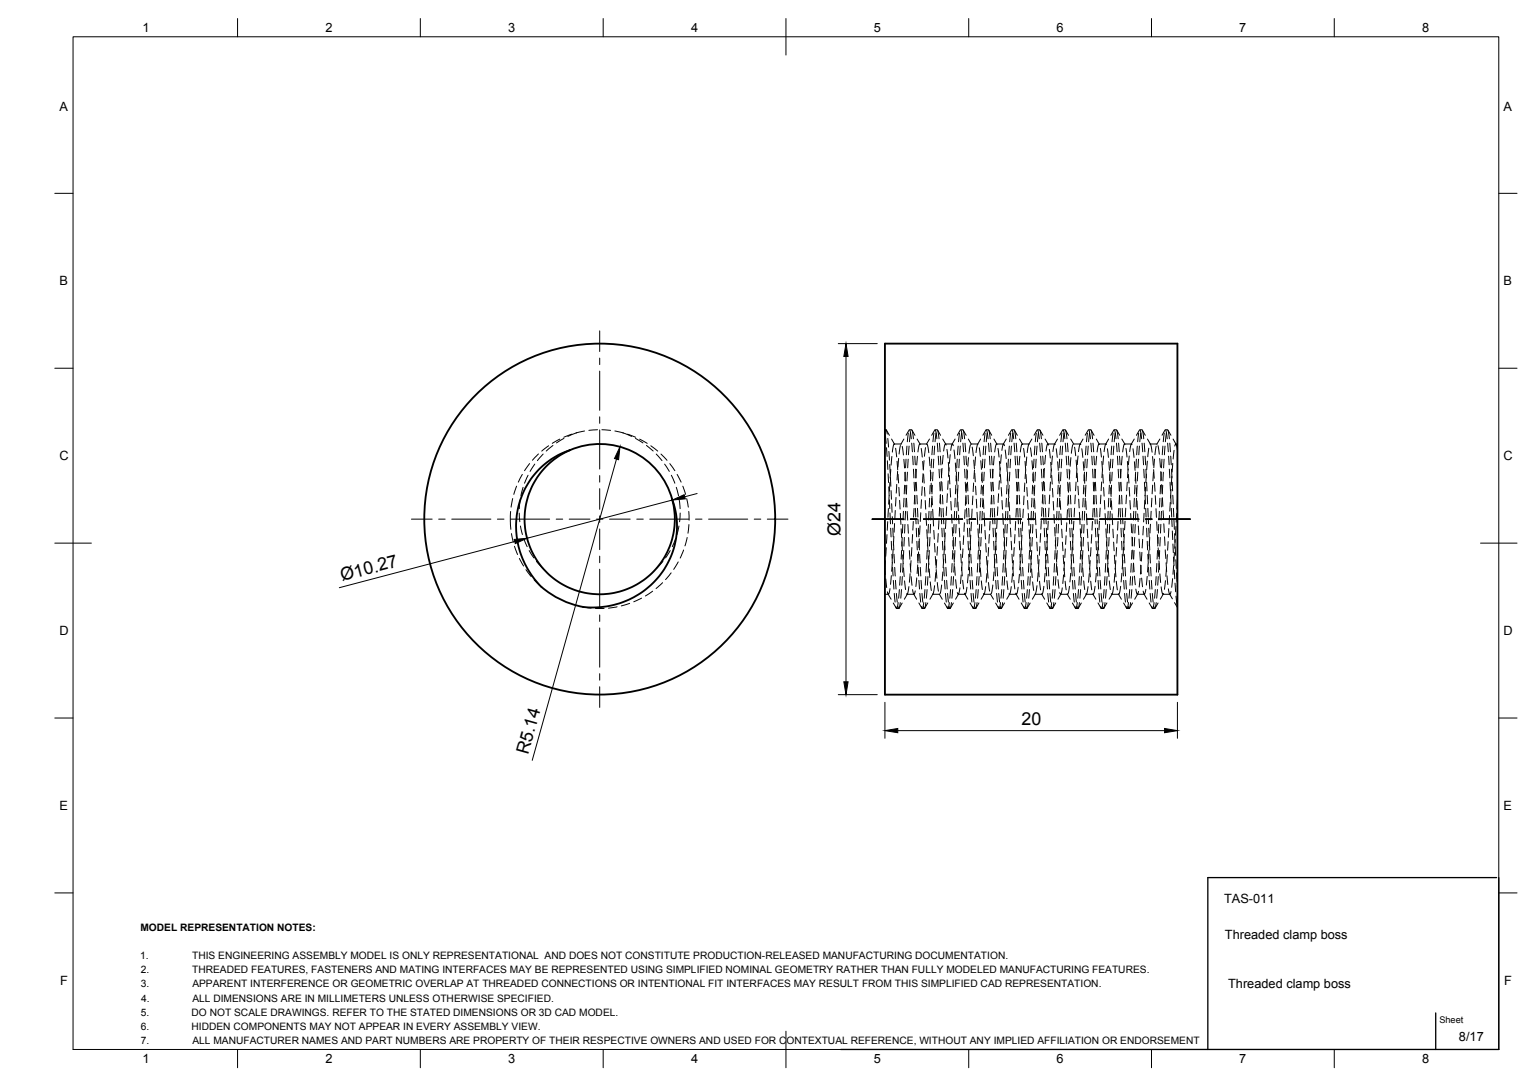
ISO-10303-21;
HEADER;
/* Generated by software containing ST-Developer
 * from STEP Tools, Inc. (www.steptools.com) 
 */

FILE_DESCRIPTION(
/* description */ (
'Independent manual bench leaf bending machine,200mm work width. Fabri
cated welded frame and folding leaf, repeated bushed and fully retaine
d hinge hardware, two handles with bonded grips, beveled clamping beam
 and modeledM12 clamp screws.2mm omitted-workpiece assembly reference 
gap, not a capacity claim. Native135deg hinge travel. Weld sizing, pro
duction fits, material condition, bending capacity, strength and life 
unassigned.'),
/* implementation_level */ '2;1');

FILE_NAME(
/* name */ 'Threaded clamp boss.step',
/* time_stamp */ '2026-11-14T09:11:34-08:00',
/* author */ (''),
/* organization */ (''),
/* preprocessor_version */ 'ST-DEVELOPER v20.2',
/* originating_system */ 'Autodesk Translation Framework v15.17.0.0',
/* authorisation */ '');

FILE_SCHEMA (('AUTOMOTIVE_DESIGN { 1 0 10303 214 3 1 1 }'));
ENDSEC;

DATA;
#10=MECHANICAL_DESIGN_GEOMETRIC_PRESENTATION_REPRESENTATION('',(#452),#37701);
#148=B_SPLINE_SURFACE_WITH_KNOTS('',3,3,((#12501,#12502,#12503,#12504,#12505,
#12506,#12507,#12508,#12509,#12510,#12511,#12512,#12513,#12514,#12515,#12516,
#12517,#12518,#12519,#12520,#12521,#12522,#12523,#12524,#12525,#12526,#12527,
#12528,#12529,#12530,#12531,#12532,#12533,#12534,#12535,#12536,#12537,#12538,
#12539,#12540,#12541,#12542,#12543,#12544,#12545,#12546,#12547,#12548,#12549,
#12550,#12551,#12552,#12553,#12554,#12555,#12556,#12557,#12558,#12559,#12560,
#12561,#12562,#12563,#12564,#12565,#12566,#12567,#12568,#12569,#12570,#12571,
#12572,#12573,#12574,#12575,#12576,#12577,#12578,#12579,#12580,#12581,#12582,
#12583,#12584,#12585,#12586,#12587,#12588,#12589,#12590,#12591,#12592,#12593,
#12594,#12595,#12596,#12597,#12598,#12599,#12600,#12601,#12602,#12603,#12604,
#12605,#12606,#12607,#12608,#12609,#12610,#12611,#12612,#12613,#12614,#12615,
#12616,#12617,#12618,#12619,#12620,#12621,#12622,#12623,#12624,#12625,#12626,
#12627,#12628,#12629,#12630,#12631,#12632,#12633,#12634,#12635,#12636,#12637,
#12638,#12639,#12640,#12641,#12642,#12643,#12644,#12645,#12646,#12647,#12648,
#12649,#12650,#12651),(#12652,#12653,#12654,#12655,#12656,#12657,#12658,
#12659,#12660,#12661,#12662,#12663,#12664,#12665,#12666,#12667,#12668,#12669,
#12670,#12671,#12672,#12673,#12674,#12675,#12676,#12677,#12678,#12679,#12680,
#12681,#12682,#12683,#12684,#12685,#12686,#12687,#12688,#12689,#12690,#12691,
#12692,#12693,#12694,#12695,#12696,#12697,#12698,#12699,#12700,#12701,#12702,
#12703,#12704,#12705,#12706,#12707,#12708,#12709,#12710,#12711,#12712,#12713,
#12714,#12715,#12716,#12717,#12718,#12719,#12720,#12721,#12722,#12723,#12724,
#12725,#12726,#12727,#12728,#12729,#12730,#12731,#12732,#12733,#12734,#12735,
#12736,#12737,#12738,#12739,#12740,#12741,#12742,#12743,#12744,#12745,#12746,
#12747,#12748,#12749,#12750,#12751,#12752,#12753,#12754,#12755,#12756,#12757,
#12758,#12759,#12760,#12761,#12762,#12763,#12764,#12765,#12766,#12767,#12768,
#12769,#12770,#12771,#12772,#12773,#12774,#12775,#12776,#12777,#12778,#12779,
#12780,#12781,#12782,#12783,#12784,#12785,#12786,#12787,#12788,#12789,#12790,
#12791,#12792,#12793,#12794,#12795,#12796,#12797,#12798,#12799,#12800,#12801,
#12802),(#12803,#12804,#12805,#12806,#12807,#12808,#12809,#12810,#12811,
#12812,#12813,#12814,#12815,#12816,#12817,#12818,#12819,#12820,#12821,#12822,
#12823,#12824,#12825,#12826,#12827,#12828,#12829,#12830,#12831,#12832,#12833,
#12834,#12835,#12836,#12837,#12838,#12839,#12840,#12841,#12842,#12843,#12844,
#12845,#12846,#12847,#12848,#12849,#12850,#12851,#12852,#12853,#12854,#12855,
#12856,#12857,#12858,#12859,#12860,#12861,#12862,#12863,#12864,#12865,#12866,
#12867,#12868,#12869,#12870,#12871,#12872,#12873,#12874,#12875,#12876,#12877,
#12878,#12879,#12880,#12881,#12882,#12883,#12884,#12885,#12886,#12887,#12888,
#12889,#12890,#12891,#12892,#12893,#12894,#12895,#12896,#12897,#12898,#12899,
#12900,#12901,#12902,#12903,#12904,#12905,#12906,#12907,#12908,#12909,#12910,
#12911,#12912,#12913,#12914,#12915,#12916,#12917,#12918,#12919,#12920,#12921,
#12922,#12923,#12924,#12925,#12926,#12927,#12928,#12929,#12930,#12931,#12932,
#12933,#12934,#12935,#12936,#12937,#12938,#12939,#12940,#12941,#12942,#12943,
#12944,#12945,#12946,#12947,#12948,#12949,#12950,#12951,#12952,#12953),
(#12954,#12955,#12956,#12957,#12958,#12959,#12960,#12961,#12962,#12963,
#12964,#12965,#12966,#12967,#12968,#12969,#12970,#12971,#12972,#12973,#12974,
#12975,#12976,#12977,#12978,#12979,#12980,#12981,#12982,#12983,#12984,#12985,
#12986,#12987,#12988,#12989,#12990,#12991,#12992,#12993,#12994,#12995,#12996,
#12997,#12998,#12999,#13000,#13001,#13002,#13003,#13004,#13005,#13006,#13007,
#13008,#13009,#13010,#13011,#13012,#13013,#13014,#13015,#13016,#13017,#13018,
#13019,#13020,#13021,#13022,#13023,#13024,#13025,#13026,#13027,#13028,#13029,
#13030,#13031,#13032,#13033,#13034,#13035,#13036,#13037,#13038,#13039,#13040,
#13041,#13042,#13043,#13044,#13045,#13046,#13047,#13048,#13049,#13050,#13051,
#13052,#13053,#13054,#13055,#13056,#13057,#13058,#13059,#13060,#13061,#13062,
#13063,#13064,#13065,#13066,#13067,#13068,#13069,#13070,#13071,#13072,#13073,
#13074,#13075,#13076,#13077,#13078,#13079,#13080,#13081,#13082,#13083,#13084,
#13085,#13086,#13087,#13088,#13089,#13090,#13091,#13092,#13093,#13094,#13095,
#13096,#13097,#13098,#13099,#13100,#13101,#13102,#13103,#13104)),
 .UNSPECIFIED.,.F.,.F.,.F.,(4,4),(4,1,1,1,1,1,1,1,1,1,1,1,1,1,1,1,1,1,1,
1,1,1,1,1,1,1,1,1,1,1,1,1,1,1,1,1,1,1,1,1,1,1,1,1,1,1,1,1,1,1,1,1,1,1,1,
1,1,1,1,1,1,1,1,1,1,1,1,1,1,1,1,1,1,1,1,1,1,1,1,1,1,1,1,1,1,1,1,1,1,1,1,
1,1,1,1,1,1,1,1,1,1,1,1,1,1,1,1,1,1,1,1,1,1,1,1,1,1,1,1,1,1,1,1,1,1,1,1,
1,1,1,1,1,1,1,1,1,1,1,1,1,1,1,1,1,1,1,1,1,4),(-6.2431789936198E-5,0.112802168308183),
(11.8516712330609,12.3505987470977,12.8494638293446,13.3483289115915,13.8471939938383,
14.3460590760852,14.8449241583321,15.343789240579,15.8426543228258,16.3415194050727,
16.8403844873196,17.3392495695665,17.8381146518133,18.3369797340602,18.8358448163071,
19.334709898554,19.8335749808009,20.3324400630477,20.8313051452946,21.3301702275415,
21.8290353097884,22.3279003920352,22.8267654742821,23.325630556529,23.8244956387759,
24.3233607210227,24.8222258032696,25.3210908855165,25.8199559677634,26.3188210500103,
26.8176861322571,27.316551214504,27.8154162967509,28.3142813789978,28.8131464612446,
29.3120115434915,29.8108766257384,30.3097417079853,30.8086067902321,31.307471872479,
31.8063369547259,32.3052020369728,32.8040671192197,33.3029322014665,33.8017972837134,
34.3006623659603,34.7995274482072,35.298392530454,35.7972576127009,36.2961226949478,
36.7949877771947,37.2938528594415,37.7927179416884,38.2915830239353,38.7904481061822,
39.2893131884291,39.7881782706759,40.2870433529228,40.7859084351697,41.2847735174166,
41.7836385996634,42.2825036819103,42.7813687641572,43.2802338464041,43.779098928651,
44.2779640108978,44.7768290931447,45.2756941753916,45.7745592576385,46.2734243398853,
46.7722894221322,47.2711545043791,47.770019586626,48.2688846688728,48.7677497511197,
49.2666148333666,49.7654799156135,50.2643449978603,50.7632100801072,51.2620751623541,
51.760940244601,52.2598053268479,52.7586704090947,53.2575354913416,53.7564005735885,
54.2552656558354,54.7541307380822,55.2529958203291,55.751860902576,56.2507259848229,
56.7495910670697,57.2484561493166,57.7473212315635,58.2461863138104,58.7450513960573,
59.2439164783041,59.742781560551,60.2416466427979,60.7405117250448,61.2393768072916,
61.7382418895385,62.2371069717854,62.7359720540323,63.2348371362792,63.733702218526,
64.2325673007729,64.7314323830198,65.2302974652667,65.7291625475135,66.2280276297604,
66.7268927120073,67.2257577942542,67.724622876501,68.2234879587479,68.7223530409948,
69.2212181232417,69.7200832054885,70.2189482877354,70.7178133699823,71.2166784522292,
71.7155435344761,72.2144086167229,72.7132736989698,73.2121387812167,73.7110038634636,
74.2098689457104,74.7087340279573,75.2075991102042,75.7064641924511,76.205329274698,
76.7041943569448,77.2030594391917,77.7019245214386,78.2007896036855,78.6996546859323,
79.1985197681792,79.6973848504261,80.196249932673,80.6951150149198,81.1939800971667,
81.6928451794136,82.1917102616605,82.6905753439074,83.1894404261542,83.6883055084011,
84.187170590648,84.6860356728949,85.1849007551417,85.6837658373886),
 .UNSPECIFIED.);
#149=B_SPLINE_SURFACE_WITH_KNOTS('',3,3,((#13322,#13323,#13324,#13325,#13326,
#13327,#13328,#13329,#13330,#13331,#13332,#13333,#13334,#13335,#13336,#13337,
#13338,#13339,#13340,#13341,#13342,#13343,#13344,#13345,#13346,#13347,#13348,
#13349,#13350,#13351,#13352,#13353,#13354,#13355,#13356,#13357,#13358,#13359,
#13360,#13361,#13362,#13363,#13364,#13365,#13366,#13367,#13368,#13369,#13370,
#13371,#13372,#13373,#13374,#13375,#13376,#13377,#13378,#13379,#13380,#13381,
#13382,#13383,#13384,#13385,#13386,#13387,#13388,#13389,#13390,#13391,#13392,
#13393,#13394,#13395,#13396,#13397,#13398,#13399,#13400,#13401,#13402,#13403,
#13404,#13405,#13406,#13407,#13408,#13409,#13410,#13411,#13412,#13413,#13414,
#13415,#13416,#13417,#13418,#13419,#13420,#13421,#13422,#13423,#13424,#13425,
#13426,#13427,#13428,#13429,#13430,#13431,#13432,#13433,#13434,#13435,#13436,
#13437,#13438,#13439,#13440,#13441,#13442,#13443,#13444,#13445,#13446,#13447,
#13448,#13449,#13450,#13451,#13452,#13453,#13454,#13455,#13456,#13457,#13458,
#13459,#13460,#13461,#13462,#13463,#13464,#13465,#13466,#13467,#13468,#13469,
#13470,#13471,#13472),(#13473,#13474,#13475,#13476,#13477,#13478,#13479,
#13480,#13481,#13482,#13483,#13484,#13485,#13486,#13487,#13488,#13489,#13490,
#13491,#13492,#13493,#13494,#13495,#13496,#13497,#13498,#13499,#13500,#13501,
#13502,#13503,#13504,#13505,#13506,#13507,#13508,#13509,#13510,#13511,#13512,
#13513,#13514,#13515,#13516,#13517,#13518,#13519,#13520,#13521,#13522,#13523,
#13524,#13525,#13526,#13527,#13528,#13529,#13530,#13531,#13532,#13533,#13534,
#13535,#13536,#13537,#13538,#13539,#13540,#13541,#13542,#13543,#13544,#13545,
#13546,#13547,#13548,#13549,#13550,#13551,#13552,#13553,#13554,#13555,#13556,
#13557,#13558,#13559,#13560,#13561,#13562,#13563,#13564,#13565,#13566,#13567,
#13568,#13569,#13570,#13571,#13572,#13573,#13574,#13575,#13576,#13577,#13578,
#13579,#13580,#13581,#13582,#13583,#13584,#13585,#13586,#13587,#13588,#13589,
#13590,#13591,#13592,#13593,#13594,#13595,#13596,#13597,#13598,#13599,#13600,
#13601,#13602,#13603,#13604,#13605,#13606,#13607,#13608,#13609,#13610,#13611,
#13612,#13613,#13614,#13615,#13616,#13617,#13618,#13619,#13620,#13621,#13622,
#13623),(#13624,#13625,#13626,#13627,#13628,#13629,#13630,#13631,#13632,
#13633,#13634,#13635,#13636,#13637,#13638,#13639,#13640,#13641,#13642,#13643,
#13644,#13645,#13646,#13647,#13648,#13649,#13650,#13651,#13652,#13653,#13654,
#13655,#13656,#13657,#13658,#13659,#13660,#13661,#13662,#13663,#13664,#13665,
#13666,#13667,#13668,#13669,#13670,#13671,#13672,#13673,#13674,#13675,#13676,
#13677,#13678,#13679,#13680,#13681,#13682,#13683,#13684,#13685,#13686,#13687,
#13688,#13689,#13690,#13691,#13692,#13693,#13694,#13695,#13696,#13697,#13698,
#13699,#13700,#13701,#13702,#13703,#13704,#13705,#13706,#13707,#13708,#13709,
#13710,#13711,#13712,#13713,#13714,#13715,#13716,#13717,#13718,#13719,#13720,
#13721,#13722,#13723,#13724,#13725,#13726,#13727,#13728,#13729,#13730,#13731,
#13732,#13733,#13734,#13735,#13736,#13737,#13738,#13739,#13740,#13741,#13742,
#13743,#13744,#13745,#13746,#13747,#13748,#13749,#13750,#13751,#13752,#13753,
#13754,#13755,#13756,#13757,#13758,#13759,#13760,#13761,#13762,#13763,#13764,
#13765,#13766,#13767,#13768,#13769,#13770,#13771,#13772,#13773,#13774),
(#13775,#13776,#13777,#13778,#13779,#13780,#13781,#13782,#13783,#13784,
#13785,#13786,#13787,#13788,#13789,#13790,#13791,#13792,#13793,#13794,#13795,
#13796,#13797,#13798,#13799,#13800,#13801,#13802,#13803,#13804,#13805,#13806,
#13807,#13808,#13809,#13810,#13811,#13812,#13813,#13814,#13815,#13816,#13817,
#13818,#13819,#13820,#13821,#13822,#13823,#13824,#13825,#13826,#13827,#13828,
#13829,#13830,#13831,#13832,#13833,#13834,#13835,#13836,#13837,#13838,#13839,
#13840,#13841,#13842,#13843,#13844,#13845,#13846,#13847,#13848,#13849,#13850,
#13851,#13852,#13853,#13854,#13855,#13856,#13857,#13858,#13859,#13860,#13861,
#13862,#13863,#13864,#13865,#13866,#13867,#13868,#13869,#13870,#13871,#13872,
#13873,#13874,#13875,#13876,#13877,#13878,#13879,#13880,#13881,#13882,#13883,
#13884,#13885,#13886,#13887,#13888,#13889,#13890,#13891,#13892,#13893,#13894,
#13895,#13896,#13897,#13898,#13899,#13900,#13901,#13902,#13903,#13904,#13905,
#13906,#13907,#13908,#13909,#13910,#13911,#13912,#13913,#13914,#13915,#13916,
#13917,#13918,#13919,#13920,#13921,#13922,#13923,#13924,#13925)),
 .UNSPECIFIED.,.F.,.F.,.F.,(4,4),(4,1,1,1,1,1,1,1,1,1,1,1,1,1,1,1,1,1,1,
1,1,1,1,1,1,1,1,1,1,1,1,1,1,1,1,1,1,1,1,1,1,1,1,1,1,1,1,1,1,1,1,1,1,1,1,
1,1,1,1,1,1,1,1,1,1,1,1,1,1,1,1,1,1,1,1,1,1,1,1,1,1,1,1,1,1,1,1,1,1,1,1,
1,1,1,1,1,1,1,1,1,1,1,1,1,1,1,1,1,1,1,1,1,1,1,1,1,1,1,1,1,1,1,1,1,1,1,1,
1,1,1,1,1,1,1,1,1,1,1,1,1,1,1,1,1,1,1,1,1,4),(-4.55374339698837E-5,0.1128189478572),
(14.3984001269718,14.8972652092187,15.3961302914656,15.8949953737124,16.3938604559593,
16.8927255382062,17.3915906204531,17.8904557026999,18.3893207849468,18.8881858671937,
19.3870509494406,19.8859160316874,20.3847811139343,20.8836461961812,21.3825112784281,
21.881376360675,22.3802414429218,22.8791065251687,23.3779716074156,23.8768366896625,
24.3757017719093,24.8745668541562,25.3734319364031,25.87229701865,26.3711621008968,
26.8700271831437,27.3688922653906,27.8677573476375,28.3666224298844,28.8654875121312,
29.3643525943781,29.863217676625,30.3620827588719,30.8609478411187,31.3598129233656,
31.8586780056125,32.3575430878594,32.8564081701062,33.3552732523531,33.8541383346,
34.3530034168469,34.8518684990938,35.3507335813406,35.8495986635875,36.3484637458344,
36.8473288280813,37.3461939103281,37.845058992575,38.3439240748219,38.8427891570688,
39.3416542393157,39.8405193215625,40.3393844038094,40.8382494860563,41.3371145683032,
41.83597965055,42.3348447327969,42.8337098150438,43.3325748972907,43.8314399795375,
44.3303050617844,44.8291701440313,45.3280352262782,45.8269003085251,46.3257653907719,
46.8246304730188,47.3234955552657,47.8223606375126,48.3212257197594,48.8200908020063,
49.3189558842532,49.8178209665001,50.316686048747,50.8155511309938,51.3144162132407,
51.8132812954876,52.3121463777345,52.8110114599813,53.3098765422282,53.8087416244751,
54.307606706722,54.8064717889688,55.3053368712157,55.8042019534626,56.3030670357095,
56.8019321179564,57.3007972002032,57.7996622824501,58.298527364697,58.7973924469439,
59.2962575291907,59.7951226114376,60.2939876936845,60.7928527759314,61.2917178581782,
61.7905829404251,62.289448022672,62.7883131049189,63.2871781871658,63.7860432694126,
64.2849083516595,64.7837734339064,65.2826385161533,65.7815035984001,66.280368680647,
66.7792337628939,67.2780988451408,67.7769639273876,68.2758290096345,68.7746940918814,
69.2735591741283,69.7724242563752,70.271289338622,70.7701544208689,71.2690195031158,
71.7678845853627,72.2667496676095,72.7656147498564,73.2644798321033,73.7633449143502,
74.2622099965971,74.7610750788439,75.2599401610908,75.7588052433377,76.2576703255846,
76.7565354078314,77.2554004900783,77.7542655723252,78.2531306545721,78.7519957368189,
79.2508608190658,79.7497259013127,80.2485909835596,80.7474560658064,81.2463211480533,
81.7451862303002,82.2440513125471,82.742916394794,83.2417814770408,83.7406465592877,
84.2395116415346,84.7383767237815,85.2372418060283,85.7361068882752,86.2349719705221,
86.733837052769,87.2327021350158,87.7315672172627,88.2304947397941),
 .UNSPECIFIED.);
#152=B_SPLINE_CURVE_WITH_KNOTS('',3,(#5917,#5918,#5919,#5920,#5921,#5922,
#5923,#5924,#5925,#5926,#5927,#5928),.UNSPECIFIED.,.F.,.F.,(4,1,1,1,1,1,
1,1,1,4),(80.7654236598523,81.1939800971667,81.6928451794136,82.1917102616605,
82.6905753439074,83.1894404261542,83.6883055084011,84.187170590648,84.6860356728949,
84.8230016469244),.UNSPECIFIED.);
#153=B_SPLINE_CURVE_WITH_KNOTS('',3,(#5930,#5931,#5932,#5933,#5934),
 .UNSPECIFIED.,.F.,.F.,(4,1,4),(84.8230016469244,85.1849007551417,85.6837658373886),
 .UNSPECIFIED.);
#154=B_SPLINE_CURVE_WITH_KNOTS('',3,(#5938,#5939,#5940,#5941,#5942,#5943,
#5944,#5945,#5946,#5947,#5948,#5949,#5950,#5951,#5952,#5953,#5954,#5955,
#5956,#5957,#5958,#5959,#5960,#5961,#5962,#5963,#5964,#5965,#5966,#5967,
#5968,#5969,#5970,#5971,#5972,#5973,#5974,#5975,#5976,#5977,#5978,#5979,
#5980,#5981,#5982,#5983,#5984,#5985,#5986,#5987,#5988,#5989),
 .UNSPECIFIED.,.F.,.F.,(4,3,3,3,3,3,3,3,3,3,3,3,3,3,3,3,3,4),(84.8230016469244,
84.9058580301686,84.9887137387844,85.0715624591206,85.1544337152411,85.2372418060283,
85.3204458619835,85.4036336567022,85.4868246260799,85.5700099876162,85.6532174303604,
85.7361068882752,85.8191359181166,85.9021481942019,85.9851620989545,86.0681715464416,
86.151200160365,86.2062322090242),.UNSPECIFIED.);
#155=B_SPLINE_CURVE_WITH_KNOTS('',3,(#5990,#5991,#5992,#5993,#5994,#5995,
#5996,#5997,#5998,#5999,#6000,#6001),.UNSPECIFIED.,.F.,.F.,(4,1,1,1,1,1,
1,1,1,4),(80.7654089732259,81.2463211480533,81.7451862303002,82.2440513125471,
82.742916394794,83.2417814770408,83.7406465592877,84.2395116415346,84.7383767237815,
84.8230016469244),.UNSPECIFIED.);
#156=B_SPLINE_CURVE_WITH_KNOTS('',3,(#6007,#6008,#6009,#6010,#6011,#6012,
#6013,#6014,#6015,#6016,#6017,#6018,#6019,#6020,#6021,#6022,#6023,#6024,
#6025,#6026,#6027,#6028,#6029,#6030,#6031,#6032,#6033,#6034,#6035,#6036,
#6037,#6038,#6039,#6040,#6041,#6042,#6043,#6044,#6045,#6046,#6047,#6048,
#6049,#6050,#6051,#6052,#6053,#6054,#6055,#6056,#6057,#6058,#6059,#6060,
#6061,#6062,#6063,#6064,#6065,#6066,#6067,#6068,#6069,#6070,#6071,#6072,
#6073,#6074,#6075,#6076,#6077,#6078,#6079,#6080,#6081,#6082,#6083,#6084,
#6085,#6086,#6087,#6088,#6089,#6090,#6091,#6092,#6093,#6094,#6095,#6096,
#6097,#6098,#6099,#6100,#6101,#6102,#6103,#6104,#6105,#6106,#6107,#6108,
#6109,#6110,#6111,#6112,#6113,#6114,#6115,#6116,#6117,#6118,#6119,#6120,
#6121,#6122,#6123,#6124,#6125,#6126,#6127,#6128,#6129,#6130,#6131,#6132,
#6133,#6134,#6135,#6136,#6137,#6138,#6139,#6140,#6141,#6142,#6143,#6144,
#6145,#6146,#6147,#6148,#6149,#6150,#6151,#6152,#6153,#6154),
 .UNSPECIFIED.,.F.,.F.,(4,3,3,3,3,3,3,3,3,3,3,3,3,3,3,3,3,3,3,3,3,3,3,3,
3,3,3,3,3,3,3,3,3,3,3,3,3,3,3,3,3,3,3,3,3,3,3,3,3,4),(74.4822133280158,
74.5653991646366,74.6486051631925,74.7087340279573,74.7919387913187,74.8751273240303,
74.9583190715775,75.0415052315879,75.1247134988495,75.2075991102042,75.2908038725438,
75.3739924042304,75.4571841507579,75.5403703097531,75.6235785760172,75.7064641924511,
75.789668956311,75.8728574895209,75.9560492375621,76.039235398063,76.1224436658041,
76.205329274698,76.2885340372514,76.3717225691568,76.454914315908,76.5381004751292,
76.6213087416209,76.7041943569448,76.7873991181458,76.8705876486823,76.9537793940503,
77.0369655518835,77.1201738169931,77.2030594391917,77.2862642100853,77.3694527503662,
77.452644505469,77.5358306730124,77.619038947697,77.7019245214386,77.7851292641372,
77.8683177761065,77.9515095029856,78.034695642409,78.1179038894172,78.2007896036855,
78.2855462877003,78.3686837869672,78.454250063356,78.5398163397448),
 .UNSPECIFIED.);
#157=B_SPLINE_CURVE_WITH_KNOTS('',3,(#6155,#6156,#6157,#6158,#6159,#6160,
#6161,#6162,#6163),.UNSPECIFIED.,.F.,.F.,(4,1,1,1,1,1,4),(78.5398163723456,
78.6996546859323,79.1985197681792,79.6973848504261,80.196249932673,80.6951150149198,
80.7654236598523),.UNSPECIFIED.);
#158=B_SPLINE_CURVE_WITH_KNOTS('',3,(#6165,#6166,#6167,#6168,#6169,#6170,
#6171,#6172,#6173),.UNSPECIFIED.,.F.,.F.,(4,1,1,1,1,1,4),(78.5398163397448,
78.7519957368189,79.2508608190658,79.7497259013127,80.2485909835596,80.7474560658064,
80.7654089732259),.UNSPECIFIED.);
#159=B_SPLINE_CURVE_WITH_KNOTS('',3,(#6174,#6175,#6176,#6177,#6178,#6179,
#6180,#6181,#6182,#6183,#6184,#6185),.UNSPECIFIED.,.F.,.F.,(4,1,1,1,1,1,
1,1,1,4),(74.4822262911247,74.7610750788439,75.2599401610908,75.7588052433377,
76.2576703255846,76.7565354078314,77.2554004900783,77.7542655723252,78.2531306545721,
78.5398163397448),.UNSPECIFIED.);
#160=B_SPLINE_CURVE_WITH_KNOTS('',3,(#6191,#6192,#6193,#6194,#6195,#6196,
#6197,#6198,#6199,#6200,#6201,#6202,#6203,#6204,#6205,#6206,#6207,#6208,
#6209,#6210,#6211,#6212,#6213,#6214,#6215,#6216,#6217,#6218,#6219,#6220,
#6221,#6222,#6223,#6224,#6225,#6226,#6227,#6228,#6229,#6230,#6231,#6232,
#6233,#6234,#6235,#6236,#6237,#6238,#6239,#6240,#6241,#6242,#6243,#6244,
#6245,#6246,#6247,#6248,#6249,#6250,#6251,#6252,#6253,#6254,#6255,#6256,
#6257,#6258,#6259,#6260,#6261,#6262,#6263,#6264,#6265,#6266,#6267,#6268,
#6269,#6270,#6271,#6272,#6273,#6274,#6275,#6276,#6277,#6278,#6279,#6280,
#6281,#6282,#6283,#6284,#6285,#6286,#6287,#6288,#6289,#6290,#6291,#6292,
#6293,#6294,#6295,#6296,#6297,#6298,#6299,#6300,#6301,#6302,#6303,#6304,
#6305,#6306,#6307,#6308,#6309,#6310,#6311,#6312,#6313,#6314,#6315,#6316,
#6317,#6318,#6319,#6320,#6321,#6322,#6323,#6324,#6325,#6326,#6327,#6328,
#6329,#6330,#6331,#6332,#6333,#6334,#6335,#6336,#6337,#6338,#6339,#6340,
#6341),.UNSPECIFIED.,.F.,.F.,(4,3,3,3,3,3,3,3,3,3,3,3,3,3,3,3,3,3,3,3,3,
3,3,3,3,3,3,3,3,3,3,3,3,3,3,3,3,3,3,3,3,3,3,3,3,3,3,3,3,3,4),(68.1990246102961,
68.2234879587479,68.3066927217448,68.3898812540909,68.473073001274,68.5562591609217,
68.6394674278267,68.7223530409948,68.805557803992,68.8887463363385,68.9719380835218,
69.0551242431698,69.1383325100748,69.2212181232417,69.3044228862387,69.3876114185846,
69.4708031657675,69.5539893254153,69.6371975923201,69.7200832054885,69.8032879684856,
69.8864765008317,69.969668248015,70.052854407663,70.136062674568,70.2189482877354,
70.3021530507327,70.3853415830785,70.4685333302618,70.5517194899096,70.6349277568148,
70.7178133699823,70.8010181329782,70.8842066653234,70.9673984125055,71.0505845721522,
71.1337928390561,71.2166784522292,71.2998832152294,71.3830717475779,71.4662634947639,
71.5494496544144,71.6326579213223,71.7155435344761,71.7987482974668,71.8819368298066,
71.9651285769834,72.0483147366248,72.1315230035237,72.2144086167229,72.2566310325652),
 .UNSPECIFIED.);
#161=B_SPLINE_CURVE_WITH_KNOTS('',3,(#6342,#6343,#6344,#6345,#6346,#6347,
#6348,#6349,#6350,#6351,#6352,#6353,#6354,#6355,#6356,#6357,#6358,#6359,
#6360,#6361,#6362,#6363,#6364,#6365,#6366,#6367,#6368,#6369,#6370,#6371,
#6372,#6373,#6374,#6375,#6376,#6377,#6378,#6379,#6380,#6381,#6382,#6383,
#6384,#6385,#6386,#6387,#6388,#6389,#6390,#6391,#6392,#6393,#6394,#6395,
#6396,#6397,#6398,#6399,#6400,#6401,#6402,#6403,#6404,#6405,#6406,#6407,
#6408,#6409,#6410,#6411,#6412,#6413,#6414,#6415,#6416,#6417,#6418,#6419,
#6420,#6421,#6422,#6423,#6424,#6425,#6426),.UNSPECIFIED.,.F.,.F.,(4,3,3,
3,3,3,3,3,3,3,3,3,3,3,3,3,3,3,3,3,3,3,3,3,3,3,3,3,4),(72.2566310327204,
72.3395787750688,72.4225108202044,72.5054456631146,72.5883776325168,72.6713290333548,
72.7132736989698,72.7964784619549,72.8796669942889,72.9628587414601,73.046044901096,
73.1292531679893,73.2121387812167,73.2953435442142,73.3785320765606,73.4617238237443,
73.5449099833926,73.6281182502978,73.7110038634636,73.7942086265049,73.8773971588956,
73.9605889061234,74.0437750658158,74.1269833327648,74.2098689457104,74.2930744028643,
74.3762623723983,74.4594439181691,74.4822133280158),.UNSPECIFIED.);
#162=B_SPLINE_CURVE_WITH_KNOTS('',3,(#6428,#6429,#6430,#6431,#6432,#6433,
#6434,#6435,#6436),.UNSPECIFIED.,.F.,.F.,(4,1,1,1,1,1,4),(72.2566310325652,
72.2667496676095,72.7656147498564,73.2644798321033,73.7633449143502,74.2622099965971,
74.4822262911247),.UNSPECIFIED.);
#163=B_SPLINE_CURVE_WITH_KNOTS('',3,(#6437,#6438,#6439,#6440,#6441,#6442,
#6443,#6444,#6445,#6446,#6447,#6448,#6449,#6450,#6451,#6452,#6453,#6454,
#6455,#6456,#6457,#6458,#6459,#6460,#6461,#6462,#6463,#6464,#6465,#6466,
#6467,#6468,#6469,#6470,#6471,#6472,#6473,#6474,#6475,#6476,#6477,#6478,
#6479,#6480,#6481,#6482,#6483,#6484,#6485,#6486,#6487,#6488,#6489,#6490,
#6491,#6492,#6493,#6494,#6495,#6496,#6497,#6498,#6499,#6500,#6501,#6502,
#6503,#6504,#6505,#6506,#6507,#6508,#6509,#6510,#6511,#6512,#6513,#6514,
#6515,#6516,#6517,#6518,#6519,#6520,#6521,#6522,#6523,#6524,#6525,#6526,
#6527,#6528,#6529,#6530,#6531,#6532,#6533,#6534,#6535,#6536,#6537,#6538,
#6539,#6540,#6541,#6542,#6543,#6544,#6545,#6546,#6547,#6548,#6549,#6550,
#6551,#6552,#6553,#6554,#6555,#6556,#6557,#6558,#6559,#6560,#6561,#6562,
#6563,#6564,#6565,#6566,#6567,#6568,#6569,#6570,#6571,#6572,#6573,#6574,
#6575,#6576,#6577,#6578,#6579,#6580,#6581,#6582,#6583,#6584),
 .UNSPECIFIED.,.F.,.F.,(4,3,3,3,3,3,3,3,3,3,3,3,3,3,3,3,3,3,3,3,3,3,3,3,
3,3,3,3,3,3,3,3,3,3,3,3,3,3,3,3,3,3,3,3,3,3,3,3,3,4),(68.1990161073015,
68.2758290096345,68.3590337726316,68.4422223049775,68.5254140521607,68.6086002118086,
68.6918084787137,68.7746940918814,68.8578988548785,68.9410873872244,69.0242791344076,
69.1074652940555,69.1906735609605,69.2735591741283,69.3567639371251,69.4399524694712,
69.5231442166544,69.6063303763024,69.6895386432074,69.7724242563752,69.8556290193721,
69.9388175517181,70.0220092989012,70.1051954585491,70.1884037254542,70.271289338622,
70.3544941016189,70.4376826339646,70.5208743811479,70.6040605407956,70.6872688077007,
70.7701544208689,70.8533591838659,70.9365477162118,71.0197394633952,71.1029256230433,
71.1861338899484,71.2690195031158,71.352224266113,71.4354127984596,71.5186045456429,
71.6017907052906,71.6849989721958,71.7678845853627,71.8510125628734,71.9341240557072,
72.0172382375382,72.1003472864947,72.1834776083169,72.2566310325652),
 .UNSPECIFIED.);
#164=B_SPLINE_CURVE_WITH_KNOTS('',3,(#6590,#6591,#6592,#6593,#6594,#6595,
#6596,#6597,#6598,#6599,#6600,#6601),.UNSPECIFIED.,.F.,.F.,(4,1,1,1,1,1,
1,1,1,4),(61.9158664354373,62.2371069717854,62.7359720540323,63.2348371362792,
63.733702218526,64.2325673007729,64.7314323830198,65.2302974652667,65.7291625475135,
65.9734457216197),.UNSPECIFIED.);
#165=B_SPLINE_CURVE_WITH_KNOTS('',3,(#6602,#6603,#6604,#6605,#6606,#6607,
#6608,#6609,#6610,#6611,#6612,#6613,#6614,#6615,#6616,#6617,#6618,#6619,
#6620,#6621,#6622,#6623,#6624,#6625,#6626,#6627,#6628,#6629,#6630,#6631,
#6632,#6633,#6634,#6635,#6636,#6637,#6638,#6639,#6640,#6641,#6642,#6643,
#6644,#6645,#6646,#6647,#6648,#6649,#6650,#6651,#6652,#6653,#6654,#6655,
#6656,#6657,#6658,#6659,#6660,#6661,#6662,#6663,#6664,#6665,#6666,#6667,
#6668,#6669,#6670,#6671,#6672,#6673,#6674,#6675,#6676,#6677,#6678,#6679,
#6680,#6681,#6682,#6683),.UNSPECIFIED.,.F.,.F.,(4,3,3,3,3,3,3,3,3,3,3,3,
3,3,3,3,3,3,3,3,3,3,3,3,3,3,3,4),(65.9734457253856,66.0575770114745,66.1428023206174,
66.2280276297604,66.3112323927575,66.3944209251034,66.4776126722867,66.5607988319345,
66.6440070988396,66.7268927120073,66.8100974750044,66.8932860073503,66.9764777545334,
67.0596639141813,67.1428721810863,67.2257577942542,67.3089625572514,67.3921510895973,
67.4753428367804,67.5585289964282,67.6417372633332,67.724622876501,67.8078273552862,
67.8910155036496,67.974204708283,68.0573885356163,68.1405895310058,68.1990246102961),
 .UNSPECIFIED.);
#166=B_SPLINE_CURVE_WITH_KNOTS('',3,(#6685,#6686,#6687,#6688,#6689,#6690,
#6691,#6692,#6693,#6694,#6695,#6696,#6697,#6698,#6699,#6700,#6701,#6702,
#6703,#6704,#6705,#6706,#6707,#6708,#6709,#6710,#6711,#6712,#6713,#6714,
#6715,#6716,#6717,#6718,#6719,#6720,#6721,#6722,#6723,#6724,#6725,#6726,
#6727,#6728,#6729,#6730,#6731,#6732,#6733,#6734,#6735,#6736,#6737,#6738,
#6739,#6740,#6741,#6742,#6743,#6744,#6745,#6746,#6747,#6748,#6749,#6750,
#6751,#6752,#6753,#6754,#6755,#6756,#6757,#6758,#6759,#6760,#6761,#6762,
#6763,#6764,#6765,#6766),.UNSPECIFIED.,.F.,.F.,(4,3,3,3,3,3,3,3,3,3,3,3,
3,3,3,3,3,3,3,3,3,3,3,3,3,3,3,4),(65.9734457253856,66.0568706822057,66.1402945367021,
66.2237400485274,66.280368680647,66.3635734436441,66.4467619759899,66.529953723173,
66.6131398828208,66.6963481497259,66.7792337628939,66.8624385258909,66.945627058237,
67.0288188054201,67.1120049650679,67.1952132319729,67.2780988451408,67.3613036081377,
67.4444921404837,67.5276838876669,67.6108700473146,67.6940783142196,67.7769639273876,
67.8601680001445,67.9448800269338,68.0280644468231,68.1135402770623,68.1990161073015),
 .UNSPECIFIED.);
#167=B_SPLINE_CURVE_WITH_KNOTS('',3,(#6767,#6768,#6769,#6770,#6771,#6772,
#6773,#6774,#6775,#6776,#6777,#6778),.UNSPECIFIED.,.F.,.F.,(4,1,1,1,1,1,
1,1,1,4),(61.9158726512869,62.289448022672,62.7883131049189,63.2871781871658,
63.7860432694126,64.2849083516595,64.7837734339064,65.2826385161533,65.7815035984001,
65.9734456901994),.UNSPECIFIED.);
#168=B_SPLINE_CURVE_WITH_KNOTS('',3,(#6784,#6785,#6786,#6787,#6788,#6789,
#6790,#6791,#6792,#6793,#6794,#6795,#6796,#6797,#6798,#6799,#6800,#6801,
#6802,#6803,#6804,#6805,#6806,#6807,#6808,#6809,#6810,#6811,#6812,#6813,
#6814,#6815,#6816,#6817,#6818,#6819,#6820,#6821,#6822,#6823,#6824,#6825,
#6826,#6827,#6828,#6829,#6830,#6831,#6832,#6833,#6834,#6835,#6836,#6837,
#6838,#6839,#6840,#6841,#6842,#6843,#6844,#6845,#6846,#6847,#6848,#6849,
#6850,#6851,#6852,#6853,#6854,#6855,#6856,#6857,#6858,#6859,#6860,#6861,
#6862,#6863,#6864,#6865,#6866,#6867,#6868,#6869,#6870,#6871,#6872,#6873,
#6874,#6875,#6876,#6877,#6878,#6879,#6880,#6881,#6882,#6883,#6884,#6885,
#6886,#6887,#6888,#6889,#6890,#6891,#6892,#6893,#6894,#6895,#6896,#6897,
#6898,#6899,#6900,#6901,#6902,#6903,#6904,#6905,#6906,#6907,#6908,#6909,
#6910,#6911,#6912,#6913,#6914,#6915,#6916,#6917,#6918,#6919,#6920,#6921,
#6922,#6923,#6924,#6925,#6926,#6927,#6928,#6929,#6930,#6931,#6932,#6933,
#6934),.UNSPECIFIED.,.F.,.F.,(4,3,3,3,3,3,3,3,3,3,3,3,3,3,3,3,3,3,3,3,3,
3,3,3,3,3,3,3,3,3,3,3,3,3,3,3,3,3,3,3,3,3,3,3,3,3,3,3,3,3,4),(55.6326446456766,
55.7158491503551,55.751860902576,55.835065665573,55.9182541979186,56.0014459451018,
56.0846321047497,56.1678403716548,56.2507259848229,56.3339307478201,56.4171192801657,
56.5003110273488,56.5834971869966,56.6667054539017,56.7495910670697,56.8327958300666,
56.9159843624127,56.9991761095957,57.0823622692435,57.1655705361485,57.2484561493166,
57.3316609123136,57.4148494446596,57.4980411918429,57.5812273514908,57.6644356183958,
57.7473212315635,57.8305259945606,57.9137145269063,57.9969062740895,58.0800924337372,
58.1633007006423,58.2461863138104,58.3293910768073,58.4125796091535,58.4957713563367,
58.5789575159845,58.6621657828895,58.7450513960573,58.8282561590543,58.9114446914002,
58.9946364385832,59.0778225982313,59.1610308651363,59.2439164783041,59.3268318318306,
59.4097299979322,59.4926282254384,59.5755226544865,59.6584334114035,59.690260418206),
 .UNSPECIFIED.);
#169=B_SPLINE_CURVE_WITH_KNOTS('',3,(#6935,#6936,#6937,#6938,#6939,#6940,
#6941,#6942,#6943),.UNSPECIFIED.,.F.,.F.,(4,1,1,1,1,1,4),(59.690260418206,
59.742781560551,60.2416466427979,60.7405117250448,61.2393768072916,61.7382418895385,
61.9158664354373),.UNSPECIFIED.);
#170=B_SPLINE_CURVE_WITH_KNOTS('',3,(#6945,#6946,#6947,#6948,#6949,#6950,
#6951,#6952,#6953),.UNSPECIFIED.,.F.,.F.,(4,1,1,1,1,1,4),(59.690260418206,
59.7951226114376,60.2939876936845,60.7928527759314,61.2917178581782,61.7905829404251,
61.9158726512869),.UNSPECIFIED.);
#171=B_SPLINE_CURVE_WITH_KNOTS('',3,(#6954,#6955,#6956,#6957,#6958,#6959,
#6960,#6961,#6962,#6963,#6964,#6965,#6966,#6967,#6968,#6969,#6970,#6971,
#6972,#6973,#6974,#6975,#6976,#6977,#6978,#6979,#6980,#6981,#6982,#6983,
#6984,#6985,#6986,#6987,#6988,#6989,#6990,#6991,#6992,#6993,#6994,#6995,
#6996,#6997,#6998,#6999,#7000,#7001,#7002,#7003,#7004,#7005,#7006,#7007,
#7008,#7009,#7010,#7011,#7012,#7013,#7014,#7015,#7016,#7017,#7018,#7019,
#7020,#7021,#7022,#7023,#7024,#7025,#7026,#7027,#7028,#7029,#7030,#7031,
#7032,#7033,#7034,#7035,#7036,#7037,#7038,#7039,#7040,#7041,#7042,#7043,
#7044,#7045,#7046,#7047,#7048,#7049,#7050,#7051,#7052,#7053,#7054,#7055,
#7056,#7057,#7058,#7059,#7060,#7061,#7062,#7063,#7064,#7065,#7066,#7067,
#7068,#7069,#7070,#7071,#7072,#7073,#7074,#7075,#7076,#7077,#7078,#7079,
#7080,#7081,#7082,#7083,#7084,#7085,#7086,#7087,#7088,#7089,#7090,#7091,
#7092,#7093,#7094,#7095,#7096,#7097,#7098,#7099,#7100,#7101),
 .UNSPECIFIED.,.F.,.F.,(4,3,3,3,3,3,3,3,3,3,3,3,3,3,3,3,3,3,3,3,3,3,3,3,
3,3,3,3,3,3,3,3,3,3,3,3,3,3,3,3,3,3,3,3,3,3,3,3,3,4),(55.6326489767496,
55.7184254651061,55.8042019534626,55.8874067164596,55.970595248806,56.0537869959891,
56.136973155637,56.220181422542,56.3030670357095,56.3862717987066,56.4694603310523,
56.5526520782354,56.6358382378835,56.7190465047884,56.8019321179564,56.8851368809535,
56.9683254132997,57.0515171604829,57.1347033201307,57.2179115870357,57.3007972002032,
57.3840019632003,57.4671904955464,57.5503822427296,57.6335684023773,57.7167766692823,
57.7996622824501,57.8828670454471,57.9660555777933,58.0492473249765,58.1324334846246,
58.2156417515297,58.298527364697,58.3817321276939,58.4649206600397,58.5481124072229,
58.6312985668706,58.7145068337754,58.7973924469439,58.880597209941,58.9637857422865,
59.0469774894696,59.1301636491172,59.2133719160221,59.2962575291907,59.3791492032558,
59.4620306976914,59.5449010195121,59.627782428294,59.690260418206),
 .UNSPECIFIED.);
#172=B_SPLINE_CURVE_WITH_KNOTS('',3,(#7107,#7108,#7109,#7110,#7111,#7112,
#7113,#7114,#7115,#7116,#7117,#7118,#7119,#7120,#7121,#7122,#7123,#7124,
#7125,#7126,#7127,#7128,#7129,#7130,#7131,#7132,#7133,#7134,#7135,#7136,
#7137,#7138,#7139,#7140,#7141,#7142,#7143,#7144,#7145,#7146,#7147,#7148,
#7149,#7150,#7151,#7152,#7153,#7154,#7155,#7156,#7157,#7158,#7159,#7160,
#7161,#7162,#7163,#7164,#7165,#7166,#7167,#7168,#7169,#7170,#7171,#7172,
#7173,#7174,#7175,#7176,#7177,#7178,#7179,#7180,#7181,#7182,#7183,#7184,
#7185,#7186,#7187,#7188,#7189,#7190,#7191,#7192,#7193,#7194,#7195,#7196,
#7197,#7198,#7199,#7200,#7201,#7202,#7203,#7204,#7205,#7206,#7207,#7208,
#7209,#7210,#7211,#7212,#7213,#7214,#7215,#7216,#7217,#7218,#7219,#7220,
#7221,#7222,#7223,#7224,#7225,#7226,#7227,#7228,#7229,#7230,#7231,#7232,
#7233,#7234,#7235,#7236,#7237,#7238,#7239,#7240,#7241,#7242,#7243,#7244,
#7245,#7246,#7247,#7248,#7249,#7250,#7251,#7252,#7253,#7254),
 .UNSPECIFIED.,.F.,.F.,(4,3,3,3,3,3,3,3,3,3,3,3,3,3,3,3,3,3,3,3,3,3,3,3,
3,3,3,3,3,3,3,3,3,3,3,3,3,3,3,3,3,3,3,3,3,3,3,3,3,4),(49.3494924806201,
49.4326810632531,49.5158807763432,49.5990669442003,49.6822752488321,49.7654799156135,
49.8486846786105,49.9318732109565,50.0150649581396,50.0982511177874,50.1814593846924,
50.2643449978603,50.3475497608573,50.4307382932033,50.5139300403864,50.5971162000342,
50.6803244669392,50.7632100801072,50.8464148431043,50.9296033754502,51.0127951226334,
51.0959812822813,51.1791895491863,51.2620751623541,51.3452799253512,51.4284684576972,
51.5116602048803,51.5948463645282,51.6780546314332,51.760940244601,51.844145007598,
51.9273335399439,52.0105252871271,52.0937114467749,52.1769197136799,52.2598053268479,
52.343010089845,52.4261986221908,52.509390369374,52.5925765290218,52.6757847959268,
52.7586704090947,52.8418751720917,52.9250637044375,53.0082554516206,53.0914416112682,
53.1746498781732,53.2575354913416,53.3441594282935,53.4070751109103),
 .UNSPECIFIED.);
#173=B_SPLINE_CURVE_WITH_KNOTS('',3,(#7255,#7256,#7257,#7258,#7259,#7260,
#7261,#7262,#7263,#7264,#7265,#7266,#7267,#7268,#7269,#7270,#7271,#7272,
#7273,#7274,#7275,#7276,#7277,#7278,#7279,#7280,#7281,#7282,#7283,#7284,
#7285,#7286,#7287,#7288,#7289,#7290,#7291,#7292,#7293,#7294,#7295,#7296,
#7297,#7298,#7299,#7300,#7301,#7302,#7303,#7304,#7305,#7306,#7307,#7308,
#7309,#7310,#7311,#7312,#7313,#7314,#7315,#7316,#7317,#7318,#7319,#7320,
#7321,#7322,#7323,#7324,#7325,#7326,#7327,#7328,#7329,#7330,#7331,#7332,
#7333,#7334,#7335,#7336,#7337,#7338,#7339),.UNSPECIFIED.,.F.,.F.,(4,3,3,
3,3,3,3,3,3,3,3,3,3,3,3,3,3,3,3,3,3,3,3,3,3,3,3,3,4),(53.4070751110264,
53.4944064766669,53.577468684068,53.6605312927296,53.7436119100014,53.7564005735885,
53.8396053365855,53.9227938689313,54.0059856161145,54.0891717757623,54.1723800426672,
54.2552656558354,54.3384704188324,54.4216589511783,54.5048506983614,54.5880368580093,
54.6712451249142,54.7541307380822,54.8373355010792,54.920524033425,55.0037157806081,
55.0869019402558,55.1701102071608,55.2529958203291,55.3361997661843,55.419392877731,
55.5025745053791,55.5857617771024,55.6326446456766),.UNSPECIFIED.);
#174=B_SPLINE_CURVE_WITH_KNOTS('',3,(#7341,#7342,#7343,#7344,#7345,#7346,
#7347,#7348,#7349,#7350,#7351,#7352,#7353,#7354,#7355,#7356,#7357,#7358,
#7359,#7360,#7361,#7362,#7363,#7364,#7365,#7366,#7367,#7368,#7369,#7370,
#7371,#7372,#7373,#7374,#7375,#7376,#7377,#7378,#7379,#7380,#7381,#7382,
#7383,#7384,#7385,#7386,#7387,#7388,#7389,#7390,#7391,#7392,#7393,#7394,
#7395,#7396,#7397,#7398,#7399,#7400,#7401,#7402,#7403,#7404,#7405,#7406,
#7407,#7408,#7409,#7410,#7411,#7412,#7413,#7414,#7415,#7416,#7417,#7418,
#7419,#7420,#7421,#7422),.UNSPECIFIED.,.F.,.F.,(4,3,3,3,3,3,3,3,3,3,3,3,
3,3,3,3,3,3,3,3,3,3,3,3,3,3,3,4),(53.4070751111526,53.4899407286186,53.5728065866223,
53.6556666653888,53.7385482014372,53.8087416244751,53.8919463874721,53.9751349198181,
54.0583266670012,54.1415128266491,54.224721093554,54.307606706722,54.390811469719,
54.4740000020651,54.5571917492483,54.6403779088962,54.7235861758011,54.8064717889688,
54.8896765519659,54.9728650843119,55.056056831495,55.1392429911428,55.2224512580478,
55.3053368712157,55.3885448552999,55.4717348798802,55.5549254912121,55.6326489767496),
 .UNSPECIFIED.);
#175=B_SPLINE_CURVE_WITH_KNOTS('',3,(#7423,#7424,#7425,#7426,#7427,#7428,
#7429,#7430,#7431,#7432,#7433,#7434,#7435,#7436,#7437,#7438,#7439,#7440,
#7441,#7442,#7443,#7444,#7445,#7446,#7447,#7448,#7449,#7450,#7451,#7452,
#7453,#7454,#7455,#7456,#7457,#7458,#7459,#7460,#7461,#7462,#7463,#7464,
#7465,#7466,#7467,#7468,#7469,#7470,#7471,#7472,#7473,#7474,#7475,#7476,
#7477,#7478,#7479,#7480,#7481,#7482,#7483,#7484,#7485,#7486,#7487,#7488,
#7489,#7490,#7491,#7492,#7493,#7494,#7495,#7496,#7497,#7498,#7499,#7500,
#7501,#7502,#7503,#7504,#7505,#7506,#7507,#7508,#7509,#7510,#7511,#7512,
#7513,#7514,#7515,#7516,#7517,#7518,#7519,#7520,#7521,#7522,#7523,#7524,
#7525,#7526,#7527,#7528,#7529,#7530,#7531,#7532,#7533,#7534,#7535,#7536,
#7537,#7538,#7539,#7540,#7541,#7542,#7543,#7544,#7545,#7546,#7547,#7548,
#7549,#7550,#7551,#7552,#7553,#7554,#7555,#7556,#7557,#7558,#7559,#7560,
#7561,#7562,#7563,#7564,#7565,#7566,#7567,#7568,#7569,#7570,#7571,#7572,
#7573),.UNSPECIFIED.,.F.,.F.,(4,3,3,3,3,3,3,3,3,3,3,3,3,3,3,3,3,3,3,3,3,
3,3,3,3,3,3,3,3,3,3,3,3,3,3,3,3,3,3,3,3,3,3,3,3,3,3,3,3,3,4),(49.349485040032,
49.432683045519,49.5158673552897,49.5990562489482,49.6822420940411,49.7654475102057,
49.8178209665001,49.9010257294971,49.984214261843,50.0674060090262,50.150592168674,
50.233800435579,50.316686048747,50.399890811744,50.48307934409,50.5662710912732,
50.649457250921,50.732665517826,50.8155511309938,50.8987558939908,50.9819444263367,
51.0651361735199,51.1483223331677,51.2315306000727,51.3144162132407,51.3976209762378,
51.4808095085838,51.564001255767,51.6471874154149,51.7303956823199,51.8132812954876,
51.8964860584847,51.9796745908306,52.0628663380137,52.1460524976615,52.2292607645664,
52.3121463777345,52.3953511407315,52.4785396730773,52.5617314202605,52.6449175799084,
52.7281258468134,52.8110114599813,52.8942162229782,52.977404755324,53.060596502507,
53.1437826621548,53.2269909290597,53.3098765422282,53.3983951832703,53.4070751110264),
 .UNSPECIFIED.);
#176=B_SPLINE_CURVE_WITH_KNOTS('',3,(#7579,#7580,#7581,#7582,#7583,#7584,
#7585,#7586,#7587,#7588,#7589,#7590,#7591,#7592,#7593,#7594,#7595,#7596,
#7597,#7598,#7599,#7600,#7601,#7602,#7603,#7604,#7605,#7606,#7607,#7608,
#7609,#7610,#7611,#7612,#7613,#7614,#7615,#7616,#7617,#7618,#7619,#7620,
#7621,#7622,#7623,#7624,#7625,#7626,#7627,#7628,#7629,#7630,#7631,#7632,
#7633,#7634,#7635,#7636,#7637,#7638,#7639,#7640,#7641,#7642,#7643,#7644,
#7645,#7646,#7647,#7648,#7649,#7650,#7651,#7652,#7653,#7654,#7655,#7656,
#7657,#7658,#7659,#7660,#7661,#7662,#7663,#7664,#7665,#7666,#7667,#7668,
#7669,#7670,#7671,#7672,#7673,#7674,#7675,#7676,#7677,#7678,#7679,#7680,
#7681,#7682,#7683,#7684,#7685,#7686,#7687,#7688,#7689,#7690,#7691,#7692,
#7693,#7694,#7695,#7696,#7697,#7698,#7699,#7700,#7701,#7702,#7703,#7704,
#7705,#7706,#7707,#7708,#7709,#7710,#7711,#7712,#7713,#7714,#7715,#7716,
#7717,#7718,#7719,#7720,#7721,#7722,#7723,#7724,#7725,#7726,#7727,#7728,
#7729),.UNSPECIFIED.,.F.,.F.,(4,3,3,3,3,3,3,3,3,3,3,3,3,3,3,3,3,3,3,3,3,
3,3,3,3,3,3,3,3,3,3,3,3,3,3,3,3,3,3,3,3,3,3,3,3,3,3,3,3,3,4),(43.0662846573068,
43.1494705378359,43.2326756410144,43.2802338464041,43.3634386094009,43.4466271417468,
43.5298188889299,43.6130050485777,43.6962133154828,43.779098928651,43.8623036916481,
43.945492223994,44.0286839711771,44.1118701308249,44.1950783977299,44.2779640108978,
44.3611687738949,44.4443573062409,44.5275490534239,44.6107352130717,44.6939434799768,
44.7768290931447,44.8600338561417,44.9432223884882,45.0264141356714,45.1096002953193,
45.1928085622243,45.2756941753916,45.3588989383885,45.4420874707345,45.5252792179175,
45.6084653775653,45.6916736444701,45.7745592576385,45.8577640206358,45.9409525529818,
46.0241443001649,46.1073304598125,46.1905387267174,46.2734243398853,46.3566291028823,
46.439817635228,46.5230093824112,46.6061955420591,46.6894038089641,46.7722894221322,
46.8553557362354,46.9384085402281,47.0214499107393,47.1044938151874,47.1238898038469),
 .UNSPECIFIED.);
#177=B_SPLINE_CURVE_WITH_KNOTS('',3,(#7730,#7731,#7732,#7733,#7734,#7735,
#7736,#7737,#7738,#7739,#7740,#7741,#7742,#7743,#7744,#7745,#7746,#7747,
#7748,#7749,#7750,#7751,#7752,#7753,#7754,#7755,#7756,#7757,#7758,#7759,
#7760,#7761,#7762,#7763,#7764,#7765,#7766,#7767,#7768,#7769,#7770,#7771,
#7772,#7773,#7774,#7775,#7776,#7777,#7778,#7779,#7780,#7781,#7782,#7783,
#7784,#7785,#7786,#7787,#7788,#7789,#7790,#7791,#7792,#7793,#7794,#7795,
#7796,#7797,#7798,#7799,#7800,#7801,#7802,#7803,#7804,#7805,#7806,#7807,
#7808,#7809,#7810,#7811),.UNSPECIFIED.,.F.,.F.,(4,3,3,3,3,3,3,3,3,3,3,3,
3,3,3,3,3,3,3,3,3,3,3,3,3,3,3,4),(47.1238898039573,47.2105854036145,47.2711545043791,
47.3543592673762,47.4375477997221,47.5207395469052,47.603925706553,47.6871339734579,
47.770019586626,47.8532243496231,47.9364128819692,48.0196046291524,48.1027907888001,
48.1859990557052,48.2688846688728,48.3520894318698,48.4352779642157,48.5184697113989,
48.6016558710467,48.6848641379517,48.7677497511197,48.8509545141168,48.9341430464628,
49.017334793646,49.1005209532939,49.183729220199,49.2666148333666,49.3494924806201),
 .UNSPECIFIED.);
#178=B_SPLINE_CURVE_WITH_KNOTS('',3,(#7813,#7814,#7815,#7816,#7817,#7818,
#7819,#7820,#7821,#7822,#7823,#7824,#7825,#7826,#7827,#7828,#7829,#7830,
#7831,#7832,#7833,#7834,#7835,#7836,#7837,#7838,#7839,#7840,#7841,#7842,
#7843,#7844,#7845,#7846,#7847,#7848,#7849,#7850,#7851,#7852,#7853,#7854,
#7855,#7856,#7857,#7858,#7859,#7860,#7861,#7862,#7863,#7864,#7865,#7866,
#7867,#7868,#7869,#7870,#7871,#7872,#7873,#7874,#7875,#7876,#7877,#7878,
#7879,#7880,#7881,#7882,#7883,#7884,#7885,#7886,#7887,#7888,#7889,#7890,
#7891,#7892,#7893,#7894,#7895,#7896,#7897),.UNSPECIFIED.,.F.,.F.,(4,3,3,
3,3,3,3,3,3,3,3,3,3,3,3,3,3,3,3,3,3,3,3,3,3,3,3,3,4),(47.1238898039889,
47.2091197733778,47.2943777275482,47.3234955552657,47.4067003182626,47.4898888506086,
47.5730805977918,47.6562667574395,47.7394750243445,47.8223606375126,47.9055654005096,
47.9887539328555,48.0719456800387,48.1551318396864,48.2383401065915,48.3212257197594,
48.4044304827564,48.4876190151023,48.5708107622854,48.6539969219332,48.7372051888382,
48.8200908020063,48.9032955650034,48.9864840973494,49.0696758445326,49.1528620041804,
49.2360702710854,49.3189558842532,49.349485040032),.UNSPECIFIED.);
#179=B_SPLINE_CURVE_WITH_KNOTS('',3,(#7898,#7899,#7900,#7901,#7902,#7903,
#7904,#7905,#7906,#7907,#7908,#7909,#7910,#7911,#7912,#7913,#7914,#7915,
#7916,#7917,#7918,#7919,#7920,#7921,#7922,#7923,#7924,#7925,#7926,#7927,
#7928,#7929,#7930,#7931,#7932,#7933,#7934,#7935,#7936,#7937,#7938,#7939,
#7940,#7941,#7942,#7943,#7944,#7945,#7946,#7947,#7948,#7949,#7950,#7951,
#7952,#7953,#7954,#7955,#7956,#7957,#7958,#7959,#7960,#7961,#7962,#7963,
#7964,#7965,#7966,#7967,#7968,#7969,#7970,#7971,#7972,#7973,#7974,#7975,
#7976,#7977,#7978,#7979,#7980,#7981,#7982,#7983,#7984,#7985,#7986,#7987,
#7988,#7989,#7990,#7991,#7992,#7993,#7994,#7995,#7996,#7997,#7998,#7999,
#8000,#8001,#8002,#8003,#8004,#8005,#8006,#8007,#8008,#8009,#8010,#8011,
#8012,#8013,#8014,#8015,#8016,#8017,#8018,#8019,#8020,#8021,#8022,#8023,
#8024,#8025,#8026,#8027,#8028,#8029,#8030,#8031,#8032,#8033,#8034,#8035,
#8036,#8037,#8038,#8039,#8040,#8041,#8042,#8043,#8044,#8045,#8046,#8047,
#8048),.UNSPECIFIED.,.F.,.F.,(4,3,3,3,3,3,3,3,3,3,3,3,3,3,3,3,3,3,3,3,3,
3,3,3,3,3,3,3,3,3,3,3,3,3,3,3,3,3,3,3,3,3,3,3,3,3,3,3,3,3,4),(43.066293790228,
43.1494805290637,43.2326671870035,43.3158711701376,43.3325748972907,43.4157796602877,
43.4989681926337,43.5821599398169,43.6653460994647,43.7485543663697,43.8314399795375,
43.9146447425345,43.9978332748805,44.0810250220636,44.1642111817114,44.2474194486164,
44.3303050617844,44.4135098247815,44.4966983571275,44.5798901043107,44.6630762639585,
44.7462845308635,44.8291701440313,44.9123749070284,44.9955634393744,45.0787551865576,
45.1619413462055,45.2451496131105,45.3280352262782,45.4112399892752,45.4944285216212,
45.5776202688043,45.6608064284521,45.7440146953571,45.8269003085251,45.9101050715222,
45.993293603868,46.0764853510512,46.159671510699,46.242879777604,46.3257653907719,
46.4089701537688,46.4921586861147,46.5753504332978,46.6585365929456,46.7417448598505,
46.8246304730188,46.9081622099044,46.9916752427181,47.0751808263689,47.1238898038469),
 .UNSPECIFIED.);
#180=B_SPLINE_CURVE_WITH_KNOTS('',3,(#8054,#8055,#8056,#8057,#8058,#8059,
#8060,#8061,#8062,#8063,#8064,#8065,#8066),.UNSPECIFIED.,.F.,.F.,(4,1,1,
1,1,1,1,1,1,1,4),(36.7831013013255,36.7949877771947,37.2938528594415,37.7927179416884,
38.2915830239353,38.7904481061822,39.2893131884291,39.7881782706759,40.2870433529228,
40.7859084351697,40.8407044966673),.UNSPECIFIED.);
#181=B_SPLINE_CURVE_WITH_KNOTS('',3,(#8067,#8068,#8069,#8070,#8071,#8072,
#8073,#8074,#8075,#8076,#8077,#8078,#8079,#8080,#8081,#8082,#8083,#8084,
#8085,#8086,#8087,#8088,#8089,#8090,#8091,#8092,#8093,#8094,#8095,#8096,
#8097,#8098,#8099,#8100,#8101,#8102,#8103,#8104,#8105,#8106,#8107,#8108,
#8109,#8110,#8111,#8112,#8113,#8114,#8115,#8116,#8117,#8118,#8119,#8120,
#8121,#8122,#8123,#8124,#8125,#8126,#8127,#8128,#8129,#8130,#8131,#8132,
#8133,#8134,#8135,#8136,#8137,#8138,#8139,#8140,#8141,#8142,#8143,#8144,
#8145,#8146,#8147,#8148,#8149,#8150,#8151),.UNSPECIFIED.,.F.,.F.,(4,3,3,
3,3,3,3,3,3,3,3,3,3,3,3,3,3,3,3,3,3,3,3,3,3,3,3,3,4),(40.8407044966673,
40.9236082621666,41.0064970381205,41.0893890046342,41.1722791221436,41.255188027838,
41.2847735174166,41.3679782804136,41.4511668127597,41.5343585599429,41.6175447195908,
41.7007529864957,41.7836385996634,41.8668433626605,41.9500318950066,42.0332236421897,
42.1164098018374,42.1996180687424,42.2825036819103,42.3657084449074,42.4488969772536,
42.5320887244368,42.6152748840845,42.6984831509895,42.7813687641572,42.8645746921478,
42.9477630246613,43.0309462152979,43.0662846573068),.UNSPECIFIED.);
#182=B_SPLINE_CURVE_WITH_KNOTS('',3,(#8153,#8154,#8155,#8156,#8157,#8158,
#8159,#8160,#8161,#8162,#8163,#8164,#8165,#8166,#8167,#8168,#8169,#8170,
#8171,#8172,#8173,#8174,#8175,#8176,#8177,#8178,#8179,#8180,#8181,#8182,
#8183,#8184,#8185,#8186,#8187,#8188,#8189,#8190,#8191,#8192,#8193,#8194,
#8195,#8196,#8197,#8198,#8199,#8200,#8201,#8202,#8203,#8204,#8205,#8206,
#8207,#8208,#8209,#8210,#8211,#8212,#8213,#8214,#8215,#8216,#8217,#8218,
#8219,#8220,#8221,#8222,#8223,#8224,#8225,#8226,#8227,#8228,#8229,#8230,
#8231,#8232,#8233,#8234),.UNSPECIFIED.,.F.,.F.,(4,3,3,3,3,3,3,3,3,3,3,3,
3,3,3,3,3,3,3,3,3,3,3,3,3,3,3,4),(40.8407044966673,40.9238896807017,41.007058573913,
41.0902305668682,41.1733970921888,41.2565855470319,41.3371145683032,41.4203193313002,
41.5035078636461,41.5866996108293,41.6698857704772,41.7530940373822,41.83597965055,
41.9191844135471,42.002372945893,42.0855646930761,42.1687508527239,42.2519591196289,
42.3348447327969,42.418049495794,42.50123802814,42.5844297753232,42.6676159349711,
42.7508242018762,42.8337098150438,42.9169142021957,43.0001074756034,43.066293790228),
 .UNSPECIFIED.);
#183=B_SPLINE_CURVE_WITH_KNOTS('',3,(#8235,#8236,#8237,#8238,#8239,#8240,
#8241,#8242,#8243,#8244,#8245,#8246,#8247,#8248,#8249,#8250,#8251,#8252,
#8253,#8254,#8255,#8256,#8257,#8258,#8259,#8260,#8261,#8262,#8263,#8264,
#8265,#8266,#8267,#8268,#8269,#8270,#8271,#8272,#8273,#8274,#8275,#8276,
#8277,#8278,#8279,#8280,#8281,#8282,#8283,#8284,#8285,#8286,#8287,#8288,
#8289,#8290,#8291,#8292,#8293,#8294,#8295,#8296,#8297,#8298,#8299,#8300,
#8301,#8302,#8303,#8304,#8305,#8306,#8307,#8308,#8309,#8310,#8311,#8312,
#8313,#8314,#8315,#8316,#8317,#8318,#8319,#8320,#8321,#8322,#8323,#8324,
#8325,#8326,#8327,#8328,#8329,#8330,#8331,#8332,#8333,#8334,#8335,#8336,
#8337,#8338,#8339,#8340,#8341,#8342,#8343,#8344,#8345,#8346,#8347,#8348,
#8349,#8350,#8351,#8352,#8353,#8354,#8355,#8356,#8357,#8358,#8359,#8360,
#8361,#8362,#8363,#8364,#8365,#8366,#8367,#8368,#8369,#8370,#8371,#8372,
#8373,#8374,#8375,#8376,#8377,#8378,#8379,#8380,#8381,#8382,#8383,#8384,
#8385),.UNSPECIFIED.,.F.,.F.,(4,3,3,3,3,3,3,3,3,3,3,3,3,3,3,3,3,3,3,3,3,
3,3,3,3,3,3,3,3,3,3,3,3,3,3,3,3,3,3,3,3,3,3,3,3,3,3,3,3,3,4),(36.7830907836671,
36.8473288280813,36.9305335910781,37.0137221234244,37.0969138706075,37.1801000302554,
37.2633082971604,37.3461939103281,37.4293986733251,37.512587205671,37.595778952854,
37.6789651125019,37.762173379407,37.845058992575,37.928263755572,38.011452287918,
38.0946440351011,38.1778301947487,38.2610384616539,38.3439240748219,38.427128837819,
38.5103173701645,38.5935091173477,38.6766952769955,38.7599035439005,38.8427891570688,
38.9259939200658,39.009182452412,39.0923741995953,39.1755603592432,39.2587686261481,
39.3416542393157,39.4248590023125,39.5080475346586,39.5912392818417,39.6744254414893,
39.7576337083944,39.8405193215625,39.9237240845596,40.0069126169054,40.0901043640886,
40.1732905237363,40.2564987906412,40.3393844038094,40.4225891668065,40.5057776991523,
40.5889694463354,40.6721556059833,40.7553638728884,40.8382494860563,40.8407044963635),
 .UNSPECIFIED.);
#184=B_SPLINE_CURVE_WITH_KNOTS('',3,(#8391,#8392,#8393,#8394,#8395,#8396,
#8397,#8398,#8399,#8400,#8401,#8402,#8403,#8404,#8405,#8406,#8407,#8408,
#8409,#8410,#8411,#8412,#8413,#8414,#8415,#8416,#8417,#8418,#8419,#8420,
#8421,#8422,#8423,#8424,#8425,#8426,#8427,#8428,#8429,#8430,#8431,#8432,
#8433,#8434,#8435,#8436,#8437,#8438,#8439,#8440,#8441,#8442,#8443,#8444,
#8445,#8446,#8447,#8448,#8449,#8450,#8451,#8452,#8453,#8454,#8455,#8456,
#8457,#8458,#8459,#8460,#8461,#8462,#8463,#8464,#8465,#8466,#8467,#8468,
#8469,#8470,#8471,#8472,#8473,#8474,#8475,#8476,#8477,#8478,#8479,#8480,
#8481,#8482,#8483,#8484,#8485,#8486,#8487,#8488,#8489,#8490,#8491,#8492,
#8493,#8494,#8495,#8496,#8497,#8498,#8499,#8500,#8501,#8502,#8503,#8504,
#8505,#8506,#8507,#8508,#8509,#8510,#8511,#8512,#8513,#8514,#8515,#8516,
#8517,#8518,#8519,#8520,#8521,#8522,#8523,#8524,#8525,#8526,#8527,#8528,
#8529,#8530,#8531,#8532,#8533,#8534,#8535,#8536,#8537,#8538),
 .UNSPECIFIED.,.F.,.F.,(4,3,3,3,3,3,3,3,3,3,3,3,3,3,3,3,3,3,3,3,3,3,3,3,
3,3,3,3,3,3,3,3,3,3,3,3,3,3,3,3,3,3,3,3,3,3,3,3,3,4),(30.4999301101848,
30.5831195524751,30.6663053868848,30.7495113023812,30.8086067902321,30.8918115532291,
30.9750000855751,31.0581918327582,31.141377992406,31.224586259311,31.307471872479,
31.3906766354761,31.473865167822,31.5570569150052,31.6402430746531,31.7234513415581,
31.8063369547259,31.889541717723,31.972730250069,32.0559219972522,32.1391081569,
32.222316423805,32.3052020369728,32.3884067999698,32.4715953323158,32.5547870794989,
32.6379732391468,32.7211815060518,32.8040671192197,32.8872718822167,32.9704604145627,
33.0536521617459,33.1368383213936,33.2200465882987,33.3029322014665,33.3861369644635,
33.4693254968094,33.5525172439925,33.6357034036404,33.7189116705454,33.8017972837134,
33.8850020467105,33.9681905790564,34.0513823262396,34.1345684858875,34.2177767527926,
34.3006623659603,34.3847827412953,34.4711509653915,34.5575191894877),
 .UNSPECIFIED.);
#185=B_SPLINE_CURVE_WITH_KNOTS('',3,(#8539,#8540,#8541,#8542,#8543,#8544,
#8545,#8546),.UNSPECIFIED.,.F.,.F.,(4,1,1,1,1,4),(34.5575191949046,34.7995274482072,
35.298392530454,35.7972576127009,36.2961226949478,36.7831013013255),
 .UNSPECIFIED.);
#186=B_SPLINE_CURVE_WITH_KNOTS('',3,(#8548,#8549,#8550,#8551,#8552,#8553,
#8554,#8555,#8556,#8557,#8558,#8559,#8560,#8561,#8562,#8563,#8564,#8565,
#8566,#8567,#8568,#8569,#8570,#8571,#8572,#8573,#8574,#8575,#8576,#8577,
#8578,#8579,#8580,#8581,#8582,#8583,#8584,#8585,#8586,#8587,#8588,#8589,
#8590,#8591,#8592,#8593,#8594,#8595,#8596,#8597,#8598,#8599,#8600,#8601,
#8602,#8603,#8604,#8605,#8606,#8607,#8608,#8609,#8610,#8611,#8612,#8613,
#8614,#8615,#8616,#8617,#8618,#8619,#8620,#8621,#8622,#8623,#8624,#8625,
#8626,#8627,#8628,#8629,#8630,#8631,#8632),.UNSPECIFIED.,.F.,.F.,(4,3,3,
3,3,3,3,3,3,3,3,3,3,3,3,3,3,3,3,3,3,3,3,3,3,3,3,3,4),(34.5575191894877,
34.6410858833927,34.7246534185875,34.8082419415075,34.8518684990938,34.9350732620908,
35.0182617944371,35.1014535416203,35.1846397012681,35.2678479681731,35.3507335813406,
35.4339383443377,35.5171268766836,35.6003186238667,35.6835047835147,35.7667130504196,
35.8495986635875,35.9328034265846,36.0159919589303,36.0991837061135,36.1823698657615,
36.2655781326667,36.3484637458344,36.4316678909786,36.5148555434348,36.5980411279957,
36.6812216768781,36.7644129039734,36.7830907836671),.UNSPECIFIED.);
#187=B_SPLINE_CURVE_WITH_KNOTS('',3,(#8633,#8634,#8635,#8636,#8637,#8638,
#8639,#8640,#8641,#8642,#8643,#8644,#8645,#8646,#8647,#8648,#8649,#8650,
#8651,#8652,#8653,#8654,#8655,#8656,#8657,#8658,#8659,#8660,#8661,#8662,
#8663,#8664,#8665,#8666,#8667,#8668,#8669,#8670,#8671,#8672,#8673,#8674,
#8675,#8676,#8677,#8678,#8679,#8680,#8681,#8682,#8683,#8684,#8685,#8686,
#8687,#8688,#8689,#8690,#8691,#8692,#8693,#8694,#8695,#8696,#8697,#8698,
#8699,#8700,#8701,#8702,#8703,#8704,#8705,#8706,#8707,#8708,#8709,#8710,
#8711,#8712,#8713,#8714,#8715,#8716,#8717,#8718,#8719,#8720,#8721,#8722,
#8723,#8724,#8725,#8726,#8727,#8728,#8729,#8730,#8731,#8732,#8733,#8734,
#8735,#8736,#8737,#8738,#8739,#8740,#8741,#8742,#8743,#8744,#8745,#8746,
#8747,#8748,#8749,#8750,#8751,#8752,#8753,#8754,#8755,#8756,#8757,#8758,
#8759,#8760,#8761,#8762,#8763,#8764,#8765,#8766,#8767,#8768,#8769,#8770,
#8771,#8772,#8773,#8774,#8775,#8776,#8777,#8778,#8779,#8780,#8781,#8782,
#8783),.UNSPECIFIED.,.F.,.F.,(4,3,3,3,3,3,3,3,3,3,3,3,3,3,3,3,3,3,3,3,3,
3,3,3,3,3,3,3,3,3,3,3,3,3,3,3,3,3,3,3,3,3,3,3,3,3,3,3,3,3,4),(30.4999360201024,
30.5831176496859,30.6663049468445,30.7494912023174,30.8326954253169,30.8609478411187,
30.9441526041158,31.0273411364619,31.1105328836451,31.193719043293,31.2769273101981,
31.3598129233656,31.4430176863626,31.5262062187086,31.6093979658918,31.6925841255396,
31.7757923924446,31.8586780056125,31.9418827686095,32.0250713009555,32.1082630481386,
32.1914492077864,32.2746574746914,32.3575430878594,32.4407478508565,32.5239363832024,
32.6071281303855,32.6903142900333,32.7735225569383,32.8564081701062,32.9396129331032,
33.0228014654491,33.1059932126322,33.1891793722801,33.272387639185,33.3552732523531,
33.4384780153501,33.5216665476963,33.6048582948794,33.6880444545274,33.7712527214324,
33.8541383346,33.937343097597,34.0205316299431,34.1037233771263,34.1869095367742,
34.2701178036792,34.3530034168469,34.4381472840239,34.5232671972151,34.5575191893576),
 .UNSPECIFIED.);
#188=B_SPLINE_CURVE_WITH_KNOTS('',3,(#8789,#8790,#8791,#8792,#8793,#8794,
#8795,#8796,#8797,#8798,#8799,#8800,#8801,#8802,#8803,#8804,#8805,#8806,
#8807,#8808,#8809,#8810,#8811,#8812,#8813,#8814,#8815,#8816,#8817,#8818,
#8819,#8820,#8821,#8822,#8823,#8824,#8825,#8826,#8827,#8828,#8829,#8830,
#8831,#8832,#8833,#8834,#8835,#8836,#8837,#8838,#8839,#8840,#8841,#8842,
#8843,#8844,#8845,#8846,#8847,#8848,#8849,#8850,#8851,#8852,#8853,#8854,
#8855,#8856,#8857,#8858,#8859,#8860,#8861,#8862,#8863,#8864,#8865,#8866,
#8867,#8868,#8869,#8870,#8871,#8872,#8873,#8874,#8875,#8876,#8877,#8878,
#8879,#8880,#8881,#8882,#8883,#8884,#8885,#8886,#8887,#8888,#8889,#8890,
#8891,#8892,#8893,#8894,#8895,#8896,#8897,#8898,#8899,#8900,#8901,#8902,
#8903,#8904,#8905,#8906,#8907,#8908,#8909,#8910,#8911,#8912,#8913,#8914,
#8915,#8916,#8917,#8918,#8919,#8920,#8921,#8922,#8923,#8924,#8925,#8926,
#8927,#8928,#8929,#8930,#8931,#8932,#8933,#8934,#8935,#8936,#8937,#8938,
#8939),.UNSPECIFIED.,.F.,.F.,(4,3,3,3,3,3,3,3,3,3,3,3,3,3,3,3,3,3,3,3,3,
3,3,3,3,3,3,3,3,3,3,3,3,3,3,3,3,3,3,3,3,3,3,3,3,3,3,3,3,3,4),(24.216717884951,
24.299921981893,24.3233607210227,24.4065654840083,24.4897540163421,24.5729457635133,
24.656131923149,24.7393401900419,24.8222258032696,24.905430566277,24.9886190986334,
25.0718108458273,25.1549970054856,25.2382052724013,25.3210908855165,25.4042956485073,
25.4874841808471,25.5706759280239,25.6538620876651,25.7370703545637,25.8199559677634,
25.9031607307635,25.9863492631122,26.0695410102983,26.1527271699493,26.2359354368573,
26.3188210500103,26.4020258130063,26.4852143453511,26.5684060925334,26.6515922521803,
26.7348005190843,26.8176861322571,26.9008908952543,26.9840794276,27.0672711747833,
27.150457334431,27.2336656013361,27.316551214504,27.3997559775011,27.4829445098478,
27.5661362570311,27.649322416679,27.7325306835841,27.8154162967509,27.8983765004895,
27.9813196738763,28.0642637478914,28.1472037199699,28.2301616567405,28.2743338821564),
 .UNSPECIFIED.);
#189=B_SPLINE_CURVE_WITH_KNOTS('',3,(#8940,#8941,#8942,#8943,#8944,#8945,
#8946,#8947,#8948,#8949,#8950,#8951,#8952,#8953,#8954,#8955,#8956,#8957,
#8958,#8959,#8960,#8961,#8962,#8963,#8964,#8965,#8966,#8967,#8968,#8969,
#8970,#8971,#8972,#8973,#8974,#8975,#8976,#8977,#8978,#8979,#8980,#8981,
#8982,#8983,#8984,#8985,#8986,#8987,#8988,#8989,#8990,#8991,#8992,#8993,
#8994,#8995,#8996,#8997,#8998,#8999,#9000,#9001,#9002,#9003,#9004,#9005,
#9006,#9007,#9008,#9009,#9010,#9011,#9012,#9013,#9014,#9015,#9016,#9017,
#9018,#9019,#9020,#9021,#9022,#9023,#9024),.UNSPECIFIED.,.F.,.F.,(4,3,3,
3,3,3,3,3,3,3,3,3,3,3,3,3,3,3,3,3,3,3,3,3,3,3,3,3,4),(28.2743338823081,
28.3142813789978,28.397486141995,28.4806746743415,28.5638664215248,28.6470525811728,
28.730260848078,28.8131464612446,28.8963512242415,28.9795397565875,29.0627315037705,
29.1459176634183,29.2291259303233,29.3120115434915,29.3952163064886,29.4784048388345,
29.5615965860178,29.6447827456656,29.7279910125707,29.8108766257384,29.8940813887354,
29.9772699210814,30.0604616682645,30.1436478279123,30.2268560948173,30.3097417079853,
30.3929456544943,30.4761344023573,30.4999301101848),.UNSPECIFIED.);
#190=B_SPLINE_CURVE_WITH_KNOTS('',3,(#9026,#9027,#9028,#9029,#9030,#9031,
#9032,#9033,#9034,#9035,#9036,#9037,#9038,#9039,#9040,#9041,#9042,#9043,
#9044,#9045,#9046,#9047,#9048,#9049,#9050,#9051,#9052,#9053,#9054,#9055,
#9056,#9057,#9058,#9059,#9060,#9061,#9062,#9063,#9064,#9065,#9066,#9067,
#9068,#9069,#9070,#9071,#9072,#9073,#9074,#9075,#9076,#9077,#9078,#9079,
#9080,#9081,#9082,#9083,#9084,#9085,#9086,#9087,#9088,#9089,#9090,#9091,
#9092,#9093,#9094,#9095,#9096,#9097,#9098,#9099,#9100,#9101,#9102,#9103,
#9104,#9105,#9106,#9107),.UNSPECIFIED.,.F.,.F.,(4,3,3,3,3,3,3,3,3,3,3,3,
3,3,3,3,3,3,3,3,3,3,3,3,3,3,3,4),(28.2743338823081,28.3666224298844,28.4498271928843,
28.5330157252333,28.6162074724194,28.6993936320702,28.7826018989782,28.8654875121312,
28.9486922751272,29.0318808074722,29.1150725546544,29.1982587143012,29.2814669812052,
29.3643525943781,29.4475573573753,29.5307458897214,29.6139376369048,29.6971237965528,
29.780332063458,29.863217676625,29.9464224396222,30.0296109719682,30.1128027191515,
30.1959888787995,30.2791971457046,30.3620827588719,30.4452883358325,30.4999360201024),
 .UNSPECIFIED.);
#191=B_SPLINE_CURVE_WITH_KNOTS('',3,(#9108,#9109,#9110,#9111,#9112,#9113,
#9114,#9115,#9116,#9117,#9118,#9119,#9120,#9121,#9122,#9123,#9124,#9125,
#9126,#9127,#9128,#9129,#9130,#9131,#9132,#9133,#9134,#9135,#9136,#9137,
#9138,#9139,#9140,#9141,#9142,#9143,#9144,#9145,#9146,#9147,#9148,#9149,
#9150,#9151,#9152,#9153,#9154,#9155,#9156,#9157,#9158,#9159,#9160,#9161,
#9162,#9163,#9164,#9165,#9166,#9167,#9168,#9169,#9170,#9171,#9172,#9173,
#9174,#9175,#9176,#9177,#9178,#9179,#9180,#9181,#9182,#9183,#9184,#9185,
#9186,#9187,#9188,#9189,#9190,#9191,#9192,#9193,#9194,#9195,#9196,#9197,
#9198,#9199,#9200,#9201,#9202,#9203,#9204,#9205,#9206,#9207,#9208,#9209,
#9210,#9211,#9212,#9213,#9214,#9215,#9216,#9217,#9218,#9219,#9220,#9221,
#9222,#9223,#9224,#9225,#9226,#9227,#9228,#9229,#9230,#9231,#9232,#9233,
#9234,#9235,#9236,#9237,#9238,#9239,#9240,#9241,#9242,#9243,#9244,#9245,
#9246,#9247,#9248,#9249,#9250,#9251,#9252,#9253,#9254,#9255),
 .UNSPECIFIED.,.F.,.F.,(4,3,3,3,3,3,3,3,3,3,3,3,3,3,3,3,3,3,3,3,3,3,3,3,
3,3,3,3,3,3,3,3,3,3,3,3,3,3,3,3,3,3,3,3,3,3,3,3,3,4),(24.2167209753283,
24.2999284446391,24.3757017719093,24.4589065342714,24.5420950659734,24.6252868125053,
24.7084729714987,24.791681237751,24.8745668541562,24.9577716175062,25.0409601502098,
25.1241518977543,25.2073380577647,25.2905463250312,25.3734319364031,25.4566366992492,
25.5398252314424,25.6230169784713,25.7062031379642,25.7894114047152,25.87229701865,
25.9555017816906,26.0386903140807,26.1218820613081,26.2050682210001,26.2882764879492,
26.3711621008968,26.4543668638941,26.5375553962401,26.6207471434236,26.7039333030718,
26.7871415699773,26.8700271831437,26.953231946129,27.0364204784631,27.1196122256344,
27.2027983852704,27.2860066521636,27.3688922653906,27.452097028398,27.5352855607541,
27.618477307948,27.7016634676065,27.7848717345221,27.8677573476375,27.950630740422,
28.0334950107661,28.116348080326,28.1992149244415,28.2743338821488),
 .UNSPECIFIED.);
#192=B_SPLINE_CURVE_WITH_KNOTS('',3,(#9261,#9262,#9263,#9264,#9265,#9266,
#9267,#9268,#9269),.UNSPECIFIED.,.F.,.F.,(4,1,1,1,1,1,4),(15.7079632679489,
15.8949953737124,16.3938604559593,16.8927255382062,17.3915906204531,17.8904557026999,
17.9335636647299),.UNSPECIFIED.);
#193=B_SPLINE_CURVE_WITH_KNOTS('',3,(#9271,#9272,#9273,#9274,#9275,#9276),
 .UNSPECIFIED.,.F.,.F.,(4,1,1,4),(14.3984001269718,14.8972652092187,15.3961302914656,
15.7079632679489),.UNSPECIFIED.);
#194=B_SPLINE_CURVE_WITH_KNOTS('',3,(#9280,#9281,#9282,#9283,#9284,#9285,
#9286,#9287,#9288,#9289,#9290,#9291,#9292,#9293,#9294,#9295,#9296,#9297,
#9298,#9299,#9300,#9301,#9302,#9303,#9304,#9305,#9306,#9307,#9308,#9309,
#9310,#9311,#9312,#9313,#9314,#9315,#9316,#9317,#9318,#9319,#9320,#9321,
#9322,#9323,#9324,#9325,#9326,#9327,#9328,#9329,#9330,#9331,#9332,#9333,
#9334,#9335,#9336,#9337,#9338,#9339,#9340,#9341,#9342,#9343,#9344,#9345,
#9346,#9347,#9348,#9349),.UNSPECIFIED.,.F.,.F.,(4,3,3,3,3,3,3,3,3,3,3,3,
3,3,3,3,3,3,3,3,3,3,3,4),(13.8759337553362,13.9589611884219,14.0419725517034,
14.1249865839979,14.2079967440506,14.2910269801202,14.3460590760852,14.4292629924508,
14.51245069532,14.5956416479347,14.6788270336895,14.7620345691255,14.8449241583321,
14.9281250993385,15.0113097465424,15.0944975472168,15.1776797345729,15.2608840240016,
15.343789240579,15.4267884627978,15.5097751925943,15.592750663241,15.6757311232471,
15.7079632679489),.UNSPECIFIED.);
#195=B_SPLINE_CURVE_WITH_KNOTS('',3,(#9350,#9351,#9352,#9353,#9354,#9355,
#9356,#9357,#9358,#9359,#9360,#9361,#9362,#9363,#9364,#9365,#9366,#9367,
#9368,#9369,#9370,#9371,#9372,#9373,#9374,#9375,#9376,#9377,#9378,#9379,
#9380,#9381,#9382,#9383,#9384,#9385,#9386,#9387,#9388,#9389,#9390,#9391,
#9392,#9393,#9394,#9395,#9396,#9397,#9398,#9399,#9400,#9401,#9402,#9403,
#9404,#9405,#9406,#9407,#9408,#9409,#9410,#9411,#9412,#9413,#9414,#9415,
#9416,#9417,#9418,#9419,#9420,#9421,#9422,#9423,#9424,#9425,#9426,#9427,
#9428,#9429,#9430,#9431,#9432,#9433,#9434),.UNSPECIFIED.,.F.,.F.,(4,3,3,
3,3,3,3,3,3,3,3,3,3,3,3,3,3,3,3,3,3,3,3,3,3,3,3,3,4),(15.7079632680893,
15.7950775824961,15.8426543228258,15.9258568205529,16.0090430574305,16.0922324840386,
16.1754163139598,16.2586222581903,16.3415194050727,16.4247252502413,16.5079148782708,
16.5911077317026,16.6742950011921,16.7575043732806,16.8403844873196,16.9235888701302,
17.0067770180441,17.0899683778634,17.1731541493092,17.2563620303484,17.3392495695665,
17.4224543918057,17.5056429836855,17.5888347902833,17.672021009163,17.7552293344183,
17.8381146518133,17.921318645311,17.9335664739021),.UNSPECIFIED.);
#196=B_SPLINE_CURVE_WITH_KNOTS('',3,(#9440,#9441,#9442,#9443,#9444,#9445,
#9446,#9447,#9448,#9449,#9450,#9451,#9452,#9453,#9454,#9455,#9456,#9457,
#9458,#9459,#9460,#9461,#9462,#9463,#9464,#9465,#9466,#9467,#9468,#9469,
#9470,#9471,#9472,#9473,#9474,#9475,#9476,#9477,#9478,#9479,#9480,#9481,
#9482,#9483,#9484,#9485,#9486,#9487,#9488,#9489,#9490,#9491,#9492,#9493,
#9494,#9495,#9496,#9497,#9498,#9499,#9500,#9501,#9502,#9503,#9504,#9505,
#9506,#9507),.UNSPECIFIED.,.F.,.F.,(4,2,2,2,2,2,2,2,2,2,2,2,2,2,2,2,2,2,
2,2,2,2,2,2,2,2,2,2,2,2,2,2,2,4),(3.21211487024883E-5,0.0789352746093392,
0.125900885216109,0.194687536519382,0.235964866096197,0.260949154170126,
0.318423911537595,0.387900638259459,0.463726389496267,0.514560383592697,
0.580602031721947,0.645219715092042,0.720385217165228,0.769263684680726,
0.826314664490939,0.892514875423717,0.99193614383231,1.0300811327044,1.08495853522793,
1.15083401376278,1.24505839048266,1.2860599861693,1.34209173725548,1.4085307353683,
1.49904769502063,1.54210420930418,1.6033802411766,1.67075334491485,1.74659608796949,
1.79662732553455,1.85318325250244,1.92072567690366,2.01576766849767,2.0528946271821),
 .UNSPECIFIED.);
#197=B_SPLINE_CURVE_WITH_KNOTS('',3,(#9510,#9511,#9512,#9513,#9514,#9515,
#9516,#9517,#9518,#9519,#9520,#9521,#9522,#9523,#9524,#9525,#9526,#9527,
#9528,#9529,#9530,#9531,#9532,#9533,#9534,#9535,#9536,#9537,#9538,#9539,
#9540,#9541,#9542,#9543,#9544,#9545,#9546,#9547,#9548,#9549,#9550,#9551,
#9552,#9553,#9554,#9555,#9556,#9557,#9558,#9559,#9560,#9561,#9562,#9563,
#9564,#9565,#9566,#9567,#9568,#9569,#9570,#9571,#9572,#9573,#9574,#9575,
#9576,#9577,#9578,#9579,#9580,#9581,#9582,#9583,#9584,#9585,#9586,#9587,
#9588,#9589,#9590,#9591,#9592,#9593,#9594,#9595,#9596,#9597,#9598,#9599,
#9600,#9601,#9602,#9603,#9604,#9605,#9606,#9607),.UNSPECIFIED.,.F.,.F.,
(4,2,2,2,2,2,2,2,2,2,2,2,2,2,2,2,2,2,2,2,2,2,2,2,2,2,2,2,2,2,2,2,2,2,2,
2,2,2,2,2,2,2,2,2,2,2,2,2,4),(-5.86775810127551,-5.77865085129505,-5.72879583160343,
-5.64761852141392,-5.61689286788677,-5.54175378043255,-5.49593445407308,
-5.4210022791591,-5.36917519324587,-5.32999908682785,-5.26057884393074,
-5.20983829062336,-5.11311910543699,-5.05694894394058,-4.98922760967673,
-4.89378617981899,-4.85349774549445,-4.79705316735085,-4.73079766409471,
-4.6414271299511,-4.59765033110434,-4.53624621476361,-4.46895286460035,
-4.39375558925325,-4.3422088475698,-4.2887681416752,-4.21895559732193,-4.12372343019229,
-4.08333396673305,-4.02676275422254,-3.96056758056503,-3.87140429745958,
-3.8274912977314,-3.7659411752726,-3.69875702039177,-3.6270581440989,-3.57197264493549,
-3.51871698633678,-3.48379939085449,-3.45946983959537,-3.40770778211876,
-3.31627953506947,-3.25897883939447,-3.19263751159846,-3.09559065383727,
-3.05613493947002,-3.00105661676876,-2.93406942190934,-2.93406320703471),
 .UNSPECIFIED.);
#198=B_SPLINE_CURVE_WITH_KNOTS('',3,(#9613,#9614,#9615,#9616,#9617,#9618,
#9619,#9620,#9621,#9622,#9623,#9624,#9625,#9626,#9627,#9628,#9629,#9630,
#9631,#9632,#9633,#9634,#9635,#9636,#9637),.UNSPECIFIED.,.F.,.F.,(4,3,3,
3,3,3,3,3,4),(63.5596986986593,63.6465864533654,63.7334716784127,63.8203763732837,
63.8547305276003,63.9421373160612,64.0295237721704,64.116898968737,64.141416212773),
 .UNSPECIFIED.);
#199=B_SPLINE_CURVE_WITH_KNOTS('',3,(#9638,#9639,#9640,#9641,#9642,#9643,
#9644,#9645,#9646,#9647,#9648,#9649,#9650,#9651,#9652,#9653,#9654,#9655,
#9656,#9657,#9658,#9659,#9660,#9661,#9662,#9663,#9664,#9665,#9666,#9667,
#9668,#9669,#9670,#9671,#9672,#9673,#9674,#9675,#9676,#9677,#9678,#9679,
#9680,#9681,#9682,#9683,#9684,#9685,#9686,#9687,#9688,#9689,#9690,#9691,
#9692,#9693,#9694,#9695,#9696,#9697,#9698,#9699,#9700,#9701,#9702,#9703,
#9704,#9705,#9706,#9707,#9708,#9709,#9710,#9711,#9712,#9713,#9714,#9715,
#9716,#9717,#9718,#9719,#9720,#9721,#9722,#9723,#9724,#9725,#9726,#9727,
#9728,#9729,#9730,#9731,#9732,#9733,#9734,#9735,#9736,#9737),
 .UNSPECIFIED.,.F.,.F.,(4,2,2,2,2,2,2,2,2,2,2,2,2,2,2,2,2,2,2,2,2,2,2,2,
2,2,2,2,2,2,2,2,2,2,2,2,2,2,2,2,2,2,2,2,2,2,2,2,2,4),(2.0528946271821,2.05626576241009,
2.11302674968695,2.1830480906073,2.26413783199407,2.31157823672075,2.38070629598805,
2.44266215948112,2.49346033978971,2.56725647762745,2.61934692210331,2.69359183141892,
2.76083907262114,2.82229340458244,2.86610520161253,2.95542529828825,3.02169497932261,
3.07812176742366,3.11844011147168,3.2138055265495,3.27997468806069,3.33443328707101,
3.37351131970449,3.47132296969718,3.53831306246984,3.594430509328,3.64658886723371,
3.72050260660357,3.78778092905754,3.84919614272541,3.89300151309997,3.98233280802618,
4.04860055488936,4.10503243207252,4.14534577607919,4.24072351997691,4.3105533054657,
4.36390165735659,4.41591933462917,4.49067966246195,4.55794899396488,4.61937890270551,
4.6439987187184,4.69174215466658,4.75022353405068,4.79591121803213,4.84141672820665,
4.87360389107397,4.8998465902543,4.9868883946957),.UNSPECIFIED.);
#200=B_SPLINE_CURVE_WITH_KNOTS('',3,(#9739,#9740,#9741,#9742,#9743,#9744,
#9745,#9746,#9747,#9748,#9749,#9750,#9751,#9752,#9753,#9754,#9755,#9756,
#9757,#9758,#9759,#9760,#9761,#9762,#9763,#9764,#9765,#9766,#9767,#9768,
#9769,#9770,#9771,#9772,#9773,#9774,#9775,#9776,#9777,#9778,#9779,#9780,
#9781,#9782,#9783,#9784,#9785,#9786,#9787,#9788,#9789,#9790,#9791,#9792,
#9793,#9794,#9795,#9796,#9797,#9798,#9799,#9800,#9801,#9802,#9803,#9804,
#9805,#9806,#9807,#9808,#9809,#9810,#9811,#9812,#9813,#9814,#9815,#9816,
#9817,#9818,#9819,#9820,#9821,#9822,#9823,#9824,#9825,#9826,#9827,#9828,
#9829,#9830,#9831,#9832,#9833,#9834,#9835,#9836,#9837,#9838),
 .UNSPECIFIED.,.F.,.F.,(4,2,2,2,2,2,2,2,2,2,2,2,2,2,2,2,2,2,2,2,2,2,2,2,
2,2,2,2,2,2,2,2,2,2,2,2,2,2,2,2,2,2,2,2,2,2,2,2,2,4),(-2.93406320703471,
-2.87143399520746,-2.80165066855307,-2.78957633910132,-2.71955698375995,
-2.66455054203141,-2.64104511916306,-2.58128673311468,-2.54612054414229,
-2.49425519550508,-2.41918658143175,-2.35194063334941,-2.29048684232513,
-2.24665291139098,-2.15736466716485,-2.09112088683949,-2.03465266774453,
-1.99431292889813,-1.89898389290717,-1.83330110908048,-1.77821193978767,
-1.73874744368731,-1.64171364265346,-1.57537757862754,-1.51806752718927,
-1.42663305972774,-1.37487191786161,-1.35054239140323,-1.31562238273091,
-1.2623809917774,-1.20733488400603,-1.13558991658024,-1.06839518968176,
-1.0068654029055,-0.962977971966592,-0.873771092672304,-0.807566317326094,
-0.751021334432702,-0.710631251450796,-0.615394224793618,-0.547614894728043,
-0.491462320766733,-0.439215915126281,-0.365393474686328,-0.31952736516029,
-0.244028081793439,-0.213798227303348,-0.122271307731145,-0.0727085983661,
-4.44326005386446E-5),.UNSPECIFIED.);
#201=B_SPLINE_CURVE_WITH_KNOTS('',3,(#9839,#9840,#9841,#9842,#9843,#9844),
 .UNSPECIFIED.,.F.,.F.,(4,1,1,4),(-60.4048973677144,-60.3626749518721,-59.8638098696252,
-59.8231584322936),.UNSPECIFIED.);
#202=B_SPLINE_CURVE_WITH_KNOTS('',3,(#9850,#9851,#9852,#9853,#9854),
 .UNSPECIFIED.,.F.,.F.,(4,1,4),(57.2764810726534,57.3694844583909,57.8582308908959),
 .UNSPECIFIED.);
#203=B_SPLINE_CURVE_WITH_KNOTS('',3,(#9855,#9856,#9857,#9858,#9859,#9860,
#9861,#9862,#9863,#9864,#9865,#9866,#9867,#9868,#9869,#9870,#9871,#9872,
#9873,#9874,#9875,#9876,#9877,#9878,#9879,#9880,#9881,#9882,#9883,#9884,
#9885,#9886,#9887,#9888,#9889,#9890,#9891,#9892,#9893,#9894,#9895,#9896,
#9897,#9898,#9899,#9900,#9901,#9902,#9903,#9904,#9905,#9906,#9907,#9908,
#9909,#9910,#9911,#9912,#9913,#9914,#9915,#9916,#9917,#9918,#9919,#9920,
#9921,#9922,#9923,#9924,#9925,#9926,#9927,#9928,#9929,#9930,#9931,#9932,
#9933,#9934,#9935,#9936,#9937,#9938,#9939,#9940,#9941,#9942,#9943,#9944,
#9945,#9946,#9947,#9948,#9949,#9950,#9951,#9952,#9953,#9954,#9955,#9956,
#9957,#9958,#9959,#9960,#9961,#9962,#9963,#9964,#9965,#9966,#9967,#9968,
#9969,#9970,#9971,#9972,#9973,#9974,#9975,#9976,#9977,#9978,#9979,#9980,
#9981,#9982,#9983,#9984,#9985,#9986,#9987,#9988,#9989,#9990,#9991,#9992,
#9993,#9994,#9995,#9996,#9997,#9998,#9999,#10000,#10001,#10002,#10003,#10004,
#10005,#10006,#10007,#10008,#10009,#10010,#10011,#10012,#10013,#10014,#10015,
#10016,#10017,#10018,#10019,#10020,#10021,#10022,#10023,#10024,#10025,#10026,
#10027,#10028,#10029,#10030,#10031,#10032,#10033,#10034,#10035,#10036,#10037,
#10038,#10039,#10040,#10041,#10042,#10043,#10044,#10045,#10046,#10047,#10048,
#10049,#10050,#10051,#10052,#10053,#10054,#10055,#10056,#10057,#10058,#10059,
#10060,#10061,#10062,#10063,#10064,#10065),.UNSPECIFIED.,.F.,.F.,(4,3,3,
3,3,3,3,3,3,3,3,3,3,3,3,3,3,3,3,3,3,3,3,3,3,3,3,3,3,3,3,3,3,3,3,3,3,3,3,
3,3,3,3,3,3,3,3,3,3,3,3,3,3,3,3,3,3,3,3,3,3,3,3,3,3,3,3,3,3,3,4),(57.8582309055934,
57.8683495406378,57.9552544117093,58.042141744008,58.1290322085361,58.2159174169424,
58.302824308488,58.3672146228846,58.4541194939581,58.5410068262592,58.6278972907892,
58.7147824991975,58.8016893907451,58.8660797051315,58.9529845762033,59.0398719085024,
59.1267623730308,59.2136475814373,59.3005544729832,59.3649447873784,59.4518496584542,
59.5387369907573,59.6256274552896,59.7125126637,59.7994195552498,59.8638098696252,
59.9507147406915,60.0376020729851,60.124492537508,60.2113777459091,60.2982846374498,
60.3626749518721,60.4495798229561,60.5364671552673,60.6233576198078,60.7102428282263,
60.7971497197841,60.861540034119,60.9484449051794,61.0353322374671,61.1222227019841,
61.2091079103795,61.2960148019144,61.3604051163659,61.4473099874394,61.53419731974,
61.6210877842698,61.7079729926777,61.7948798842248,61.8592701986127,61.9461750697315,
62.0330624020779,62.1199528666535,62.2068380751072,62.2937449666998,62.3581352808596,
62.4450401517717,62.5319274839105,62.6188179482788,62.7057031565261,62.7926100479151,
62.8570003631065,62.9439052345569,63.0307925672361,63.1176830321429,63.204568240926,
63.2914751328423,63.3558654453534,63.4427695286802,63.5296580199759,63.5596986986593),
 .UNSPECIFIED.);
#204=B_SPLINE_CURVE_WITH_KNOTS('',3,(#10067,#10068,#10069,#10070,#10071,
#10072,#10073,#10074,#10075,#10076,#10077,#10078,#10079,#10080,#10081),
 .UNSPECIFIED.,.F.,.F.,(4,1,1,1,1,1,1,1,1,1,1,1,4),(-59.8231584322936,-59.3649447873784,
-58.8660797051315,-58.3672146228846,-57.8683495406377,-57.3694844583909,
-56.870619376144,-56.3717542938971,-55.8728892116502,-55.3740241294033,
-54.8751590471565,-54.3762939649096,-54.1217120605348),.UNSPECIFIED.);
#205=B_SPLINE_CURVE_WITH_KNOTS('',3,(#10082,#10083,#10084,#10085,#10086,
#10087,#10088,#10089,#10090,#10091,#10092,#10093,#10094,#10095,#10096,#10097,
#10098,#10099,#10100,#10101,#10102,#10103),.UNSPECIFIED.,.F.,.F.,(4,3,3,
3,3,3,3,4),(-54.1217120605348,-54.03365517902,-53.9455686638589,-53.8774288826627,
-53.7905200232061,-53.7036306829589,-53.6167399703894,-53.5400003888938),
 .UNSPECIFIED.);
#206=B_SPLINE_CURVE_WITH_KNOTS('',3,(#10109,#10110,#10111,#10112,#10113,
#10114,#10115,#10116,#10117,#10118,#10119,#10120,#10121,#10122,#10123,#10124,
#10125,#10126,#10127,#10128,#10129,#10130,#10131,#10132,#10133),
 .UNSPECIFIED.,.F.,.F.,(4,3,3,3,3,3,3,3,4),(50.9933372706279,51.0802213852619,
51.1671097576151,51.253994887845,51.3409000108923,51.3831034714283,51.4723469196116,
51.561562638303,51.5750455984138),.UNSPECIFIED.);
#207=B_SPLINE_CURVE_WITH_KNOTS('',3,(#10134,#10135,#10136,#10137,#10138,
#10139,#10140,#10141,#10142,#10143,#10144,#10145,#10146,#10147,#10148),
 .UNSPECIFIED.,.F.,.F.,(4,1,1,1,1,1,1,1,1,1,1,1,4),(51.5750455984138,51.8819685536752,
52.3808336359221,52.879698718169,53.3785638004159,53.8774288826627,54.3762939649096,
54.8751590471565,55.3740241294034,55.8728892116502,56.3717542938971,56.870619376144,
57.2764810726534),.UNSPECIFIED.);
#208=B_SPLINE_CURVE_WITH_KNOTS('',3,(#10150,#10151,#10152,#10153,#10154,
#10155,#10156,#10157,#10158,#10159,#10160,#10161,#10162,#10163,#10164,#10165,
#10166,#10167,#10168,#10169,#10170,#10171,#10172,#10173,#10174,#10175,#10176,
#10177,#10178,#10179,#10180,#10181,#10182,#10183,#10184,#10185,#10186,#10187,
#10188,#10189,#10190,#10191,#10192,#10193,#10194,#10195,#10196,#10197,#10198,
#10199,#10200,#10201,#10202,#10203,#10204,#10205,#10206,#10207,#10208,#10209,
#10210,#10211,#10212,#10213,#10214,#10215,#10216,#10217,#10218,#10219,#10220,
#10221,#10222,#10223,#10224,#10225,#10226,#10227,#10228,#10229,#10230,#10231,
#10232,#10233,#10234,#10235,#10236,#10237,#10238,#10239,#10240,#10241,#10242,
#10243,#10244,#10245,#10246,#10247,#10248,#10249,#10250,#10251,#10252,#10253,
#10254,#10255,#10256,#10257,#10258,#10259,#10260,#10261,#10262,#10263,#10264,
#10265,#10266,#10267,#10268,#10269,#10270,#10271,#10272,#10273,#10274,#10275,
#10276,#10277,#10278,#10279,#10280,#10281,#10282,#10283,#10284,#10285,#10286,
#10287,#10288,#10289,#10290,#10291,#10292,#10293,#10294,#10295,#10296,#10297,
#10298,#10299,#10300,#10301,#10302,#10303,#10304,#10305,#10306,#10307,#10308,
#10309,#10310,#10311,#10312,#10313,#10314,#10315,#10316,#10317,#10318,#10319,
#10320,#10321,#10322,#10323,#10324,#10325,#10326,#10327,#10328,#10329,#10330,
#10331,#10332,#10333,#10334,#10335,#10336,#10337,#10338,#10339,#10340,#10341,
#10342,#10343,#10344,#10345,#10346,#10347,#10348,#10349,#10350,#10351,#10352,
#10353,#10354,#10355,#10356,#10357),.UNSPECIFIED.,.F.,.F.,(4,3,3,3,3,3,
3,3,3,3,3,3,3,3,3,3,3,3,3,3,3,3,3,3,3,3,3,3,3,3,3,3,3,3,3,3,3,3,3,3,3,3,
3,3,3,3,3,3,3,3,3,3,3,3,3,3,3,3,3,3,3,3,3,3,3,3,3,3,3,4),(-53.5400003888938,
-53.4530924137426,-53.3785638004158,-53.2916589293431,-53.2047715970428,
-53.1178811325135,-53.0309959241062,-52.9440890325594,-52.879698718169,
-52.7927938470961,-52.7059065147958,-52.6190160502663,-52.5321308418588,
-52.4452239503118,-52.3808336359221,-52.2939287648492,-52.2070414325489,
-52.1201509680195,-52.0332657596117,-51.9463588680647,-51.8819685536752,
-51.7950636826023,-51.708176350302,-51.6212858857725,-51.5344006773649,
-51.4474937858178,-51.3831034714283,-51.2961986003556,-51.2093112680556,
-51.1224208035263,-51.0355355951188,-50.948628703572,-50.8842383891815,
-50.7973335181086,-50.7104461858084,-50.6235557212789,-50.5366705128713,
-50.4497636213243,-50.3853733069346,-50.2984684358617,-50.2115811035614,
-50.124690639032,-50.0378054306243,-49.9508985390773,-49.8865082246877,
-49.7996033536149,-49.7127160213146,-49.6258255567852,-49.5389403483777,
-49.4520334568307,-49.3876431424408,-49.3007382713678,-49.2138509390675,
-49.126960474538,-49.0400752661303,-48.9531683745832,-48.8887780601939,
-48.8018731891212,-48.714985856821,-48.6280953922917,-48.5412101838842,
-48.4543032923373,-48.3899129779471,-48.3030081068742,-48.216120774574,
-48.1292303100445,-48.0423451016371,-47.9554382100901,-47.8910478957002,
-47.8385267533552),.UNSPECIFIED.);
#209=B_SPLINE_CURVE_WITH_KNOTS('',3,(#10358,#10359,#10360,#10361,#10362,
#10363,#10364,#10365,#10366,#10367,#10368,#10369),.UNSPECIFIED.,.F.,.F.,
(4,2,2,2,2,4),(-6.46678606976702,-6.36974609711427,-6.35327484653255,-6.24967349408771,
-6.22280337759775,-6.16735576612806),.UNSPECIFIED.);
#210=B_SPLINE_CURVE_WITH_KNOTS('',3,(#10375,#10376,#10377,#10378,#10379),
 .UNSPECIFIED.,.F.,.F.,(4,1,4),(44.710117486282,44.897857402219,45.2918602818348),
 .UNSPECIFIED.);
#211=B_SPLINE_CURVE_WITH_KNOTS('',3,(#10380,#10381,#10382,#10383,#10384,
#10385,#10386,#10387,#10388,#10389,#10390,#10391,#10392,#10393,#10394,#10395,
#10396,#10397,#10398,#10399,#10400,#10401,#10402,#10403,#10404,#10405,#10406,
#10407,#10408,#10409,#10410,#10411,#10412,#10413,#10414,#10415,#10416,#10417,
#10418,#10419,#10420,#10421,#10422,#10423,#10424,#10425,#10426,#10427,#10428,
#10429,#10430,#10431,#10432,#10433,#10434,#10435,#10436,#10437,#10438,#10439,
#10440,#10441,#10442,#10443,#10444,#10445,#10446,#10447,#10448,#10449,#10450,
#10451,#10452,#10453,#10454,#10455,#10456,#10457,#10458,#10459,#10460,#10461,
#10462,#10463,#10464,#10465,#10466,#10467,#10468,#10469,#10470,#10471,#10472,
#10473,#10474,#10475,#10476,#10477,#10478,#10479,#10480,#10481,#10482,#10483,
#10484,#10485,#10486,#10487,#10488,#10489,#10490,#10491,#10492,#10493,#10494,
#10495,#10496,#10497,#10498,#10499,#10500,#10501,#10502,#10503,#10504,#10505,
#10506,#10507,#10508,#10509,#10510,#10511,#10512,#10513,#10514,#10515,#10516,
#10517,#10518,#10519,#10520,#10521,#10522,#10523,#10524,#10525,#10526,#10527,
#10528,#10529,#10530,#10531,#10532,#10533,#10534,#10535,#10536,#10537,#10538,
#10539,#10540,#10541,#10542,#10543,#10544,#10545,#10546,#10547,#10548,#10549,
#10550,#10551,#10552,#10553,#10554,#10555,#10556,#10557,#10558,#10559,#10560,
#10561,#10562,#10563,#10564,#10565,#10566,#10567,#10568,#10569,#10570,#10571,
#10572,#10573,#10574,#10575,#10576,#10577,#10578,#10579,#10580,#10581,#10582,
#10583,#10584,#10585,#10586,#10587,#10588,#10589,#10590),.UNSPECIFIED.,
 .F.,.F.,(4,3,3,3,3,3,3,3,3,3,3,3,3,3,3,3,3,3,3,3,3,3,3,3,3,3,3,3,3,3,3,
3,3,3,3,3,3,3,3,3,3,3,3,3,3,3,3,3,3,3,3,3,3,3,3,3,3,3,3,3,3,3,3,3,3,3,3,
3,3,3,4),(45.2918602912342,45.3839897102111,45.3967224844658,45.4836273555394,
45.5705146878403,45.6574051523704,45.7442903607789,45.8311972523266,45.8955875667127,
45.9824924377854,46.0693797700853,46.1562702346145,46.2431554430219,46.3300623345686,
46.3944526489596,46.4813575200326,46.5682448523329,46.6551353168625,46.7420205252702,
46.8289274168173,46.8933177312065,46.9802226022792,47.0671099345793,47.1540003991085,
47.240885607516,47.3277924990628,47.3921828134533,47.4790876845262,47.5659750168264,
47.6528654813558,47.7397506897635,47.8266575813105,47.8910478957002,47.9779527667731,
48.0648400990734,48.1517305636029,48.2386157720106,48.3255226635576,48.3899129779471,
48.47681784902,48.5637051813202,48.6505956458497,48.7374808542574,48.8243877458044,
48.888778060194,48.9756829312668,49.0625702635668,49.1494607280961,49.2363459365036,
49.3232528280504,49.3876431424408,49.4745480135137,49.5614353458139,49.6483258103434,
49.7352110187511,49.8221179102981,49.8865082246877,49.9734130957606,50.0603004280608,
50.1471908925903,50.234076100998,50.320982992545,50.3853733069346,50.4722781780076,
50.5591655103079,50.6460559748374,50.732941183245,50.8198480747921,50.8842383891815,
50.9711426268903,50.9933372706279),.UNSPECIFIED.);
#212=B_SPLINE_CURVE_WITH_KNOTS('',3,(#10591,#10592,#10593,#10594,#10595,
#10596,#10597,#10598,#10599,#10600,#10601,#10602,#10603,#10604,#10605,#10606,
#10607,#10608,#10609,#10610,#10611,#10612,#10613,#10614,#10615,#10616,#10617,
#10618,#10619,#10620,#10621,#10622,#10623,#10624,#10625,#10626,#10627,#10628,
#10629,#10630,#10631,#10632,#10633,#10634,#10635,#10636,#10637,#10638,#10639,
#10640,#10641,#10642,#10643,#10644,#10645,#10646,#10647,#10648,#10649,#10650,
#10651,#10652,#10653,#10654,#10655,#10656,#10657,#10658,#10659,#10660,#10661,
#10662,#10663,#10664,#10665,#10666,#10667,#10668,#10669,#10670,#10671,#10672,
#10673,#10674,#10675,#10676,#10677,#10678,#10679,#10680,#10681,#10682,#10683,
#10684,#10685,#10686,#10687,#10688,#10689,#10690,#10691,#10692,#10693,#10694,
#10695,#10696,#10697,#10698,#10699,#10700,#10701,#10702),.UNSPECIFIED.,
 .F.,.F.,(4,2,2,2,2,2,2,2,2,2,2,2,2,2,2,2,2,2,2,2,2,2,2,2,2,2,2,2,2,2,2,
2,2,2,2,2,2,2,2,2,2,2,2,2,2,2,2,2,2,2,2,2,2,2,2,4),(-6.16735576612806,-6.15921345146165,
-6.11345500378577,-6.01807848390996,-5.97776732229564,-5.92133925481309,
-5.85507237955178,-5.76574269662213,-5.72193933189343,-5.66052737580998,
-5.59325028222066,-5.51873451616644,-5.46743249191829,-5.41027892343107,
-5.34388007609257,-5.24667547941811,-5.20730073602016,-5.15235443733306,
-5.0866278090815,-4.99107975420786,-4.95085991288905,-4.89457189350567,
-4.82967302269615,-4.73488188081266,-4.69426163275514,-4.63736534206582,
-4.57134972752306,-4.48254497888756,-4.43840929496829,-4.37651978835189,
-4.30958035640124,-4.23801488265242,-4.18284695730065,-4.12965507624722,
-4.09471677844922,-4.07038370453636,-4.01862976067098,-3.92717495748881,
-3.86986731003032,-3.8033950930707,-3.70182512452207,-3.66560106131781,
-3.60357428245561,-3.53882169825608,-3.45805550073204,-3.41189659075085,
-3.36164150274549,-3.30921114318311,-3.28606788502557,-3.23338728280752,
-3.17281530728171,-3.1431045953554,-3.07197166944413,-3.01772333034713,
-2.99411202495098,-2.93408130173726),.UNSPECIFIED.);
#213=B_SPLINE_CURVE_WITH_KNOTS('',3,(#10708,#10709,#10710,#10711,#10712,
#10713,#10714,#10715,#10716,#10717,#10718,#10719),.UNSPECIFIED.,.F.,.F.,
(4,2,2,2,2,4),(-0.29941706624709,-0.272624008446249,-0.193071594358554,
-0.14393047447416,-0.0491105809088329,-4.41492292512854E-5),
 .UNSPECIFIED.);
#214=B_SPLINE_CURVE_WITH_KNOTS('',3,(#10720,#10721,#10722,#10723,#10724,
#10725,#10726,#10727,#10728,#10729,#10730,#10731,#10732,#10733,#10734),
 .UNSPECIFIED.,.F.,.F.,(4,1,1,1,1,1,1,1,1,1,1,1,4),(39.0086749840546,39.4103414975033,
39.9092065797502,40.4080716619971,40.9069367442439,41.4058018264908,41.9046669087377,
42.4035319909846,42.9023970732314,43.4012621554783,43.9001272377252,44.3989923199721,
44.710117486282),.UNSPECIFIED.);
#215=B_SPLINE_CURVE_WITH_KNOTS('',3,(#10736,#10737,#10738,#10739,#10740,
#10741,#10742,#10743,#10744,#10745,#10746,#10747,#10748,#10749,#10750,#10751,
#10752,#10753,#10754,#10755,#10756,#10757,#10758,#10759,#10760,#10761,#10762,
#10763,#10764,#10765,#10766,#10767,#10768,#10769,#10770,#10771,#10772,#10773,
#10774,#10775,#10776,#10777,#10778,#10779,#10780,#10781,#10782,#10783,#10784,
#10785,#10786,#10787,#10788,#10789,#10790,#10791,#10792,#10793,#10794,#10795,
#10796,#10797,#10798,#10799,#10800,#10801,#10802,#10803,#10804,#10805,#10806,
#10807,#10808,#10809,#10810,#10811,#10812,#10813,#10814,#10815,#10816,#10817,
#10818,#10819,#10820,#10821,#10822,#10823,#10824,#10825,#10826,#10827,#10828,
#10829,#10830,#10831,#10832,#10833,#10834,#10835,#10836,#10837),
 .UNSPECIFIED.,.F.,.F.,(4,2,2,2,2,2,2,2,2,2,2,2,2,2,2,2,2,2,2,2,2,2,2,2,
2,2,2,2,2,2,2,2,2,2,2,2,2,2,2,2,2,2,2,2,2,2,2,2,2,2,4),(-2.93408130173726,
-2.93304885547358,-2.91194674280188,-2.88204922197342,-2.84302030640522,
-2.77352700671621,-2.70675002102001,-2.64463095528211,-2.60033769366457,
-2.51176973473058,-2.44586660880208,-2.38876135407395,-2.34799899037949,
-2.25346425894163,-2.18361280540833,-2.12995714258924,-2.03336695858138,
-1.98251129590212,-1.88096958966132,-1.84930159101389,-1.80041718264956,
-1.74516693890976,-1.67541237326298,-1.6186224109205,-1.57807059358303,
-1.48313964198103,-1.4134917643136,-1.3597162357856,-1.30826755598738,-1.23305628927718,
-1.16582344893134,-1.10434789521201,-1.06049846430573,-0.971231602678871,
-0.904997802848148,-0.848507296731753,-0.808152960198933,-0.712848230441378,
-0.646904496746172,-0.592135568633003,-0.552865968410389,-0.45543675033151,
-0.388883997280267,-0.332023636198457,-0.308123738779688,-0.257508419796942,
-0.198789885410597,-0.152986897520325,-0.0793248458577054,-0.0663949178379873,
-4.4182641542272E-5),.UNSPECIFIED.);
#216=B_SPLINE_CURVE_WITH_KNOTS('',3,(#10838,#10839,#10840,#10841,#10842),
 .UNSPECIFIED.,.F.,.F.,(4,1,4),(-35.272156138996,-34.9205557572814,-34.690424885304),
 .UNSPECIFIED.);
#217=B_SPLINE_CURVE_WITH_KNOTS('',3,(#10847,#10848,#10849,#10850,#10851,
#10852,#10853,#10854,#10855,#10856,#10857,#10858,#10859,#10860,#10861,#10862,
#10863,#10864,#10865,#10866,#10867,#10868,#10869,#10870,#10871,#10872,#10873,
#10874,#10875,#10876,#10877,#10878,#10879,#10880,#10881,#10882,#10883,#10884,
#10885,#10886,#10887,#10888,#10889,#10890,#10891,#10892,#10893,#10894,#10895,
#10896,#10897,#10898,#10899,#10900,#10901,#10902,#10903,#10904,#10905,#10906,
#10907,#10908,#10909,#10910,#10911,#10912,#10913,#10914,#10915,#10916,#10917,
#10918,#10919,#10920,#10921,#10922,#10923,#10924,#10925,#10926,#10927,#10928,
#10929,#10930,#10931,#10932,#10933,#10934,#10935,#10936,#10937,#10938,#10939,
#10940,#10941,#10942,#10943,#10944,#10945,#10946,#10947,#10948,#10949,#10950,
#10951,#10952,#10953,#10954,#10955,#10956,#10957,#10958,#10959,#10960,#10961,
#10962,#10963,#10964),.UNSPECIFIED.,.F.,.F.,(4,2,2,2,2,2,2,2,2,2,2,2,2,
2,2,2,2,2,2,2,2,2,2,2,2,2,2,2,2,2,2,2,2,2,2,2,2,2,2,2,2,2,2,2,2,2,2,2,2,
2,2,2,2,2,2,2,2,2,4),(-3.53273226990805,-3.51217029370589,-3.43143246081615,
-3.38602691469201,-3.33619900388063,-3.2836417674659,-3.2333912848074,-3.18011428936759,
-3.13269368376827,-3.09047605886201,-2.99852804850881,-2.93085259017726,
-2.8733208960313,-2.86123265038794,-2.79119116778289,-2.7362228838575,-2.71271252262557,
-2.65289371301879,-2.6270334813131,-2.59632911246521,-2.55229814685202,
-2.49081566908837,-2.42306295857898,-2.36232675411795,-2.31900273175731,
-2.22889487345454,-2.16223976266328,-2.10653972026565,-2.06669457195355,
-1.97040951439539,-1.90341780941698,-1.84665279589094,-1.79446397924416,
-1.72073312461513,-1.65346107052155,-1.59203976036453,-1.54822866909107,
-1.4588996007104,-1.39263551281092,-1.33620007127111,-1.2958819143125,-1.20050681071984,
-1.17730395962771,-1.12221644598454,-1.07691779399216,-0.985679253607082,
-0.933714695344074,-0.909482207307218,-0.875100002972594,-0.820236697278058,
-0.768907984868682,-0.693855037781347,-0.62660630905221,-0.565153519541634,
-0.521320313654361,-0.432027958888678,-0.365781987637995,-0.309414102241624,
-0.29941706624709),.UNSPECIFIED.);
#218=B_SPLINE_CURVE_WITH_KNOTS('',3,(#10966,#10967,#10968,#10969,#10970,
#10971,#10972,#10973,#10974,#10975,#10976,#10977,#10978,#10979,#10980),
 .UNSPECIFIED.,.F.,.F.,(4,1,1,1,1,1,1,1,1,1,1,1,4),(-34.690424885304,-34.4216906750345,
-33.9228255927876,-33.4239605105408,-32.9250954282939,-32.426230346047,
-31.9273652638001,-31.4285001815533,-30.9296350993064,-30.4307700170595,
-29.9319049348126,-29.4330398525657,-28.9889708747585),.UNSPECIFIED.);
#219=B_SPLINE_CURVE_WITH_KNOTS('',3,(#10981,#10982,#10983,#10984,#10985,
#10986,#10987,#10988,#10989,#10990,#10991,#10992,#10993,#10994,#10995,#10996,
#10997,#10998,#10999,#11000,#11001,#11002,#11003,#11004,#11005),
 .UNSPECIFIED.,.F.,.F.,(4,3,3,3,3,3,3,3,4),(-28.9889708318164,-28.9341747703189,
-28.8472698992443,-28.7603825669425,-28.6734921024112,-28.5866068940016,
-28.4997000024527,-28.435309688072,-28.4072371742117),.UNSPECIFIED.);
#220=B_SPLINE_CURVE_WITH_KNOTS('',3,(#11011,#11012,#11013,#11014,#11015,
#11016,#11017,#11018,#11019,#11020,#11021,#11022,#11023,#11024),
 .UNSPECIFIED.,.F.,.F.,(4,2,2,2,2,2,4),(-0.299389883818606,-0.261813445457985,
-0.235776114650808,-0.189442449010928,-0.130882530543728,-0.0850842402352701,
-4.4159677240208E-5),.UNSPECIFIED.);
#221=B_SPLINE_CURVE_WITH_KNOTS('',3,(#11025,#11026,#11027,#11028,#11029,
#11030,#11031,#11032,#11033,#11034,#11035,#11036,#11037,#11038,#11039,#11040,
#11041,#11042,#11043,#11044,#11045,#11046,#11047,#11048,#11049,#11050,#11051,
#11052,#11053,#11054,#11055,#11056,#11057,#11058,#11059,#11060,#11061,#11062,
#11063,#11064,#11065,#11066,#11067,#11068,#11069,#11070,#11071,#11072,#11073,
#11074,#11075,#11076,#11077,#11078,#11079,#11080,#11081,#11082,#11083,#11084,
#11085,#11086,#11087,#11088,#11089,#11090,#11091,#11092,#11093,#11094,#11095,
#11096,#11097,#11098,#11099,#11100,#11101,#11102,#11103,#11104,#11105,#11106,
#11107,#11108,#11109,#11110,#11111,#11112,#11113,#11114,#11115,#11116,#11117,
#11118,#11119,#11120,#11121,#11122,#11123,#11124),.UNSPECIFIED.,.F.,.F.,
(4,2,2,2,2,2,2,2,2,2,2,2,2,2,2,2,2,2,2,2,2,2,2,2,2,2,2,2,2,2,2,2,2,2,2,
2,2,2,2,2,2,2,2,2,2,2,2,2,2,4),(-6.46680925296249,-6.38442007318614,-6.33863123016491,
-6.28248089476868,-6.23448359497408,-6.21006599349175,-6.14608635288184,
-6.09823123559437,-6.04639873864054,-5.95477998639039,-5.90909496631497,
-5.85413175757243,-5.83093420372116,-5.73604918032842,-5.69547435977023,
-5.63864626091275,-5.57258925836412,-5.48369869485737,-5.43961270500058,
-5.37779513039796,-5.31079934616192,-5.23445340596768,-5.18506973985015,
-5.12779019417545,-5.0612833673779,-4.96469937036644,-4.9250099182995,-4.86955389952252,
-4.80413015425949,-4.70888429015701,-4.67968108286381,-4.64838581031007,
-4.55174482168042,-4.49656510528779,-4.42664142849673,-4.41462808513177,
-4.3583027779773,-4.29069171816555,-4.19532338116545,-4.15500509298302,
-4.09856603006887,-4.03230201601623,-3.94297927638577,-3.89916840051344,
-3.83774544887639,-3.77047264300654,-3.6957926407437,-3.64557402910458,
-3.57459764904799,-3.53273226990805),.UNSPECIFIED.);
#222=B_SPLINE_CURVE_WITH_KNOTS('',3,(#11126,#11127,#11128,#11129,#11130,
#11131,#11132,#11133,#11134,#11135,#11136,#11137,#11138,#11139,#11140,#11141,
#11142,#11143,#11144,#11145,#11146,#11147,#11148,#11149,#11150,#11151,#11152,
#11153,#11154,#11155,#11156,#11157,#11158,#11159,#11160,#11161,#11162,#11163,
#11164,#11165,#11166,#11167,#11168,#11169,#11170,#11171,#11172,#11173,#11174,
#11175,#11176,#11177,#11178,#11179,#11180,#11181,#11182,#11183,#11184,#11185,
#11186,#11187,#11188,#11189,#11190,#11191,#11192,#11193,#11194,#11195,#11196,
#11197,#11198,#11199,#11200,#11201,#11202,#11203,#11204,#11205,#11206,#11207,
#11208,#11209,#11210,#11211,#11212,#11213,#11214,#11215,#11216,#11217,#11218,
#11219,#11220,#11221,#11222,#11223,#11224,#11225,#11226,#11227,#11228,#11229,
#11230,#11231,#11232,#11233,#11234,#11235,#11236,#11237,#11238,#11239,#11240,
#11241,#11242,#11243,#11244,#11245,#11246,#11247,#11248,#11249,#11250,#11251,
#11252,#11253,#11254,#11255,#11256,#11257,#11258,#11259,#11260,#11261,#11262,
#11263,#11264,#11265,#11266,#11267,#11268,#11269,#11270,#11271,#11272,#11273,
#11274,#11275,#11276,#11277,#11278,#11279,#11280,#11281,#11282,#11283,#11284,
#11285,#11286,#11287,#11288,#11289,#11290,#11291,#11292,#11293,#11294,#11295,
#11296,#11297,#11298,#11299,#11300,#11301,#11302,#11303,#11304,#11305,#11306,
#11307,#11308,#11309,#11310,#11311,#11312,#11313,#11314,#11315,#11316,#11317,
#11318,#11319,#11320,#11321,#11322,#11323,#11324,#11325,#11326,#11327,#11328,
#11329,#11330,#11331,#11332,#11333),.UNSPECIFIED.,.F.,.F.,(4,3,3,3,3,3,
3,3,3,3,3,3,3,3,3,3,3,3,3,3,3,3,3,3,3,3,3,3,3,3,3,3,3,3,3,3,3,3,3,3,3,3,
3,3,3,3,3,3,3,3,3,3,3,3,3,3,3,3,3,3,3,3,3,3,3,3,3,3,3,4),(-28.4072371742117,
-28.3203388291425,-28.23345547998,-28.1465675751263,-28.0596823795464,-27.9727775859982,
-27.9364446058251,-27.849539734752,-27.7626524024515,-27.6757619379218,
-27.5888767295139,-27.5019698379666,-27.4375795235782,-27.3506746525055,
-27.2637873202054,-27.1768968556761,-27.0900116472686,-27.0031047557218,
-26.9387144413314,-26.8518095702586,-26.7649222379583,-26.6780317734289,
-26.5911465650213,-26.5042396734743,-26.4398493590845,-26.3529444880116,
-26.2660571557112,-26.1791666911817,-26.0922814827741,-26.005374591227,
-25.9409842768376,-25.8540794057648,-25.7671920734646,-25.6803016089352,
-25.5934164005277,-25.5065095089807,-25.4421191945907,-25.3552143235177,
-25.2683269912175,-25.181436526688,-25.0945513182803,-25.0076444267333,
-24.9432541123438,-24.8563492412711,-24.7694619089709,-24.6825714444416,
-24.5956862360341,-24.5087793444873,-24.444389030097,-24.3574841590241,
-24.2705968267238,-24.1837063621944,-24.0968211537868,-24.0099142622398,
-23.9455239478501,-23.8586190767772,-23.771731744477,-23.6848412799475,
-23.5979560715399,-23.5110491799929,-23.4466588656032,-23.3597539945303,
-23.2728666622302,-23.1859761977007,-23.0990909892933,-23.0121840977463,
-22.9477937833563,-22.8596658861628,-22.7715576075161,-22.7057855246368),
 .UNSPECIFIED.);
#223=B_SPLINE_CURVE_WITH_KNOTS('',3,(#11334,#11335,#11336,#11337,#11338,
#11339,#11340,#11341,#11342,#11343,#11344,#11345),.UNSPECIFIED.,.F.,.F.,
(4,2,2,2,2,4),(-6.46682447949202,-6.36050996356338,-6.3360943075336,-6.25630149105725,
-6.21056945448505,-6.16740264682167),.UNSPECIFIED.);
#224=B_SPLINE_CURVE_WITH_KNOTS('',3,(#11350,#11351,#11352,#11353,#11354,
#11355,#11356,#11357,#11358,#11359,#11360,#11361,#11362,#11363,#11364,#11365,
#11366,#11367,#11368,#11369,#11370,#11371,#11372,#11373,#11374,#11375,#11376,
#11377,#11378,#11379,#11380,#11381,#11382,#11383,#11384,#11385,#11386,#11387,
#11388,#11389,#11390,#11391,#11392,#11393,#11394,#11395,#11396,#11397,#11398,
#11399,#11400,#11401,#11402,#11403,#11404,#11405,#11406,#11407,#11408,#11409,
#11410,#11411,#11412,#11413,#11414,#11415,#11416,#11417,#11418,#11419,#11420,
#11421,#11422,#11423,#11424,#11425,#11426,#11427,#11428,#11429,#11430,#11431,
#11432,#11433,#11434,#11435,#11436,#11437,#11438,#11439,#11440,#11441,#11442,
#11443,#11444,#11445,#11446,#11447,#11448,#11449,#11450,#11451,#11452,#11453,
#11454,#11455,#11456,#11457,#11458,#11459,#11460,#11461,#11462,#11463),
 .UNSPECIFIED.,.F.,.F.,(4,2,2,2,2,2,2,2,2,2,2,2,2,2,2,2,2,2,2,2,2,2,2,2,
2,2,2,2,2,2,2,2,2,2,2,2,2,2,2,2,2,2,2,2,2,2,2,2,2,2,2,2,2,2,2,2,4),(-3.53204766679888,
-3.49982421516289,-3.47626775403068,-3.42173140785212,-3.36502956813804,
-3.34916018500265,-3.31900175765622,-3.25903249160735,-3.23286461982597,
-3.18258127700049,-3.12816194346365,-3.0808734759152,-2.9894913208945,-2.93774632455422,
-2.9134283703324,-2.8785335070882,-2.82527828015015,-2.77339179940797,-2.6985322974546,
-2.63129804283183,-2.56988945816759,-2.5260875802445,-2.43681108506132,
-2.37058223526934,-2.31415718165661,-2.27384726176553,-2.17852929410056,
-2.11277006943221,-2.05784330744651,-2.01848056986588,-1.92131214425873,
-1.85494144458653,-1.79780691309944,-1.7437811615371,-1.67161461307685,
-1.60238749597071,-1.54374644484518,-1.5019238525573,-1.40929374630339,
-1.34120370799465,-1.28446321322327,-1.23364780099984,-1.15854616594712,
-1.09130309820798,-1.02984437445668,-0.986007010959373,-0.896723369940915,
-0.830481941090336,-0.774008379874504,-0.733665362334244,-0.638341651544923,
-0.572859401100843,-0.517511704800658,-0.477887577999317,-0.382128516453115,
-0.313437902341981,-0.299389883818606),.UNSPECIFIED.);
#225=B_SPLINE_CURVE_WITH_KNOTS('',3,(#11464,#11465,#11466,#11467,#11468,
#11469,#11470,#11471,#11472,#11473,#11474,#11475,#11476,#11477,#11478,#11479,
#11480,#11481,#11482,#11483,#11484,#11485,#11486,#11487,#11488,#11489,#11490,
#11491,#11492,#11493,#11494,#11495,#11496,#11497,#11498,#11499,#11500,#11501,
#11502,#11503,#11504,#11505,#11506,#11507,#11508,#11509,#11510,#11511,#11512,
#11513,#11514,#11515,#11516,#11517,#11518,#11519,#11520,#11521,#11522,#11523,
#11524,#11525,#11526,#11527,#11528,#11529,#11530,#11531,#11532,#11533,#11534,
#11535,#11536,#11537,#11538,#11539,#11540,#11541,#11542,#11543,#11544,#11545,
#11546,#11547,#11548,#11549,#11550,#11551,#11552,#11553,#11554,#11555,#11556,
#11557,#11558,#11559,#11560,#11561,#11562,#11563,#11564,#11565,#11566,#11567,
#11568,#11569,#11570,#11571,#11572,#11573,#11574,#11575,#11576,#11577,#11578,
#11579),.UNSPECIFIED.,.F.,.F.,(4,2,2,2,2,2,2,2,2,2,2,2,2,2,2,2,2,2,2,2,
2,2,2,2,2,2,2,2,2,2,2,2,2,2,2,2,2,2,2,2,2,2,2,2,2,2,2,2,2,2,2,2,2,2,2,2,
2,4),(-6.16740264682167,-6.11563365794476,-6.07532444593123,-6.0188994362692,
-5.9526295528832,-5.86329436872957,-5.81949304354482,-5.75808399690235,
-5.69080327778159,-5.61641055390375,-5.56442438541974,-5.50967749272918,
-5.43531913424907,-5.37797403236362,-5.31542697489267,-5.28344297801199,
-5.187491173287,-5.13146699607826,-5.05785111294859,-5.02512521307028,-4.96672822773466,
-4.94166264026503,-4.89085619430738,-4.79412421453088,-4.73988129353064,
-4.67071491794505,-4.57533420650859,-4.53502488775429,-4.47859966065171,
-4.41233088639287,-4.32299749628851,-4.27919607150013,-4.21778687492078,
-4.15050739988328,-4.07645024969687,-4.02442447301068,-3.95504297002624,
-3.90807117489429,-3.85496196358606,-3.78258372534596,-3.76997422021965,
-3.73282142537731,-3.67247481912233,-3.6489218695235,-3.59427629725168,
-3.524052896448,-3.51184750374542,-3.44139495257376,-3.3944774964091,-3.34125289840925,
-3.26408027613105,-3.2335036593988,-3.19016415151798,-3.12768137039442,
-3.06040030541999,-2.99899320386999,-2.95519186805188,-2.93416253856114),
 .UNSPECIFIED.);
#226=B_SPLINE_CURVE_WITH_KNOTS('',3,(#11585,#11586,#11587,#11588,#11589,
#11590,#11591,#11592,#11593,#11594,#11595,#11596,#11597,#11598),
 .UNSPECIFIED.,.F.,.F.,(4,2,2,2,2,2,4),(-0.299449727543266,-0.287141748908116,
-0.223493924177034,-0.196628569872181,-0.0910589500302473,-0.0595876231948999,
-4.44166853382205E-5),.UNSPECIFIED.);
#227=B_SPLINE_CURVE_WITH_KNOTS('',3,(#11599,#11600,#11601,#11602,#11603,
#11604,#11605,#11606,#11607,#11608,#11609,#11610,#11611,#11612,#11613,#11614,
#11615,#11616,#11617,#11618,#11619,#11620,#11621,#11622,#11623,#11624,#11625,
#11626,#11627,#11628,#11629,#11630,#11631,#11632,#11633,#11634,#11635,#11636,
#11637,#11638,#11639,#11640,#11641,#11642,#11643,#11644,#11645,#11646,#11647,
#11648,#11649,#11650,#11651,#11652,#11653,#11654,#11655,#11656,#11657,#11658,
#11659,#11660,#11661,#11662,#11663,#11664,#11665,#11666,#11667,#11668,#11669,
#11670,#11671,#11672,#11673,#11674,#11675,#11676,#11677,#11678,#11679,#11680,
#11681,#11682,#11683,#11684,#11685,#11686,#11687,#11688,#11689,#11690,#11691,
#11692,#11693,#11694,#11695,#11696,#11697,#11698,#11699,#11700),
 .UNSPECIFIED.,.F.,.F.,(4,2,2,2,2,2,2,2,2,2,2,2,2,2,2,2,2,2,2,2,2,2,2,2,
2,2,2,2,2,2,2,2,2,2,2,2,2,2,2,2,2,2,2,2,2,2,2,2,2,2,4),(-6.46489889827727,
-6.41872330513384,-6.37412377088042,-6.29277358877099,-6.23367193274467,
-6.18453002104199,-6.16086699093738,-6.1070859069055,-6.07222718892308,
-6.04791497663975,-5.99615591714179,-5.90471723431846,-5.84788220120214,
-5.78135088156293,-5.68395911282417,-5.64470746758329,-5.5899603318361,
-5.52401238712714,-5.42883390716834,-5.38845088473501,-5.33191111691408,
-5.26573841136418,-5.17658551816971,-5.132706347603,-5.07118567603099,-5.00402471070972,
-4.92852970160446,-4.87769643036357,-4.82291086896213,-4.7551299024827,
-4.65684710934992,-4.6180311171497,-4.56401881018412,-4.4975433648843,-4.40222212718805,
-4.3619159629023,-4.30549331372222,-4.23925984243533,-4.14998075341933,
-4.10618318176873,-4.04477879324171,-3.97753798197369,-3.9028000877843,
-3.85143748823915,-3.78217319085083,-3.73521456109145,-3.68213522868841,
-3.6097860585557,-3.59717469579274,-3.5603009501235,-3.53204766679888),
 .UNSPECIFIED.);
#228=B_SPLINE_CURVE_WITH_KNOTS('',3,(#11702,#11703,#11704,#11705,#11706,
#11707,#11708,#11709,#11710,#11711,#11712,#11713,#11714,#11715,#11716,#11717,
#11718,#11719,#11720,#11721,#11722,#11723,#11724,#11725,#11726,#11727,#11728,
#11729,#11730,#11731,#11732,#11733,#11734,#11735,#11736,#11737,#11738,#11739,
#11740,#11741,#11742,#11743,#11744,#11745,#11746,#11747,#11748,#11749,#11750,
#11751,#11752,#11753,#11754,#11755,#11756,#11757,#11758,#11759,#11760,#11761,
#11762,#11763,#11764,#11765,#11766,#11767,#11768,#11769,#11770,#11771,#11772,
#11773,#11774,#11775,#11776,#11777,#11778,#11779,#11780,#11781,#11782,#11783,
#11784,#11785,#11786,#11787,#11788,#11789,#11790,#11791,#11792,#11793,#11794,
#11795,#11796,#11797,#11798,#11799),.UNSPECIFIED.,.F.,.F.,(4,2,2,2,2,2,
2,2,2,2,2,2,2,2,2,2,2,2,2,2,2,2,2,2,2,2,2,2,2,2,2,2,2,2,2,2,2,2,2,2,2,2,
2,2,2,2,2,2,4),(-2.93416253856114,-2.8658487605409,-2.7995778425485,-2.74315680984522,
-2.70284793186746,-2.60745671480959,-2.58425385749397,-2.52916228410746,
-2.48271237418502,-2.43431203632113,-2.35897151295802,-2.29623441308256,
-2.22702425643058,-2.2150594067632,-2.14520695210958,-2.08988541840876,
-2.03740229931192,-1.97158151274785,-1.9243935139356,-1.84252085959546,
-1.77221502501627,-1.71643224860532,-1.67653453813169,-1.58035272865833,
-1.51310228342344,-1.45663670399648,-1.40556004367395,-1.33064675499336,
-1.26338555679267,-1.20194942495713,-1.15812767395307,-1.0688161119025,
-1.00256045821056,-0.946109900161033,-0.905781699015191,-0.810426361879754,
-0.744510427396677,-0.689724658717433,-0.650444847521016,-0.553035219322984,
-0.486499385581561,-0.429607216311699,-0.37861337124737,-0.301545345367292,
-0.255833865889075,-0.176908182396489,-0.151053254639042,-0.0538737242154548,
-4.41474414227578E-5),.UNSPECIFIED.);
#229=B_SPLINE_CURVE_WITH_KNOTS('',3,(#11800,#11801,#11802,#11803,#11804),
 .UNSPECIFIED.,.F.,.F.,(4,1,4),(-10.1394149102777,-9.97730164493754,-9.55771221567013),
 .UNSPECIFIED.);
#230=B_SPLINE_CURVE_WITH_KNOTS('',3,(#11810,#11811,#11812,#11813,#11814,
#11815,#11816,#11817,#11818,#11819,#11820,#11821,#11822,#11823,#11824,#11825,
#11826,#11827,#11828,#11829,#11830,#11831,#11832,#11833,#11834,#11835,#11836,
#11837,#11838,#11839,#11840,#11841,#11842,#11843,#11844,#11845,#11846,#11847,
#11848,#11849,#11850,#11851,#11852,#11853,#11854,#11855,#11856,#11857,#11858,
#11859,#11860,#11861,#11862,#11863,#11864,#11865,#11866,#11867,#11868,#11869,
#11870,#11871,#11872,#11873,#11874,#11875,#11876,#11877,#11878,#11879,#11880,
#11881,#11882,#11883,#11884,#11885,#11886,#11887,#11888,#11889,#11890,#11891,
#11892,#11893,#11894,#11895,#11896,#11897,#11898,#11899,#11900,#11901,#11902,
#11903,#11904,#11905,#11906,#11907,#11908,#11909,#11910,#11911,#11912,#11913,
#11914,#11915,#11916,#11917,#11918,#11919,#11920,#11921,#11922,#11923,#11924,
#11925,#11926,#11927,#11928,#11929,#11930),.UNSPECIFIED.,.F.,.F.,(4,3,3,
3,3,3,3,3,3,3,3,3,3,3,3,3,3,3,3,3,3,3,3,3,3,3,3,3,3,3,3,3,3,3,3,3,3,3,3,
3,4),(-3.27449886892727,-3.18761614376122,-3.10073466380896,-3.01383445139677,
-2.99319049348126,-2.90628637831284,-2.81939983534294,-2.73251020278055,
-2.64562584817912,-2.55871983698197,-2.49432541123439,-2.40740187823325,
-2.32049576623348,-2.23358652858203,-2.14668259333812,-2.05975722263729,
-1.99546032898751,-1.90861705921206,-1.82179160018738,-1.73496281748211,
-1.64813904686475,-1.56129263759828,-1.49659524674063,-1.409546118953,-1.32251404603999,
-1.23547955077808,-1.14845104380955,-1.06140335733105,-0.997730164493756,
-0.911094995373688,-0.824477714185506,-0.737855241080792,-0.651236305870609,
-0.564590515016393,-0.498865082246876,-0.411426010329821,-0.324005451184797,
-0.23658882318787,-0.149182757533382,-0.0617684476840146,0.),
 .UNSPECIFIED.);
#231=B_SPLINE_CURVE_WITH_KNOTS('',3,(#11933,#11934,#11935,#11936,#11937,
#11938,#11939,#11940,#11941,#11942,#11943,#11944,#11945,#11946,#11947,#11948,
#11949,#11950,#11951,#11952,#11953,#11954,#11955,#11956,#11957,#11958,#11959,
#11960,#11961,#11962,#11963,#11964,#11965,#11966,#11967,#11968,#11969,#11970,
#11971,#11972,#11973,#11974,#11975,#11976,#11977,#11978,#11979,#11980,#11981,
#11982,#11983,#11984,#11985,#11986,#11987,#11988,#11989,#11990,#11991,#11992,
#11993,#11994,#11995,#11996,#11997,#11998,#11999,#12000,#12001,#12002,#12003,
#12004,#12005,#12006,#12007,#12008,#12009,#12010,#12011,#12012,#12013,#12014,
#12015,#12016,#12017,#12018),.UNSPECIFIED.,.F.,.F.,(4,2,2,2,2,2,2,2,2,2,
2,2,2,2,2,2,2,2,2,2,2,2,2,2,2,2,2,2,2,2,2,2,2,2,2,2,2,2,2,2,2,2,4),(-6.09872156040909,
-6.00749427805286,-5.95742926200475,-5.8822861453486,-5.85809857342036,
-5.78022624038386,-5.73447496159819,-5.63655125552659,-5.59754757665871,
-5.54254594849079,-5.47675567134605,-5.38173848350033,-5.34123963860053,
-5.2847878351896,-5.21852565229132,-5.12920756671915,-5.085388588857,-5.023881617872,
-4.95667908611682,-4.88197222379136,-4.82990297021068,-4.77657904741458,
-4.7416829481717,-4.7173559230713,-4.66557707226733,-4.57412938940594,-4.517139405479,
-4.45003936488945,-4.35464382778697,-4.31434369371454,-4.25790859518146,
-4.19164432464583,-4.10233620771383,-4.05851850179046,-3.99710349847546,
-3.92982829922061,-3.85557626231805,-3.80332580353464,-3.74888562478497,
-3.67415716796871,-3.61620401672537,-3.55429967198194,-3.53290494255096),
 .UNSPECIFIED.);
#232=B_SPLINE_CURVE_WITH_KNOTS('',3,(#12020,#12021,#12022,#12023,#12024,
#12025,#12026,#12027,#12028,#12029,#12030,#12031,#12032,#12033,#12034,#12035,
#12036,#12037,#12038,#12039,#12040,#12041,#12042,#12043,#12044,#12045,#12046,
#12047,#12048,#12049,#12050,#12051,#12052,#12053,#12054,#12055,#12056,#12057,
#12058,#12059,#12060,#12061,#12062,#12063,#12064,#12065,#12066,#12067,#12068,
#12069,#12070,#12071,#12072,#12073,#12074,#12075,#12076,#12077,#12078,#12079,
#12080,#12081,#12082,#12083,#12084,#12085,#12086,#12087,#12088,#12089,#12090,
#12091,#12092,#12093,#12094,#12095,#12096,#12097,#12098,#12099,#12100,#12101,
#12102,#12103,#12104,#12105,#12106,#12107,#12108,#12109,#12110,#12111,#12112,
#12113,#12114,#12115,#12116,#12117,#12118,#12119,#12120,#12121,#12122,#12123,
#12124,#12125,#12126,#12127,#12128,#12129,#12130,#12131),.UNSPECIFIED.,
 .F.,.F.,(4,2,2,2,2,2,2,2,2,2,2,2,2,2,2,2,2,2,2,2,2,2,2,2,2,2,2,2,2,2,2,
2,2,2,2,2,2,2,2,2,2,2,2,2,2,2,2,2,2,2,2,2,2,2,2,4),(-3.53290494255096,-3.52220028737842,
-3.42634731206105,-3.37017838496927,-3.29839478213502,-3.26691402455281,
-3.20007373282,-3.17593663231303,-3.12374653463165,-3.04965357055732,-3.01994343430044,
-2.94881420189061,-2.89456737670883,-2.87095448036624,-2.80988148046529,
-2.78713854085941,-2.75675827729302,-2.71452852641755,-2.65036372662648,
-2.58355717107225,-2.52147302895015,-2.47720377226936,-2.3885914938337,
-2.32266697315307,-2.26559363389747,-2.22485270583054,-2.13027050849742,
-2.06329937440856,-2.00582007712969,-1.95319927659059,-1.88007976087321,
-1.81284777182449,-1.75136827054773,-1.70751629794579,-1.61825068119185,
-1.55201726258365,-1.49552289407734,-1.45516613459724,-1.35986300161468,
-1.29371280701194,-1.23920424216273,-1.20009091465415,-1.10234083242336,
-1.03544008499539,-0.97917424594622,-0.926655501305632,-0.853133409595351,
-0.78587124449319,-0.72443292852784,-0.680609872629603,-0.591296775173454,
-0.525040040584877,-0.468587421209888,-0.428257965622739,-0.332901112037465,
-0.299449727543266),.UNSPECIFIED.);
#233=B_SPLINE_CURVE_WITH_KNOTS('',3,(#12133,#12134,#12135,#12136,#12137,
#12138,#12139,#12140,#12141,#12142,#12143,#12144,#12145,#12146,#12147,#12148),
 .UNSPECIFIED.,.F.,.F.,(4,1,1,1,1,1,1,1,1,1,1,1,1,4),(-9.55771221567013,
-9.47843656269067,-8.97957148044379,-8.48070639819691,-7.98184131595003,
-7.48297623370316,-6.98411115145628,-6.4852460692094,-5.98638098696252,
-5.48751590471565,-4.98865082246877,-4.48978574022189,-3.99092065797502,
-3.85622961843176),.UNSPECIFIED.);
#234=B_SPLINE_CURVE_WITH_KNOTS('',3,(#12149,#12150,#12151,#12152,#12153,
#12154,#12155,#12156,#12157,#12158,#12159,#12160,#12161,#12162,#12163,#12164,
#12165,#12166,#12167,#12168,#12169,#12170,#12171,#12172,#12173),
 .UNSPECIFIED.,.F.,.F.,(4,3,3,3,3,3,3,3,4),(-3.85622960309808,-3.76518609625559,
-3.67851407926643,-3.59184296748841,-3.50515277910997,-3.49205557572814,
-3.4051555060907,-3.31826970863097,-3.27449886892727),.UNSPECIFIED.);
#235=B_SPLINE_CURVE_WITH_KNOTS('',3,(#12176,#12177,#12178,#12179,#12180,
#12181,#12182,#12183,#12184,#12185,#12186,#12187,#12188,#12189,#12190,#12191,
#12192,#12193,#12194,#12195,#12196,#12197,#12198,#12199,#12200,#12201,#12202,
#12203,#12204,#12205,#12206,#12207,#12208,#12209,#12210,#12211,#12212,#12213,
#12214,#12215,#12216,#12217,#12218,#12219,#12220,#12221,#12222,#12223,#12224,
#12225,#12226,#12227,#12228,#12229,#12230,#12231,#12232,#12233,#12234,#12235,
#12236,#12237,#12238,#12239,#12240,#12241,#12242,#12243,#12244,#12245,#12246,
#12247,#12248,#12249,#12250,#12251,#12252,#12253,#12254,#12255,#12256,#12257,
#12258,#12259,#12260,#12261,#12262,#12263,#12264,#12265,#12266,#12267,#12268,
#12269,#12270,#12271,#12272,#12273,#12274,#12275,#12276,#12277,#12278,#12279,
#12280,#12281,#12282,#12283,#12284,#12285,#12286,#12287,#12288,#12289,#12290,
#12291,#12292,#12293,#12294,#12295,#12296,#12297,#12298,#12299,#12300,#12301,
#12302,#12303,#12304,#12305,#12306,#12307,#12308,#12309,#12310,#12311,#12312,
#12313,#12314,#12315,#12316,#12317,#12318,#12319,#12320,#12321,#12322,#12323),
 .UNSPECIFIED.,.F.,.F.,(4,3,3,3,3,3,3,3,3,3,3,3,3,3,3,3,3,3,3,3,3,3,3,3,
3,3,3,3,3,3,3,3,3,3,3,3,3,3,3,3,3,3,3,3,3,3,3,3,3,4),(17.9335664739021,
18.0167532469952,18.0999437848247,18.1831297542433,18.2663367453336,18.3369797340602,
18.4201844407613,18.5033729159824,18.5865646052947,18.6697507067779,18.7529589155841,
18.8358448163071,18.9190496178174,19.0022381892001,19.0854299758621,19.1686161751527,
19.2518244815942,19.334709898554,19.4179146417019,19.5011031539455,19.5842948808243,
19.6674810200974,19.7506892667057,19.8335749808009,19.9167797515611,19.9999682917609,
20.0831600468638,20.1663462144518,20.2495544892548,20.3324400630477,20.4156448242515,
20.4988333547888,20.5820251001567,20.6652112579893,20.7484195230966,20.8313051452946,
20.9145099078806,20.9976984398057,21.0808901865568,21.1640763457672,21.2472846122301,
21.3301702275415,21.4133749913722,21.4965635245643,21.5797552726057,21.6629414331165,
21.7461497008841,21.8290353097884,21.9152790381123,21.9911485749839),
 .UNSPECIFIED.);
#236=B_SPLINE_CURVE_WITH_KNOTS('',3,(#12324,#12325,#12326,#12327,#12328,
#12329,#12330,#12331,#12332,#12333,#12334,#12335,#12336,#12337,#12338,#12339,
#12340,#12341,#12342,#12343,#12344,#12345,#12346,#12347,#12348,#12349,#12350,
#12351,#12352,#12353,#12354,#12355,#12356,#12357,#12358,#12359,#12360,#12361,
#12362,#12363,#12364,#12365,#12366,#12367,#12368,#12369,#12370,#12371,#12372,
#12373,#12374,#12375,#12376,#12377,#12378,#12379,#12380,#12381,#12382,#12383,
#12384,#12385,#12386,#12387,#12388,#12389,#12390,#12391,#12392,#12393,#12394,
#12395,#12396,#12397,#12398,#12399,#12400,#12401,#12402,#12403,#12404,#12405),
 .UNSPECIFIED.,.F.,.F.,(4,3,3,3,3,3,3,3,3,3,3,3,3,3,3,3,3,3,3,3,3,3,3,3,
3,3,3,4),(21.9911485751285,22.0753365293552,22.1584867074775,22.2431935497563,
22.3279003920352,22.4111051553879,22.4942936880944,22.5774854356416,22.6606715956548,
22.743879862924,22.8267654742821,22.9099702371268,22.9931587693188,23.0763505163464,
23.1595366758383,23.242744942588,23.325630556529,23.4088353195699,23.4920238519602,
23.5752155991881,23.6584017588804,23.7416100258298,23.8244956387759,23.9076996034063,
23.9908936205378,24.0740760457086,24.157266075357,24.216717884951),
 .UNSPECIFIED.);
#237=B_SPLINE_CURVE_WITH_KNOTS('',3,(#12407,#12408,#12409,#12410,#12411,
#12412,#12413,#12414,#12415,#12416,#12417,#12418,#12419,#12420,#12421,#12422,
#12423,#12424,#12425,#12426,#12427,#12428,#12429,#12430,#12431,#12432,#12433,
#12434,#12435,#12436,#12437,#12438,#12439,#12440,#12441,#12442,#12443,#12444,
#12445,#12446,#12447,#12448,#12449,#12450,#12451,#12452,#12453,#12454,#12455,
#12456,#12457,#12458,#12459,#12460,#12461,#12462,#12463,#12464,#12465,#12466,
#12467,#12468,#12469,#12470,#12471,#12472,#12473,#12474,#12475,#12476,#12477,
#12478,#12479,#12480,#12481,#12482,#12483,#12484,#12485,#12486,#12487,#12488),
 .UNSPECIFIED.,.F.,.F.,(4,3,3,3,3,3,3,3,3,3,3,3,3,3,3,3,3,3,3,3,3,3,3,3,
3,3,3,4),(21.9911485751285,22.0740357535315,22.1569243101385,22.2398084002157,
22.3227130388891,22.3802414429218,22.4634462136298,22.5466347537768,22.6298265088266,
22.7130126763613,22.7962209511113,22.8791065251687,22.962311286388,23.0454998169407,
23.1286915623243,23.2118777201727,23.2950859852955,23.3779716074156,23.461176370002,
23.5443649019275,23.627556648679,23.7107428078902,23.7939510743537,23.8768366896625,
23.961807761079,24.0449981194178,24.1308595473731,24.2167209753283),
 .UNSPECIFIED.);
#238=B_SPLINE_CURVE_WITH_KNOTS('',3,(#12489,#12490,#12491,#12492,#12493,
#12494,#12495,#12496,#12497,#12498,#12499,#12500),.UNSPECIFIED.,.F.,.F.,
(4,1,1,1,1,1,1,1,1,4),(17.9335636647299,18.3893207849468,18.8881858671937,
19.3870509494406,19.8859160316874,20.3847811139343,20.8836461961812,21.3825112784281,
21.881376360675,21.9911485751285),.UNSPECIFIED.);
#239=B_SPLINE_CURVE_WITH_KNOTS('',3,(#13106,#13107,#13108,#13109,#13110,
#13111,#13112,#13113,#13114,#13115,#13116,#13117,#13118,#13119,#13120,#13121,
#13122,#13123,#13124,#13125,#13126,#13127,#13128,#13129,#13130,#13131,#13132,
#13133,#13134,#13135,#13136,#13137,#13138,#13139,#13140,#13141,#13142,#13143,
#13144,#13145,#13146,#13147,#13148,#13149,#13150,#13151,#13152,#13153,#13154,
#13155,#13156,#13157,#13158,#13159,#13160,#13161,#13162,#13163,#13164,#13165,
#13166,#13167,#13168,#13169,#13170,#13171,#13172,#13173,#13174,#13175,#13176,
#13177,#13178,#13179,#13180,#13181,#13182,#13183,#13184,#13185,#13186,#13187,
#13188,#13189,#13190,#13191,#13192,#13193,#13194,#13195,#13196,#13197,#13198,
#13199,#13200,#13201,#13202,#13203,#13204,#13205,#13206,#13207,#13208,#13209,
#13210,#13211,#13212,#13213,#13214),.UNSPECIFIED.,.F.,.F.,(4,3,3,3,3,3,
3,3,3,3,3,3,3,3,3,3,3,3,3,3,3,3,3,3,3,3,3,3,3,3,3,3,3,3,3,3,4),(0.,0.0504375942257773,
0.101438275560147,0.152274851141068,0.202297764828748,0.22690245747524,
0.234086631352025,0.240471303452472,0.290088861606672,0.300961710715322,
0.350777659556104,0.400503660438411,0.449535507751653,0.461532737431569,
0.467774024709387,0.516338001498774,0.564497803363664,0.590321666658535,
0.638741707992651,0.678586472467412,0.686372968117243,0.73377925644372,
0.781056303170048,0.827516437945467,0.867854641571887,0.88442683737737,
0.893641475723393,0.901004136370051,0.947492195713632,0.988132467775281,
1.00845260380611,1.02136292095409,1.02877273983693,1.07430587688627,1.11913723974879,
1.13300977445962,1.14791015664666),.UNSPECIFIED.);
#240=B_SPLINE_CURVE_WITH_KNOTS('',3,(#13215,#13216,#13217,#13218,#13219,
#13220,#13221,#13222,#13223,#13224,#13225,#13226,#13227,#13228,#13229,#13230,
#13231,#13232,#13233,#13234,#13235,#13236,#13237,#13238,#13239,#13240,#13241,
#13242,#13243,#13244,#13245,#13246,#13247,#13248,#13249,#13250,#13251,#13252,
#13253,#13254,#13255,#13256,#13257,#13258,#13259,#13260,#13261,#13262,#13263,
#13264,#13265,#13266,#13267,#13268,#13269,#13270,#13271,#13272,#13273,#13274,
#13275,#13276,#13277,#13278,#13279,#13280,#13281,#13282,#13283,#13284,#13285,
#13286,#13287,#13288,#13289,#13290,#13291,#13292,#13293,#13294,#13295,#13296,
#13297,#13298,#13299,#13300,#13301,#13302,#13303,#13304,#13305,#13306,#13307,
#13308,#13309,#13310,#13311,#13312,#13313,#13314,#13315,#13316,#13317),
 .UNSPECIFIED.,.F.,.F.,(4,3,3,3,3,3,3,3,3,3,3,3,3,3,3,3,3,3,3,3,3,3,3,3,
3,3,3,3,3,3,3,3,3,3,4),(0.,0.0441046329368436,0.0893560015723501,0.135009828313389,
0.180704033776388,0.193938392122172,0.203205013495769,0.210348094081718,
0.257081268324377,0.264009708387661,0.310275553315939,0.357011042681633,
0.403920433703055,0.412397541162293,0.418270821497181,0.465898848410438,
0.514060796055048,0.539889422154883,0.58787940607083,0.631052019999542,
0.637374575989874,0.686132719762263,0.735352712852578,0.78461919933138,
0.827437465561715,0.848796759809365,0.857479630116978,0.869246119150075,
0.918875449822967,0.969139233393724,0.998311819542916,1.02159545864218,
1.07387015547638,1.12614485231058,1.14369440702988),.UNSPECIFIED.);
#241=B_SPLINE_CURVE_WITH_KNOTS('',3,(#13318,#13319,#13320,#13321),
 .UNSPECIFIED.,.F.,.F.,(4,4),(-0.000845053830584482,0.),.UNSPECIFIED.);
#242=B_SPLINE_CURVE_WITH_KNOTS('',3,(#13926,#13927,#13928,#13929,#13930,
#13931,#13932,#13933,#13934,#13935,#13936,#13937,#13938,#13939,#13940,#13941,
#13942,#13943,#13944,#13945,#13946,#13947,#13948,#13949,#13950,#13951,#13952,
#13953,#13954,#13955,#13956,#13957,#13958,#13959,#13960,#13961,#13962,#13963,
#13964,#13965,#13966,#13967,#13968,#13969,#13970,#13971,#13972,#13973,#13974,
#13975,#13976,#13977,#13978,#13979,#13980,#13981,#13982,#13983,#13984,#13985,
#13986,#13987,#13988,#13989,#13990,#13991,#13992,#13993,#13994,#13995,#13996,
#13997,#13998,#13999,#14000,#14001,#14002,#14003,#14004,#14005,#14006,#14007,
#14008,#14009,#14010,#14011,#14012,#14013,#14014,#14015,#14016,#14017,#14018,
#14019,#14020,#14021,#14022,#14023,#14024,#14025,#14026,#14027,#14028,#14029,
#14030,#14031),.UNSPECIFIED.,.F.,.F.,(4,3,3,3,3,3,3,3,3,3,3,3,3,3,3,3,3,
3,3,3,3,3,3,3,3,3,3,3,3,3,3,3,3,3,3,4),(0.,0.0441046059006624,0.0893559560019204,
0.135009773091842,0.180703983785403,0.193938306952095,0.20186334331925,
0.20763014540964,0.254347571323218,0.264009708387664,0.310275573079556,
0.357011074596214,0.40392046597413,0.412397589145282,0.418270878708949,
0.465898922469038,0.514060873473489,0.539889422154889,0.587879400706368,
0.63105191632105,0.63737455243671,0.686132686358541,0.735352674476775,0.784619161308775,
0.827437465561743,0.846106677233546,0.854394315893421,0.861034178817951,
0.910558531735202,0.960799533634331,0.998311819663738,1.00642292873682,
1.05734275824645,1.10836149070654,1.12614485231059,1.14369440711896),
 .UNSPECIFIED.);
#243=B_SPLINE_CURVE_WITH_KNOTS('',3,(#14033,#14034,#14035,#14036),
 .UNSPECIFIED.,.F.,.F.,(4,4),(0.,0.000845029145043154),.UNSPECIFIED.);
#244=B_SPLINE_CURVE_WITH_KNOTS('',3,(#14037,#14038,#14039,#14040,#14041,
#14042,#14043,#14044,#14045,#14046,#14047,#14048,#14049,#14050,#14051,#14052,
#14053,#14054,#14055,#14056,#14057,#14058,#14059,#14060,#14061,#14062,#14063,
#14064,#14065,#14066,#14067,#14068,#14069,#14070,#14071,#14072,#14073,#14074,
#14075,#14076,#14077,#14078,#14079,#14080,#14081,#14082,#14083,#14084,#14085,
#14086,#14087,#14088,#14089,#14090,#14091,#14092,#14093,#14094,#14095,#14096,
#14097,#14098,#14099,#14100,#14101,#14102,#14103,#14104,#14105,#14106,#14107,
#14108,#14109,#14110,#14111,#14112,#14113,#14114,#14115,#14116,#14117,#14118,
#14119,#14120,#14121,#14122,#14123,#14124,#14125,#14126,#14127,#14128,#14129,
#14130,#14131,#14132,#14133,#14134,#14135,#14136,#14137,#14138,#14139,#14140,
#14141,#14142),.UNSPECIFIED.,.F.,.F.,(4,3,3,3,3,3,3,3,3,3,3,3,3,3,3,3,3,
3,3,3,3,3,3,3,3,3,3,3,3,3,3,3,3,3,3,4),(0.,0.0504375760143521,0.101438257257583,
0.152274841648771,0.202297771586617,0.226902464456934,0.234086657304898,
0.24047130670072,0.290088872824462,0.300961710715323,0.350765609901174,
0.400474445038685,0.447936250443642,0.461532739091791,0.473284706306216,
0.521843710447206,0.569966130302076,0.590321666658515,0.638741707119349,
0.678586470967118,0.686372967853733,0.733779255798812,0.781056301894992,
0.827516432241143,0.867854641571862,0.894324374113917,0.901004135934422,
0.947484960275739,0.993866163821704,1.01125911515144,1.02227210782131,1.03199949352102,
1.07751008814374,1.12231103370646,1.1330097744596,1.14791015664664),
 .UNSPECIFIED.);
#416=SHAPE_REPRESENTATION_RELATIONSHIP('SRR','None',#37785,#434);
#434=ADVANCED_BREP_SHAPE_REPRESENTATION('',(#470),#37689);
#452=STYLED_ITEM('',(#37880),#470);
#470=MANIFOLD_SOLID_BREP('Body1',#4150);
#500=FACE_BOUND('',#913,.T.);
#501=FACE_BOUND('',#916,.T.);
#552=PLANE('',#4483);
#553=PLANE('',#4487);
#656=FACE_OUTER_BOUND('',#886,.T.);
#657=FACE_OUTER_BOUND('',#887,.T.);
#658=FACE_OUTER_BOUND('',#888,.T.);
#659=FACE_OUTER_BOUND('',#889,.T.);
#660=FACE_OUTER_BOUND('',#890,.T.);
#661=FACE_OUTER_BOUND('',#891,.T.);
#662=FACE_OUTER_BOUND('',#892,.T.);
#663=FACE_OUTER_BOUND('',#893,.T.);
#664=FACE_OUTER_BOUND('',#894,.T.);
#665=FACE_OUTER_BOUND('',#895,.T.);
#666=FACE_OUTER_BOUND('',#896,.T.);
#667=FACE_OUTER_BOUND('',#897,.T.);
#668=FACE_OUTER_BOUND('',#898,.T.);
#669=FACE_OUTER_BOUND('',#899,.T.);
#670=FACE_OUTER_BOUND('',#900,.T.);
#671=FACE_OUTER_BOUND('',#901,.T.);
#672=FACE_OUTER_BOUND('',#902,.T.);
#673=FACE_OUTER_BOUND('',#903,.T.);
#674=FACE_OUTER_BOUND('',#904,.T.);
#675=FACE_OUTER_BOUND('',#905,.T.);
#676=FACE_OUTER_BOUND('',#906,.T.);
#677=FACE_OUTER_BOUND('',#907,.T.);
#678=FACE_OUTER_BOUND('',#908,.T.);
#679=FACE_OUTER_BOUND('',#909,.T.);
#680=FACE_OUTER_BOUND('',#910,.T.);
#681=FACE_OUTER_BOUND('',#911,.T.);
#682=FACE_OUTER_BOUND('',#912,.T.);
#683=FACE_OUTER_BOUND('',#914,.T.);
#684=FACE_OUTER_BOUND('',#915,.T.);
#886=EDGE_LOOP('',(#2883,#2884,#2885,#2886,#2887,#2888));
#887=EDGE_LOOP('',(#2889,#2890,#2891,#2892,#2893,#2894));
#888=EDGE_LOOP('',(#2895,#2896,#2897,#2898,#2899,#2900));
#889=EDGE_LOOP('',(#2901,#2902,#2903,#2904,#2905,#2906));
#890=EDGE_LOOP('',(#2907,#2908,#2909,#2910,#2911,#2912));
#891=EDGE_LOOP('',(#2913,#2914,#2915,#2916,#2917,#2918));
#892=EDGE_LOOP('',(#2919,#2920,#2921,#2922,#2923,#2924));
#893=EDGE_LOOP('',(#2925,#2926,#2927,#2928,#2929,#2930));
#894=EDGE_LOOP('',(#2931,#2932,#2933,#2934,#2935,#2936));
#895=EDGE_LOOP('',(#2937,#2938,#2939,#2940,#2941,#2942));
#896=EDGE_LOOP('',(#2943,#2944,#2945,#2946,#2947,#2948));
#897=EDGE_LOOP('',(#2949,#2950,#2951,#2952));
#898=EDGE_LOOP('',(#2953,#2954,#2955,#2956,#2957,#2958));
#899=EDGE_LOOP('',(#2959,#2960,#2961,#2962,#2963,#2964));
#900=EDGE_LOOP('',(#2965,#2966,#2967,#2968,#2969,#2970));
#901=EDGE_LOOP('',(#2971,#2972,#2973,#2974,#2975));
#902=EDGE_LOOP('',(#2976,#2977,#2978,#2979,#2980,#2981));
#903=EDGE_LOOP('',(#2982,#2983,#2984,#2985,#2986));
#904=EDGE_LOOP('',(#2987,#2988,#2989,#2990,#2991,#2992));
#905=EDGE_LOOP('',(#2993,#2994,#2995,#2996));
#906=EDGE_LOOP('',(#2997,#2998,#2999,#3000,#3001,#3002));
#907=EDGE_LOOP('',(#3003,#3004,#3005,#3006));
#908=EDGE_LOOP('',(#3007,#3008,#3009,#3010,#3011));
#909=EDGE_LOOP('',(#3012,#3013,#3014,#3015,#3016,#3017));
#910=EDGE_LOOP('',(#3018,#3019,#3020,#3021,#3022,#3023,#3024,#3025,#3026,
#3027,#3028,#3029,#3030,#3031,#3032,#3033,#3034,#3035,#3036,#3037,#3038,
#3039,#3040,#3041,#3042,#3043,#3044,#3045,#3046,#3047,#3048,#3049,#3050,
#3051,#3052,#3053,#3054,#3055,#3056,#3057,#3058,#3059,#3060,#3061,#3062,
#3063,#3064));
#911=EDGE_LOOP('',(#3065,#3066,#3067,#3068,#3069,#3070,#3071,#3072,#3073,
#3074,#3075,#3076,#3077,#3078,#3079,#3080,#3081,#3082,#3083,#3084,#3085,
#3086,#3087,#3088,#3089,#3090,#3091,#3092,#3093,#3094,#3095,#3096,#3097,
#3098,#3099,#3100,#3101,#3102,#3103,#3104,#3105,#3106,#3107,#3108,#3109,
#3110));
#912=EDGE_LOOP('',(#3111));
#913=EDGE_LOOP('',(#3112,#3113,#3114,#3115,#3116));
#914=EDGE_LOOP('',(#3117,#3118,#3119,#3120));
#915=EDGE_LOOP('',(#3121));
#916=EDGE_LOOP('',(#3122,#3123,#3124,#3125,#3126));
#1150=LINE('',#5915,#1399);
#1151=LINE('',#6005,#1400);
#1152=LINE('',#6189,#1401);
#1153=LINE('',#6588,#1402);
#1154=LINE('',#6782,#1403);
#1155=LINE('',#7105,#1404);
#1156=LINE('',#7577,#1405);
#1157=LINE('',#8052,#1406);
#1158=LINE('',#8389,#1407);
#1159=LINE('',#8787,#1408);
#1160=LINE('',#9259,#1409);
#1161=LINE('',#9438,#1410);
#1162=LINE('',#9611,#1411);
#1163=LINE('',#9848,#1412);
#1164=LINE('',#10107,#1413);
#1165=LINE('',#10373,#1414);
#1166=LINE('',#10706,#1415);
#1167=LINE('',#10846,#1416);
#1168=LINE('',#11009,#1417);
#1169=LINE('',#11349,#1418);
#1170=LINE('',#11583,#1419);
#1171=LINE('',#11808,#1420);
#1172=LINE('',#14148,#1421);
#1399=VECTOR('',#4987,6.11325);
#1400=VECTOR('',#4992,6.11325);
#1401=VECTOR('',#4995,6.11325);
#1402=VECTOR('',#4998,6.11325);
#1403=VECTOR('',#5001,6.11325);
#1404=VECTOR('',#5004,6.11325);
#1405=VECTOR('',#5007,6.11325);
#1406=VECTOR('',#5010,6.11325);
#1407=VECTOR('',#5013,6.11325);
#1408=VECTOR('',#5016,6.11325);
#1409=VECTOR('',#5019,6.11325);
#1410=VECTOR('',#5024,5.13675);
#1411=VECTOR('',#5029,5.13675);
#1412=VECTOR('',#5032,5.13675);
#1413=VECTOR('',#5035,5.13675);
#1414=VECTOR('',#5038,5.13675);
#1415=VECTOR('',#5041,5.13675);
#1416=VECTOR('',#5044,5.13675);
#1417=VECTOR('',#5047,5.13675);
#1418=VECTOR('',#5050,5.13675);
#1419=VECTOR('',#5053,5.13675);
#1420=VECTOR('',#5056,5.13675);
#1421=VECTOR('',#5069,12.);
#1586=CIRCLE('',#4456,6.11325);
#1587=CIRCLE('',#4467,6.11325);
#1588=CIRCLE('',#4469,5.13675);
#1589=CIRCLE('',#4480,5.13675);
#1590=CIRCLE('',#4484,12.);
#1591=CIRCLE('',#4486,12.);
#1717=VERTEX_POINT('',#5913);
#1718=VERTEX_POINT('',#5914);
#1719=VERTEX_POINT('',#5916);
#1720=VERTEX_POINT('',#5929);
#1721=VERTEX_POINT('',#5935);
#1722=VERTEX_POINT('',#5937);
#1723=VERTEX_POINT('',#6003);
#1724=VERTEX_POINT('',#6004);
#1725=VERTEX_POINT('',#6006);
#1726=VERTEX_POINT('',#6164);
#1727=VERTEX_POINT('',#6187);
#1728=VERTEX_POINT('',#6188);
#1729=VERTEX_POINT('',#6190);
#1730=VERTEX_POINT('',#6427);
#1731=VERTEX_POINT('',#6586);
#1732=VERTEX_POINT('',#6587);
#1733=VERTEX_POINT('',#6589);
#1734=VERTEX_POINT('',#6684);
#1735=VERTEX_POINT('',#6780);
#1736=VERTEX_POINT('',#6781);
#1737=VERTEX_POINT('',#6783);
#1738=VERTEX_POINT('',#6944);
#1739=VERTEX_POINT('',#7103);
#1740=VERTEX_POINT('',#7104);
#1741=VERTEX_POINT('',#7106);
#1742=VERTEX_POINT('',#7340);
#1743=VERTEX_POINT('',#7575);
#1744=VERTEX_POINT('',#7576);
#1745=VERTEX_POINT('',#7578);
#1746=VERTEX_POINT('',#7812);
#1747=VERTEX_POINT('',#8050);
#1748=VERTEX_POINT('',#8051);
#1749=VERTEX_POINT('',#8053);
#1750=VERTEX_POINT('',#8152);
#1751=VERTEX_POINT('',#8387);
#1752=VERTEX_POINT('',#8388);
#1753=VERTEX_POINT('',#8390);
#1754=VERTEX_POINT('',#8547);
#1755=VERTEX_POINT('',#8785);
#1756=VERTEX_POINT('',#8786);
#1757=VERTEX_POINT('',#8788);
#1758=VERTEX_POINT('',#9025);
#1759=VERTEX_POINT('',#9257);
#1760=VERTEX_POINT('',#9258);
#1761=VERTEX_POINT('',#9260);
#1762=VERTEX_POINT('',#9270);
#1763=VERTEX_POINT('',#9277);
#1764=VERTEX_POINT('',#9279);
#1765=VERTEX_POINT('',#9436);
#1766=VERTEX_POINT('',#9437);
#1767=VERTEX_POINT('',#9439);
#1768=VERTEX_POINT('',#9508);
#1769=VERTEX_POINT('',#9609);
#1770=VERTEX_POINT('',#9610);
#1771=VERTEX_POINT('',#9612);
#1772=VERTEX_POINT('',#9738);
#1773=VERTEX_POINT('',#9846);
#1774=VERTEX_POINT('',#9847);
#1775=VERTEX_POINT('',#9849);
#1776=VERTEX_POINT('',#10066);
#1777=VERTEX_POINT('',#10105);
#1778=VERTEX_POINT('',#10106);
#1779=VERTEX_POINT('',#10108);
#1780=VERTEX_POINT('',#10149);
#1781=VERTEX_POINT('',#10371);
#1782=VERTEX_POINT('',#10372);
#1783=VERTEX_POINT('',#10374);
#1784=VERTEX_POINT('',#10704);
#1785=VERTEX_POINT('',#10705);
#1786=VERTEX_POINT('',#10707);
#1787=VERTEX_POINT('',#10735);
#1788=VERTEX_POINT('',#10844);
#1789=VERTEX_POINT('',#10845);
#1790=VERTEX_POINT('',#10965);
#1791=VERTEX_POINT('',#11007);
#1792=VERTEX_POINT('',#11008);
#1793=VERTEX_POINT('',#11010);
#1794=VERTEX_POINT('',#11125);
#1795=VERTEX_POINT('',#11347);
#1796=VERTEX_POINT('',#11348);
#1797=VERTEX_POINT('',#11581);
#1798=VERTEX_POINT('',#11582);
#1799=VERTEX_POINT('',#11584);
#1800=VERTEX_POINT('',#11701);
#1801=VERTEX_POINT('',#11806);
#1802=VERTEX_POINT('',#11807);
#1803=VERTEX_POINT('',#11809);
#1804=VERTEX_POINT('',#11931);
#1805=VERTEX_POINT('',#12132);
#1806=VERTEX_POINT('',#12175);
#1807=VERTEX_POINT('',#12406);
#1808=VERTEX_POINT('',#13105);
#1809=VERTEX_POINT('',#14032);
#1810=VERTEX_POINT('',#14144);
#1811=VERTEX_POINT('',#14147);
#2175=EDGE_CURVE('',#1717,#1718,#1150,.T.);
#2176=EDGE_CURVE('',#1718,#1719,#152,.T.);
#2177=EDGE_CURVE('',#1719,#1720,#153,.T.);
#2178=EDGE_CURVE('',#1721,#1720,#1586,.T.);
#2179=EDGE_CURVE('',#1722,#1721,#154,.T.);
#2180=EDGE_CURVE('',#1717,#1722,#155,.T.);
#2181=EDGE_CURVE('',#1723,#1724,#1151,.T.);
#2182=EDGE_CURVE('',#1724,#1725,#156,.T.);
#2183=EDGE_CURVE('',#1725,#1718,#157,.T.);
#2184=EDGE_CURVE('',#1726,#1717,#158,.T.);
#2185=EDGE_CURVE('',#1723,#1726,#159,.T.);
#2186=EDGE_CURVE('',#1727,#1728,#1152,.T.);
#2187=EDGE_CURVE('',#1728,#1729,#160,.T.);
#2188=EDGE_CURVE('',#1729,#1724,#161,.T.);
#2189=EDGE_CURVE('',#1730,#1723,#162,.T.);
#2190=EDGE_CURVE('',#1727,#1730,#163,.T.);
#2191=EDGE_CURVE('',#1731,#1732,#1153,.T.);
#2192=EDGE_CURVE('',#1732,#1733,#164,.T.);
#2193=EDGE_CURVE('',#1733,#1728,#165,.T.);
#2194=EDGE_CURVE('',#1734,#1727,#166,.T.);
#2195=EDGE_CURVE('',#1731,#1734,#167,.T.);
#2196=EDGE_CURVE('',#1735,#1736,#1154,.T.);
#2197=EDGE_CURVE('',#1736,#1737,#168,.T.);
#2198=EDGE_CURVE('',#1737,#1732,#169,.T.);
#2199=EDGE_CURVE('',#1738,#1731,#170,.T.);
#2200=EDGE_CURVE('',#1735,#1738,#171,.T.);
#2201=EDGE_CURVE('',#1739,#1740,#1155,.T.);
#2202=EDGE_CURVE('',#1740,#1741,#172,.T.);
#2203=EDGE_CURVE('',#1741,#1736,#173,.T.);
#2204=EDGE_CURVE('',#1742,#1735,#174,.T.);
#2205=EDGE_CURVE('',#1739,#1742,#175,.T.);
#2206=EDGE_CURVE('',#1743,#1744,#1156,.T.);
#2207=EDGE_CURVE('',#1744,#1745,#176,.T.);
#2208=EDGE_CURVE('',#1745,#1740,#177,.T.);
#2209=EDGE_CURVE('',#1746,#1739,#178,.T.);
#2210=EDGE_CURVE('',#1743,#1746,#179,.T.);
#2211=EDGE_CURVE('',#1747,#1748,#1157,.T.);
#2212=EDGE_CURVE('',#1748,#1749,#180,.T.);
#2213=EDGE_CURVE('',#1749,#1744,#181,.T.);
#2214=EDGE_CURVE('',#1750,#1743,#182,.T.);
#2215=EDGE_CURVE('',#1747,#1750,#183,.T.);
#2216=EDGE_CURVE('',#1751,#1752,#1158,.T.);
#2217=EDGE_CURVE('',#1752,#1753,#184,.T.);
#2218=EDGE_CURVE('',#1753,#1748,#185,.T.);
#2219=EDGE_CURVE('',#1754,#1747,#186,.T.);
#2220=EDGE_CURVE('',#1751,#1754,#187,.T.);
#2221=EDGE_CURVE('',#1755,#1756,#1159,.T.);
#2222=EDGE_CURVE('',#1756,#1757,#188,.T.);
#2223=EDGE_CURVE('',#1757,#1752,#189,.T.);
#2224=EDGE_CURVE('',#1758,#1751,#190,.T.);
#2225=EDGE_CURVE('',#1755,#1758,#191,.T.);
#2226=EDGE_CURVE('',#1759,#1760,#1160,.T.);
#2227=EDGE_CURVE('',#1761,#1759,#192,.T.);
#2228=EDGE_CURVE('',#1762,#1761,#193,.T.);
#2229=EDGE_CURVE('',#1763,#1762,#1587,.T.);
#2230=EDGE_CURVE('',#1763,#1764,#194,.T.);
#2231=EDGE_CURVE('',#1764,#1760,#195,.T.);
#2232=EDGE_CURVE('',#1765,#1766,#1161,.T.);
#2233=EDGE_CURVE('',#1766,#1767,#196,.F.);
#2234=EDGE_CURVE('',#1768,#1767,#1588,.F.);
#2235=EDGE_CURVE('',#1768,#1765,#197,.T.);
#2236=EDGE_CURVE('',#1769,#1770,#1162,.T.);
#2237=EDGE_CURVE('',#1770,#1771,#198,.T.);
#2238=EDGE_CURVE('',#1771,#1766,#199,.F.);
#2239=EDGE_CURVE('',#1765,#1772,#200,.T.);
#2240=EDGE_CURVE('',#1772,#1769,#201,.T.);
#2241=EDGE_CURVE('',#1773,#1774,#1163,.T.);
#2242=EDGE_CURVE('',#1774,#1775,#202,.T.);
#2243=EDGE_CURVE('',#1775,#1770,#203,.T.);
#2244=EDGE_CURVE('',#1769,#1776,#204,.T.);
#2245=EDGE_CURVE('',#1776,#1773,#205,.T.);
#2246=EDGE_CURVE('',#1777,#1778,#1164,.T.);
#2247=EDGE_CURVE('',#1778,#1779,#206,.T.);
#2248=EDGE_CURVE('',#1779,#1774,#207,.T.);
#2249=EDGE_CURVE('',#1773,#1780,#208,.T.);
#2250=EDGE_CURVE('',#1780,#1777,#209,.T.);
#2251=EDGE_CURVE('',#1781,#1782,#1165,.T.);
#2252=EDGE_CURVE('',#1782,#1783,#210,.T.);
#2253=EDGE_CURVE('',#1783,#1778,#211,.T.);
#2254=EDGE_CURVE('',#1777,#1781,#212,.T.);
#2255=EDGE_CURVE('',#1784,#1785,#1166,.T.);
#2256=EDGE_CURVE('',#1785,#1786,#213,.T.);
#2257=EDGE_CURVE('',#1786,#1782,#214,.T.);
#2258=EDGE_CURVE('',#1781,#1787,#215,.T.);
#2259=EDGE_CURVE('',#1787,#1784,#216,.T.);
#2260=EDGE_CURVE('',#1788,#1789,#1167,.T.);
#2261=EDGE_CURVE('',#1789,#1785,#217,.T.);
#2262=EDGE_CURVE('',#1784,#1790,#218,.T.);
#2263=EDGE_CURVE('',#1790,#1788,#219,.T.);
#2264=EDGE_CURVE('',#1791,#1792,#1168,.T.);
#2265=EDGE_CURVE('',#1792,#1793,#220,.T.);
#2266=EDGE_CURVE('',#1793,#1789,#221,.T.);
#2267=EDGE_CURVE('',#1788,#1794,#222,.T.);
#2268=EDGE_CURVE('',#1794,#1791,#223,.T.);
#2269=EDGE_CURVE('',#1795,#1796,#1169,.T.);
#2270=EDGE_CURVE('',#1796,#1792,#224,.T.);
#2271=EDGE_CURVE('',#1791,#1795,#225,.T.);
#2272=EDGE_CURVE('',#1797,#1798,#1170,.T.);
#2273=EDGE_CURVE('',#1798,#1799,#226,.T.);
#2274=EDGE_CURVE('',#1799,#1796,#227,.T.);
#2275=EDGE_CURVE('',#1795,#1800,#228,.T.);
#2276=EDGE_CURVE('',#1800,#1797,#229,.T.);
#2277=EDGE_CURVE('',#1801,#1802,#1171,.T.);
#2278=EDGE_CURVE('',#1801,#1803,#230,.T.);
#2279=EDGE_CURVE('',#1803,#1804,#1589,.F.);
#2280=EDGE_CURVE('',#1804,#1802,#231,.T.);
#2281=EDGE_CURVE('',#1802,#1798,#232,.T.);
#2282=EDGE_CURVE('',#1797,#1805,#233,.T.);
#2283=EDGE_CURVE('',#1805,#1801,#234,.T.);
#2284=EDGE_CURVE('',#1760,#1806,#235,.T.);
#2285=EDGE_CURVE('',#1806,#1756,#236,.T.);
#2286=EDGE_CURVE('',#1807,#1755,#237,.T.);
#2287=EDGE_CURVE('',#1759,#1807,#238,.T.);
#2288=EDGE_CURVE('',#1720,#1808,#239,.T.);
#2289=EDGE_CURVE('',#1803,#1763,#240,.T.);
#2290=EDGE_CURVE('',#1808,#1768,#241,.T.);
#2291=EDGE_CURVE('',#1767,#1721,#242,.T.);
#2292=EDGE_CURVE('',#1804,#1809,#243,.T.);
#2293=EDGE_CURVE('',#1762,#1809,#244,.T.);
#2294=EDGE_CURVE('',#1810,#1810,#1590,.T.);
#2295=EDGE_CURVE('',#1810,#1811,#1172,.T.);
#2296=EDGE_CURVE('',#1811,#1811,#1591,.T.);
#2883=ORIENTED_EDGE('',*,*,#2175,.T.);
#2884=ORIENTED_EDGE('',*,*,#2176,.T.);
#2885=ORIENTED_EDGE('',*,*,#2177,.T.);
#2886=ORIENTED_EDGE('',*,*,#2178,.F.);
#2887=ORIENTED_EDGE('',*,*,#2179,.F.);
#2888=ORIENTED_EDGE('',*,*,#2180,.F.);
#2889=ORIENTED_EDGE('',*,*,#2181,.T.);
#2890=ORIENTED_EDGE('',*,*,#2182,.T.);
#2891=ORIENTED_EDGE('',*,*,#2183,.T.);
#2892=ORIENTED_EDGE('',*,*,#2175,.F.);
#2893=ORIENTED_EDGE('',*,*,#2184,.F.);
#2894=ORIENTED_EDGE('',*,*,#2185,.F.);
#2895=ORIENTED_EDGE('',*,*,#2186,.T.);
#2896=ORIENTED_EDGE('',*,*,#2187,.T.);
#2897=ORIENTED_EDGE('',*,*,#2188,.T.);
#2898=ORIENTED_EDGE('',*,*,#2181,.F.);
#2899=ORIENTED_EDGE('',*,*,#2189,.F.);
#2900=ORIENTED_EDGE('',*,*,#2190,.F.);
#2901=ORIENTED_EDGE('',*,*,#2191,.T.);
#2902=ORIENTED_EDGE('',*,*,#2192,.T.);
#2903=ORIENTED_EDGE('',*,*,#2193,.T.);
#2904=ORIENTED_EDGE('',*,*,#2186,.F.);
#2905=ORIENTED_EDGE('',*,*,#2194,.F.);
#2906=ORIENTED_EDGE('',*,*,#2195,.F.);
#2907=ORIENTED_EDGE('',*,*,#2196,.T.);
#2908=ORIENTED_EDGE('',*,*,#2197,.T.);
#2909=ORIENTED_EDGE('',*,*,#2198,.T.);
#2910=ORIENTED_EDGE('',*,*,#2191,.F.);
#2911=ORIENTED_EDGE('',*,*,#2199,.F.);
#2912=ORIENTED_EDGE('',*,*,#2200,.F.);
#2913=ORIENTED_EDGE('',*,*,#2201,.T.);
#2914=ORIENTED_EDGE('',*,*,#2202,.T.);
#2915=ORIENTED_EDGE('',*,*,#2203,.T.);
#2916=ORIENTED_EDGE('',*,*,#2196,.F.);
#2917=ORIENTED_EDGE('',*,*,#2204,.F.);
#2918=ORIENTED_EDGE('',*,*,#2205,.F.);
#2919=ORIENTED_EDGE('',*,*,#2206,.T.);
#2920=ORIENTED_EDGE('',*,*,#2207,.T.);
#2921=ORIENTED_EDGE('',*,*,#2208,.T.);
#2922=ORIENTED_EDGE('',*,*,#2201,.F.);
#2923=ORIENTED_EDGE('',*,*,#2209,.F.);
#2924=ORIENTED_EDGE('',*,*,#2210,.F.);
#2925=ORIENTED_EDGE('',*,*,#2211,.T.);
#2926=ORIENTED_EDGE('',*,*,#2212,.T.);
#2927=ORIENTED_EDGE('',*,*,#2213,.T.);
#2928=ORIENTED_EDGE('',*,*,#2206,.F.);
#2929=ORIENTED_EDGE('',*,*,#2214,.F.);
#2930=ORIENTED_EDGE('',*,*,#2215,.F.);
#2931=ORIENTED_EDGE('',*,*,#2216,.T.);
#2932=ORIENTED_EDGE('',*,*,#2217,.T.);
#2933=ORIENTED_EDGE('',*,*,#2218,.T.);
#2934=ORIENTED_EDGE('',*,*,#2211,.F.);
#2935=ORIENTED_EDGE('',*,*,#2219,.F.);
#2936=ORIENTED_EDGE('',*,*,#2220,.F.);
#2937=ORIENTED_EDGE('',*,*,#2221,.T.);
#2938=ORIENTED_EDGE('',*,*,#2222,.T.);
#2939=ORIENTED_EDGE('',*,*,#2223,.T.);
#2940=ORIENTED_EDGE('',*,*,#2216,.F.);
#2941=ORIENTED_EDGE('',*,*,#2224,.F.);
#2942=ORIENTED_EDGE('',*,*,#2225,.F.);
#2943=ORIENTED_EDGE('',*,*,#2226,.F.);
#2944=ORIENTED_EDGE('',*,*,#2227,.F.);
#2945=ORIENTED_EDGE('',*,*,#2228,.F.);
#2946=ORIENTED_EDGE('',*,*,#2229,.F.);
#2947=ORIENTED_EDGE('',*,*,#2230,.T.);
#2948=ORIENTED_EDGE('',*,*,#2231,.T.);
#2949=ORIENTED_EDGE('',*,*,#2232,.T.);
#2950=ORIENTED_EDGE('',*,*,#2233,.T.);
#2951=ORIENTED_EDGE('',*,*,#2234,.F.);
#2952=ORIENTED_EDGE('',*,*,#2235,.T.);
#2953=ORIENTED_EDGE('',*,*,#2236,.T.);
#2954=ORIENTED_EDGE('',*,*,#2237,.T.);
#2955=ORIENTED_EDGE('',*,*,#2238,.T.);
#2956=ORIENTED_EDGE('',*,*,#2232,.F.);
#2957=ORIENTED_EDGE('',*,*,#2239,.T.);
#2958=ORIENTED_EDGE('',*,*,#2240,.T.);
#2959=ORIENTED_EDGE('',*,*,#2241,.T.);
#2960=ORIENTED_EDGE('',*,*,#2242,.T.);
#2961=ORIENTED_EDGE('',*,*,#2243,.T.);
#2962=ORIENTED_EDGE('',*,*,#2236,.F.);
#2963=ORIENTED_EDGE('',*,*,#2244,.T.);
#2964=ORIENTED_EDGE('',*,*,#2245,.T.);
#2965=ORIENTED_EDGE('',*,*,#2246,.T.);
#2966=ORIENTED_EDGE('',*,*,#2247,.T.);
#2967=ORIENTED_EDGE('',*,*,#2248,.T.);
#2968=ORIENTED_EDGE('',*,*,#2241,.F.);
#2969=ORIENTED_EDGE('',*,*,#2249,.T.);
#2970=ORIENTED_EDGE('',*,*,#2250,.T.);
#2971=ORIENTED_EDGE('',*,*,#2251,.T.);
#2972=ORIENTED_EDGE('',*,*,#2252,.T.);
#2973=ORIENTED_EDGE('',*,*,#2253,.T.);
#2974=ORIENTED_EDGE('',*,*,#2246,.F.);
#2975=ORIENTED_EDGE('',*,*,#2254,.T.);
#2976=ORIENTED_EDGE('',*,*,#2255,.T.);
#2977=ORIENTED_EDGE('',*,*,#2256,.T.);
#2978=ORIENTED_EDGE('',*,*,#2257,.T.);
#2979=ORIENTED_EDGE('',*,*,#2251,.F.);
#2980=ORIENTED_EDGE('',*,*,#2258,.T.);
#2981=ORIENTED_EDGE('',*,*,#2259,.T.);
#2982=ORIENTED_EDGE('',*,*,#2260,.T.);
#2983=ORIENTED_EDGE('',*,*,#2261,.T.);
#2984=ORIENTED_EDGE('',*,*,#2255,.F.);
#2985=ORIENTED_EDGE('',*,*,#2262,.T.);
#2986=ORIENTED_EDGE('',*,*,#2263,.T.);
#2987=ORIENTED_EDGE('',*,*,#2264,.T.);
#2988=ORIENTED_EDGE('',*,*,#2265,.T.);
#2989=ORIENTED_EDGE('',*,*,#2266,.T.);
#2990=ORIENTED_EDGE('',*,*,#2260,.F.);
#2991=ORIENTED_EDGE('',*,*,#2267,.T.);
#2992=ORIENTED_EDGE('',*,*,#2268,.T.);
#2993=ORIENTED_EDGE('',*,*,#2269,.T.);
#2994=ORIENTED_EDGE('',*,*,#2270,.T.);
#2995=ORIENTED_EDGE('',*,*,#2264,.F.);
#2996=ORIENTED_EDGE('',*,*,#2271,.T.);
#2997=ORIENTED_EDGE('',*,*,#2272,.T.);
#2998=ORIENTED_EDGE('',*,*,#2273,.T.);
#2999=ORIENTED_EDGE('',*,*,#2274,.T.);
#3000=ORIENTED_EDGE('',*,*,#2269,.F.);
#3001=ORIENTED_EDGE('',*,*,#2275,.T.);
#3002=ORIENTED_EDGE('',*,*,#2276,.T.);
#3003=ORIENTED_EDGE('',*,*,#2277,.F.);
#3004=ORIENTED_EDGE('',*,*,#2278,.T.);
#3005=ORIENTED_EDGE('',*,*,#2279,.T.);
#3006=ORIENTED_EDGE('',*,*,#2280,.T.);
#3007=ORIENTED_EDGE('',*,*,#2277,.T.);
#3008=ORIENTED_EDGE('',*,*,#2281,.T.);
#3009=ORIENTED_EDGE('',*,*,#2272,.F.);
#3010=ORIENTED_EDGE('',*,*,#2282,.T.);
#3011=ORIENTED_EDGE('',*,*,#2283,.T.);
#3012=ORIENTED_EDGE('',*,*,#2226,.T.);
#3013=ORIENTED_EDGE('',*,*,#2284,.T.);
#3014=ORIENTED_EDGE('',*,*,#2285,.T.);
#3015=ORIENTED_EDGE('',*,*,#2221,.F.);
#3016=ORIENTED_EDGE('',*,*,#2286,.F.);
#3017=ORIENTED_EDGE('',*,*,#2287,.F.);
#3018=ORIENTED_EDGE('',*,*,#2288,.F.);
#3019=ORIENTED_EDGE('',*,*,#2177,.F.);
#3020=ORIENTED_EDGE('',*,*,#2176,.F.);
#3021=ORIENTED_EDGE('',*,*,#2183,.F.);
#3022=ORIENTED_EDGE('',*,*,#2182,.F.);
#3023=ORIENTED_EDGE('',*,*,#2188,.F.);
#3024=ORIENTED_EDGE('',*,*,#2187,.F.);
#3025=ORIENTED_EDGE('',*,*,#2193,.F.);
#3026=ORIENTED_EDGE('',*,*,#2192,.F.);
#3027=ORIENTED_EDGE('',*,*,#2198,.F.);
#3028=ORIENTED_EDGE('',*,*,#2197,.F.);
#3029=ORIENTED_EDGE('',*,*,#2203,.F.);
#3030=ORIENTED_EDGE('',*,*,#2202,.F.);
#3031=ORIENTED_EDGE('',*,*,#2208,.F.);
#3032=ORIENTED_EDGE('',*,*,#2207,.F.);
#3033=ORIENTED_EDGE('',*,*,#2213,.F.);
#3034=ORIENTED_EDGE('',*,*,#2212,.F.);
#3035=ORIENTED_EDGE('',*,*,#2218,.F.);
#3036=ORIENTED_EDGE('',*,*,#2217,.F.);
#3037=ORIENTED_EDGE('',*,*,#2223,.F.);
#3038=ORIENTED_EDGE('',*,*,#2222,.F.);
#3039=ORIENTED_EDGE('',*,*,#2285,.F.);
#3040=ORIENTED_EDGE('',*,*,#2284,.F.);
#3041=ORIENTED_EDGE('',*,*,#2231,.F.);
#3042=ORIENTED_EDGE('',*,*,#2230,.F.);
#3043=ORIENTED_EDGE('',*,*,#2289,.F.);
#3044=ORIENTED_EDGE('',*,*,#2278,.F.);
#3045=ORIENTED_EDGE('',*,*,#2283,.F.);
#3046=ORIENTED_EDGE('',*,*,#2282,.F.);
#3047=ORIENTED_EDGE('',*,*,#2276,.F.);
#3048=ORIENTED_EDGE('',*,*,#2275,.F.);
#3049=ORIENTED_EDGE('',*,*,#2271,.F.);
#3050=ORIENTED_EDGE('',*,*,#2268,.F.);
#3051=ORIENTED_EDGE('',*,*,#2267,.F.);
#3052=ORIENTED_EDGE('',*,*,#2263,.F.);
#3053=ORIENTED_EDGE('',*,*,#2262,.F.);
#3054=ORIENTED_EDGE('',*,*,#2259,.F.);
#3055=ORIENTED_EDGE('',*,*,#2258,.F.);
#3056=ORIENTED_EDGE('',*,*,#2254,.F.);
#3057=ORIENTED_EDGE('',*,*,#2250,.F.);
#3058=ORIENTED_EDGE('',*,*,#2249,.F.);
#3059=ORIENTED_EDGE('',*,*,#2245,.F.);
#3060=ORIENTED_EDGE('',*,*,#2244,.F.);
#3061=ORIENTED_EDGE('',*,*,#2240,.F.);
#3062=ORIENTED_EDGE('',*,*,#2239,.F.);
#3063=ORIENTED_EDGE('',*,*,#2235,.F.);
#3064=ORIENTED_EDGE('',*,*,#2290,.F.);
#3065=ORIENTED_EDGE('',*,*,#2291,.F.);
#3066=ORIENTED_EDGE('',*,*,#2233,.F.);
#3067=ORIENTED_EDGE('',*,*,#2238,.F.);
#3068=ORIENTED_EDGE('',*,*,#2237,.F.);
#3069=ORIENTED_EDGE('',*,*,#2243,.F.);
#3070=ORIENTED_EDGE('',*,*,#2242,.F.);
#3071=ORIENTED_EDGE('',*,*,#2248,.F.);
#3072=ORIENTED_EDGE('',*,*,#2247,.F.);
#3073=ORIENTED_EDGE('',*,*,#2253,.F.);
#3074=ORIENTED_EDGE('',*,*,#2252,.F.);
#3075=ORIENTED_EDGE('',*,*,#2257,.F.);
#3076=ORIENTED_EDGE('',*,*,#2256,.F.);
#3077=ORIENTED_EDGE('',*,*,#2261,.F.);
#3078=ORIENTED_EDGE('',*,*,#2266,.F.);
#3079=ORIENTED_EDGE('',*,*,#2265,.F.);
#3080=ORIENTED_EDGE('',*,*,#2270,.F.);
#3081=ORIENTED_EDGE('',*,*,#2274,.F.);
#3082=ORIENTED_EDGE('',*,*,#2273,.F.);
#3083=ORIENTED_EDGE('',*,*,#2281,.F.);
#3084=ORIENTED_EDGE('',*,*,#2280,.F.);
#3085=ORIENTED_EDGE('',*,*,#2292,.T.);
#3086=ORIENTED_EDGE('',*,*,#2293,.F.);
#3087=ORIENTED_EDGE('',*,*,#2228,.T.);
#3088=ORIENTED_EDGE('',*,*,#2227,.T.);
#3089=ORIENTED_EDGE('',*,*,#2287,.T.);
#3090=ORIENTED_EDGE('',*,*,#2286,.T.);
#3091=ORIENTED_EDGE('',*,*,#2225,.T.);
#3092=ORIENTED_EDGE('',*,*,#2224,.T.);
#3093=ORIENTED_EDGE('',*,*,#2220,.T.);
#3094=ORIENTED_EDGE('',*,*,#2219,.T.);
#3095=ORIENTED_EDGE('',*,*,#2215,.T.);
#3096=ORIENTED_EDGE('',*,*,#2214,.T.);
#3097=ORIENTED_EDGE('',*,*,#2210,.T.);
#3098=ORIENTED_EDGE('',*,*,#2209,.T.);
#3099=ORIENTED_EDGE('',*,*,#2205,.T.);
#3100=ORIENTED_EDGE('',*,*,#2204,.T.);
#3101=ORIENTED_EDGE('',*,*,#2200,.T.);
#3102=ORIENTED_EDGE('',*,*,#2199,.T.);
#3103=ORIENTED_EDGE('',*,*,#2195,.T.);
#3104=ORIENTED_EDGE('',*,*,#2194,.T.);
#3105=ORIENTED_EDGE('',*,*,#2190,.T.);
#3106=ORIENTED_EDGE('',*,*,#2189,.T.);
#3107=ORIENTED_EDGE('',*,*,#2185,.T.);
#3108=ORIENTED_EDGE('',*,*,#2184,.T.);
#3109=ORIENTED_EDGE('',*,*,#2180,.T.);
#3110=ORIENTED_EDGE('',*,*,#2179,.T.);
#3111=ORIENTED_EDGE('',*,*,#2294,.T.);
#3112=ORIENTED_EDGE('',*,*,#2291,.T.);
#3113=ORIENTED_EDGE('',*,*,#2178,.T.);
#3114=ORIENTED_EDGE('',*,*,#2288,.T.);
#3115=ORIENTED_EDGE('',*,*,#2290,.T.);
#3116=ORIENTED_EDGE('',*,*,#2234,.T.);
#3117=ORIENTED_EDGE('',*,*,#2294,.F.);
#3118=ORIENTED_EDGE('',*,*,#2295,.T.);
#3119=ORIENTED_EDGE('',*,*,#2296,.T.);
#3120=ORIENTED_EDGE('',*,*,#2295,.F.);
#3121=ORIENTED_EDGE('',*,*,#2296,.F.);
#3122=ORIENTED_EDGE('',*,*,#2293,.T.);
#3123=ORIENTED_EDGE('',*,*,#2292,.F.);
#3124=ORIENTED_EDGE('',*,*,#2279,.F.);
#3125=ORIENTED_EDGE('',*,*,#2289,.T.);
#3126=ORIENTED_EDGE('',*,*,#2229,.T.);
#3829=CYLINDRICAL_SURFACE('',#4455,6.11325);
#3830=CYLINDRICAL_SURFACE('',#4457,6.11325);
#3831=CYLINDRICAL_SURFACE('',#4458,6.11325);
#3832=CYLINDRICAL_SURFACE('',#4459,6.11325);
#3833=CYLINDRICAL_SURFACE('',#4460,6.11325);
#3834=CYLINDRICAL_SURFACE('',#4461,6.11325);
#3835=CYLINDRICAL_SURFACE('',#4462,6.11325);
#3836=CYLINDRICAL_SURFACE('',#4463,6.11325);
#3837=CYLINDRICAL_SURFACE('',#4464,6.11325);
#3838=CYLINDRICAL_SURFACE('',#4465,6.11325);
#3839=CYLINDRICAL_SURFACE('',#4466,6.11325);
#3840=CYLINDRICAL_SURFACE('',#4468,5.13675);
#3841=CYLINDRICAL_SURFACE('',#4470,5.13675);
#3842=CYLINDRICAL_SURFACE('',#4471,5.13675);
#3843=CYLINDRICAL_SURFACE('',#4472,5.13675);
#3844=CYLINDRICAL_SURFACE('',#4473,5.13675);
#3845=CYLINDRICAL_SURFACE('',#4474,5.13675);
#3846=CYLINDRICAL_SURFACE('',#4475,5.13675);
#3847=CYLINDRICAL_SURFACE('',#4476,5.13675);
#3848=CYLINDRICAL_SURFACE('',#4477,5.13675);
#3849=CYLINDRICAL_SURFACE('',#4478,5.13675);
#3850=CYLINDRICAL_SURFACE('',#4479,5.13675);
#3851=CYLINDRICAL_SURFACE('',#4481,5.13675);
#3852=CYLINDRICAL_SURFACE('',#4482,6.11325);
#3853=CYLINDRICAL_SURFACE('',#4485,12.);
#3986=ADVANCED_FACE('',(#656),#3829,.F.);
#3987=ADVANCED_FACE('',(#657),#3830,.F.);
#3988=ADVANCED_FACE('',(#658),#3831,.F.);
#3989=ADVANCED_FACE('',(#659),#3832,.F.);
#3990=ADVANCED_FACE('',(#660),#3833,.F.);
#3991=ADVANCED_FACE('',(#661),#3834,.F.);
#3992=ADVANCED_FACE('',(#662),#3835,.F.);
#3993=ADVANCED_FACE('',(#663),#3836,.F.);
#3994=ADVANCED_FACE('',(#664),#3837,.F.);
#3995=ADVANCED_FACE('',(#665),#3838,.F.);
#3996=ADVANCED_FACE('',(#666),#3839,.F.);
#3997=ADVANCED_FACE('',(#667),#3840,.F.);
#3998=ADVANCED_FACE('',(#668),#3841,.F.);
#3999=ADVANCED_FACE('',(#669),#3842,.F.);
#4000=ADVANCED_FACE('',(#670),#3843,.F.);
#4001=ADVANCED_FACE('',(#671),#3844,.F.);
#4002=ADVANCED_FACE('',(#672),#3845,.F.);
#4003=ADVANCED_FACE('',(#673),#3846,.F.);
#4004=ADVANCED_FACE('',(#674),#3847,.F.);
#4005=ADVANCED_FACE('',(#675),#3848,.F.);
#4006=ADVANCED_FACE('',(#676),#3849,.F.);
#4007=ADVANCED_FACE('',(#677),#3850,.F.);
#4008=ADVANCED_FACE('',(#678),#3851,.F.);
#4009=ADVANCED_FACE('',(#679),#3852,.F.);
#4010=ADVANCED_FACE('',(#680),#148,.F.);
#4011=ADVANCED_FACE('',(#681),#149,.F.);
#4012=ADVANCED_FACE('',(#682,#500),#552,.T.);
#4013=ADVANCED_FACE('',(#683),#3853,.T.);
#4014=ADVANCED_FACE('',(#684,#501),#553,.F.);
#4150=CLOSED_SHELL('',(#3986,#3987,#3988,#3989,#3990,#3991,#3992,#3993,
#3994,#3995,#3996,#3997,#3998,#3999,#4000,#4001,#4002,#4003,#4004,#4005,
#4006,#4007,#4008,#4009,#4010,#4011,#4012,#4013,#4014));
#4454=AXIS2_PLACEMENT_3D('',#5911,#4983,#4984);
#4455=AXIS2_PLACEMENT_3D('',#5912,#4985,#4986);
#4456=AXIS2_PLACEMENT_3D('',#5936,#4988,#4989);
#4457=AXIS2_PLACEMENT_3D('',#6002,#4990,#4991);
#4458=AXIS2_PLACEMENT_3D('',#6186,#4993,#4994);
#4459=AXIS2_PLACEMENT_3D('',#6585,#4996,#4997);
#4460=AXIS2_PLACEMENT_3D('',#6779,#4999,#5000);
#4461=AXIS2_PLACEMENT_3D('',#7102,#5002,#5003);
#4462=AXIS2_PLACEMENT_3D('',#7574,#5005,#5006);
#4463=AXIS2_PLACEMENT_3D('',#8049,#5008,#5009);
#4464=AXIS2_PLACEMENT_3D('',#8386,#5011,#5012);
#4465=AXIS2_PLACEMENT_3D('',#8784,#5014,#5015);
#4466=AXIS2_PLACEMENT_3D('',#9256,#5017,#5018);
#4467=AXIS2_PLACEMENT_3D('',#9278,#5020,#5021);
#4468=AXIS2_PLACEMENT_3D('',#9435,#5022,#5023);
#4469=AXIS2_PLACEMENT_3D('',#9509,#5025,#5026);
#4470=AXIS2_PLACEMENT_3D('',#9608,#5027,#5028);
#4471=AXIS2_PLACEMENT_3D('',#9845,#5030,#5031);
#4472=AXIS2_PLACEMENT_3D('',#10104,#5033,#5034);
#4473=AXIS2_PLACEMENT_3D('',#10370,#5036,#5037);
#4474=AXIS2_PLACEMENT_3D('',#10703,#5039,#5040);
#4475=AXIS2_PLACEMENT_3D('',#10843,#5042,#5043);
#4476=AXIS2_PLACEMENT_3D('',#11006,#5045,#5046);
#4477=AXIS2_PLACEMENT_3D('',#11346,#5048,#5049);
#4478=AXIS2_PLACEMENT_3D('',#11580,#5051,#5052);
#4479=AXIS2_PLACEMENT_3D('',#11805,#5054,#5055);
#4480=AXIS2_PLACEMENT_3D('',#11932,#5057,#5058);
#4481=AXIS2_PLACEMENT_3D('',#12019,#5059,#5060);
#4482=AXIS2_PLACEMENT_3D('',#12174,#5061,#5062);
#4483=AXIS2_PLACEMENT_3D('',#14143,#5063,#5064);
#4484=AXIS2_PLACEMENT_3D('',#14145,#5065,#5066);
#4485=AXIS2_PLACEMENT_3D('',#14146,#5067,#5068);
#4486=AXIS2_PLACEMENT_3D('',#14149,#5070,#5071);
#4487=AXIS2_PLACEMENT_3D('',#14150,#5072,#5073);
#4983=DIRECTION('axis',(0.,0.,1.));
#4984=DIRECTION('refdir',(1.,0.,0.));
#4985=DIRECTION('center_axis',(0.,0.,1.));
#4986=DIRECTION('ref_axis',(-0.608992685579745,0.793175837321315,0.));
#4987=DIRECTION('',(0.,0.,1.));
#4988=DIRECTION('center_axis',(0.,0.,-1.));
#4989=DIRECTION('ref_axis',(1.,6.25384645961333E-14,0.));
#4990=DIRECTION('center_axis',(0.,0.,1.));
#4991=DIRECTION('ref_axis',(-0.608992685579745,0.793175837321315,0.));
#4992=DIRECTION('',(0.,0.,1.));
#4993=DIRECTION('center_axis',(0.,0.,1.));
#4994=DIRECTION('ref_axis',(-0.608992685579745,0.793175837321315,0.));
#4995=DIRECTION('',(0.,0.,1.));
#4996=DIRECTION('center_axis',(0.,0.,1.));
#4997=DIRECTION('ref_axis',(-0.608992685579745,0.793175837321315,0.));
#4998=DIRECTION('',(0.,0.,1.));
#4999=DIRECTION('center_axis',(0.,0.,1.));
#5000=DIRECTION('ref_axis',(-0.608992685579745,0.793175837321315,0.));
#5001=DIRECTION('',(0.,0.,1.));
#5002=DIRECTION('center_axis',(0.,0.,1.));
#5003=DIRECTION('ref_axis',(-0.608992685579745,0.793175837321315,0.));
#5004=DIRECTION('',(0.,0.,1.));
#5005=DIRECTION('center_axis',(0.,0.,1.));
#5006=DIRECTION('ref_axis',(-0.608992685579745,0.793175837321315,0.));
#5007=DIRECTION('',(0.,0.,1.));
#5008=DIRECTION('center_axis',(0.,0.,1.));
#5009=DIRECTION('ref_axis',(-0.608992685579745,0.793175837321315,0.));
#5010=DIRECTION('',(0.,0.,1.));
#5011=DIRECTION('center_axis',(0.,0.,1.));
#5012=DIRECTION('ref_axis',(-0.608992685579745,0.793175837321315,0.));
#5013=DIRECTION('',(0.,0.,1.));
#5014=DIRECTION('center_axis',(0.,0.,1.));
#5015=DIRECTION('ref_axis',(-0.608992685579745,0.793175837321315,0.));
#5016=DIRECTION('',(0.,0.,1.));
#5017=DIRECTION('center_axis',(0.,0.,1.));
#5018=DIRECTION('ref_axis',(-0.608992685579745,0.793175837321315,0.));
#5019=DIRECTION('',(0.,0.,1.));
#5020=DIRECTION('center_axis',(0.,0.,1.));
#5021=DIRECTION('ref_axis',(1.,6.25384645961333E-14,0.));
#5022=DIRECTION('center_axis',(0.,0.,1.));
#5023=DIRECTION('ref_axis',(0.835515886164021,-0.549466290110277,0.));
#5024=DIRECTION('',(0.,0.,1.));
#5025=DIRECTION('center_axis',(0.,0.,1.));
#5026=DIRECTION('ref_axis',(1.,0.,0.));
#5027=DIRECTION('center_axis',(0.,0.,1.));
#5028=DIRECTION('ref_axis',(0.835515886164021,-0.549466290110277,0.));
#5029=DIRECTION('',(0.,0.,1.));
#5030=DIRECTION('center_axis',(0.,0.,1.));
#5031=DIRECTION('ref_axis',(0.835515886164021,-0.549466290110277,0.));
#5032=DIRECTION('',(0.,0.,1.));
#5033=DIRECTION('center_axis',(0.,0.,1.));
#5034=DIRECTION('ref_axis',(0.835515886164021,-0.549466290110277,0.));
#5035=DIRECTION('',(0.,0.,1.));
#5036=DIRECTION('center_axis',(0.,0.,1.));
#5037=DIRECTION('ref_axis',(0.835515886164021,-0.549466290110277,0.));
#5038=DIRECTION('',(0.,0.,1.));
#5039=DIRECTION('center_axis',(0.,0.,1.));
#5040=DIRECTION('ref_axis',(0.835515886164021,-0.549466290110277,0.));
#5041=DIRECTION('',(0.,0.,1.));
#5042=DIRECTION('center_axis',(0.,0.,1.));
#5043=DIRECTION('ref_axis',(0.835515886164021,-0.549466290110277,0.));
#5044=DIRECTION('',(0.,0.,1.));
#5045=DIRECTION('center_axis',(0.,0.,1.));
#5046=DIRECTION('ref_axis',(0.835515886164021,-0.549466290110277,0.));
#5047=DIRECTION('',(0.,0.,1.));
#5048=DIRECTION('center_axis',(0.,0.,1.));
#5049=DIRECTION('ref_axis',(0.835515886164021,-0.549466290110277,0.));
#5050=DIRECTION('',(0.,0.,1.));
#5051=DIRECTION('center_axis',(0.,0.,1.));
#5052=DIRECTION('ref_axis',(0.835515886164021,-0.549466290110277,0.));
#5053=DIRECTION('',(0.,0.,1.));
#5054=DIRECTION('center_axis',(0.,0.,1.));
#5055=DIRECTION('ref_axis',(0.835515886164021,-0.549466290110277,0.));
#5056=DIRECTION('',(0.,0.,1.));
#5057=DIRECTION('center_axis',(0.,0.,1.));
#5058=DIRECTION('ref_axis',(1.,0.,0.));
#5059=DIRECTION('center_axis',(0.,0.,1.));
#5060=DIRECTION('ref_axis',(0.835515886164021,-0.549466290110277,0.));
#5061=DIRECTION('center_axis',(0.,0.,1.));
#5062=DIRECTION('ref_axis',(-0.608992685579745,0.793175837321315,0.));
#5063=DIRECTION('center_axis',(0.,0.,1.));
#5064=DIRECTION('ref_axis',(1.,0.,0.));
#5065=DIRECTION('center_axis',(0.,0.,1.));
#5066=DIRECTION('ref_axis',(1.,0.,0.));
#5067=DIRECTION('center_axis',(0.,0.,1.));
#5068=DIRECTION('ref_axis',(1.,0.,0.));
#5069=DIRECTION('',(0.,0.,-1.));
#5070=DIRECTION('center_axis',(0.,0.,1.));
#5071=DIRECTION('ref_axis',(1.,0.,0.));
#5072=DIRECTION('center_axis',(0.,0.,1.));
#5073=DIRECTION('ref_axis',(1.,0.,0.));
#5911=CARTESIAN_POINT('',(0.,0.,0.));
#5912=CARTESIAN_POINT('Origin',(0.,0.,-3.86474103256053));
#5913=CARTESIAN_POINT('',(3.72323265631142,-4.84928321986684,18.4846156531836));
#5914=CARTESIAN_POINT('',(3.72309647396852,-4.84910580413568,18.6301376785985));
#5915=CARTESIAN_POINT('',(3.72292453512038,-4.84888218750453,-3.86474103256053));
#5916=CARTESIAN_POINT('',(-6.11311691712474,0.000135883258949067,19.7602589674395));
#5917=CARTESIAN_POINT('Ctrl Pts',(3.72309647396852,-4.84910580413568,18.6301376785985));
#5918=CARTESIAN_POINT('Ctrl Pts',(4.41515761247881,-4.31670063397706,18.6699250225774));
#5919=CARTESIAN_POINT('Ctrl Pts',(5.66534840628249,-2.84103380498307,18.7560271920921));
#5920=CARTESIAN_POINT('Ctrl Pts',(6.37224631075142,0.0728805235909378,18.8884441871425));
#5921=CARTESIAN_POINT('Ctrl Pts',(5.56076804884914,3.1126581338182,19.0273886637497));
#5922=CARTESIAN_POINT('Ctrl Pts',(3.39386814118494,5.39375839285986,19.1663331403569));
#5923=CARTESIAN_POINT('Ctrl Pts',(0.399713947821312,6.3600905721262,19.3052776169641));
#5924=CARTESIAN_POINT('Ctrl Pts',(-2.69185701515731,5.77626560449043,19.4442220935712));
#5925=CARTESIAN_POINT('Ctrl Pts',(-5.12731864093646,3.78429047467954,19.5831665701784));
#5926=CARTESIAN_POINT('Ctrl Pts',(-6.02625257748595,1.57494231132565,19.6885121948012));
#5927=CARTESIAN_POINT('Ctrl Pts',(-6.11338345835182,0.279275489936728,19.7475429938882));
#5928=CARTESIAN_POINT('Ctrl Pts',(-6.11311691712474,0.000135883258949067,
19.7602589674395));
#5929=CARTESIAN_POINT('',(-3.98497178445977,-4.63592767842203,20.));
#5930=CARTESIAN_POINT('Ctrl Pts',(-6.11311691712474,0.000135883258949067,
19.7602589674395));
#5931=CARTESIAN_POINT('Ctrl Pts',(-6.11241264708201,-0.73742229818409,19.7938578194239));
#5932=CARTESIAN_POINT('Ctrl Pts',(-5.79464560539175,-2.49228840649804,19.8737714969441));
#5933=CARTESIAN_POINT('Ctrl Pts',(-4.7558725986553,-3.97327325275336,19.9536851744643));
#5934=CARTESIAN_POINT('Ctrl Pts',(-3.98497178445977,-4.63592767842204,20.));
#5935=CARTESIAN_POINT('',(-1.13987236463957,-6.00604000609645,20.));
#5936=CARTESIAN_POINT('Origin',(0.,0.,20.));
#5937=CARTESIAN_POINT('',(-6.11324999831214,0.000143654567398843,19.6147410325606));
#5938=CARTESIAN_POINT('Ctrl Pts',(-6.11324999831214,0.000143654567399398,
19.6147410325606));
#5939=CARTESIAN_POINT('Ctrl Pts',(-6.11325396531437,-0.168672950627852,
19.622433450954));
#5940=CARTESIAN_POINT('Ctrl Pts',(-6.10626081651799,-0.337517076952744,
19.6301258693473));
#5941=CARTESIAN_POINT('Ctrl Pts',(-6.09228978312654,-0.505797153918474,
19.6378182877407));
#5942=CARTESIAN_POINT('Ctrl Pts',(-6.07831886348921,-0.674075860724036,
19.6455106435012));
#5943=CARTESIAN_POINT('Ctrl Pts',(-6.05737019381285,-0.841790205929373,
19.6532029992618));
#5944=CARTESIAN_POINT('Ctrl Pts',(-6.02951500037806,-1.0083523306444,19.6608953550224));
#5945=CARTESIAN_POINT('Ctrl Pts',(-6.0016621563273,-1.17490040704931,19.6685870619885));
#5946=CARTESIAN_POINT('Ctrl Pts',(-5.96690400636522,-1.34029613956119,19.6762787689545));
#5947=CARTESIAN_POINT('Ctrl Pts',(-5.9253631909807,-1.50396031113559,19.6839704759205));
#5948=CARTESIAN_POINT('Ctrl Pts',(-5.88381107602692,-1.66766900120639,19.6916642751174));
#5949=CARTESIAN_POINT('Ctrl Pts',(-5.8354726859269,-1.82964487612697,19.6993580743143));
#5950=CARTESIAN_POINT('Ctrl Pts',(-5.78052122573528,-1.98932147259408,19.7070518735112));
#5951=CARTESIAN_POINT('Ctrl Pts',(-5.72561165011813,-2.14887636189871,19.7147398084143));
#5952=CARTESIAN_POINT('Ctrl Pts',(-5.66409920055024,-2.30613517773545,19.7224277433174));
#5953=CARTESIAN_POINT('Ctrl Pts',(-5.59620555660258,-2.46055053407776,19.7301156782206));
#5954=CARTESIAN_POINT('Ctrl Pts',(-5.5279872642072,-2.61570426153742,19.7378403746817));
#5955=CARTESIAN_POINT('Ctrl Pts',(-5.4533004837073,-2.76804675380112,19.7455650711429));
#5956=CARTESIAN_POINT('Ctrl Pts',(-5.37240216219969,-2.91703969292365,19.753289767604));
#5957=CARTESIAN_POINT('Ctrl Pts',(-5.29151965130044,-3.0660035131601,19.7610129543658));
#5958=CARTESIAN_POINT('Ctrl Pts',(-5.20442817283899,-3.21161880811471,19.7687361411275));
#5959=CARTESIAN_POINT('Ctrl Pts',(-5.11143070011772,-3.35337170030315,19.7764593278892));
#5960=CARTESIAN_POINT('Ctrl Pts',(-5.01842967837498,-3.49513000214461,19.7841828093875));
#5961=CARTESIAN_POINT('Ctrl Pts',(-4.91952238188278,-3.63302533909178,19.7919062908858));
#5962=CARTESIAN_POINT('Ctrl Pts',(-4.81505563463806,-3.76657202212307,19.7996297723841));
#5963=CARTESIAN_POINT('Ctrl Pts',(-4.71059592941913,-3.90010970287171,19.8073527332482));
#5964=CARTESIAN_POINT('Ctrl Pts',(-4.60057771869083,-4.02929906666183,19.8150756941124));
#5965=CARTESIAN_POINT('Ctrl Pts',(-4.4853888174845,-4.15368664182615,19.8227986549765));
#5966=CARTESIAN_POINT('Ctrl Pts',(-4.37016933986405,-4.27810723515429,19.8305236658685));
#5967=CARTESIAN_POINT('Ctrl Pts',(-4.24977664299735,-4.3977232586767,19.8382486767604));
#5968=CARTESIAN_POINT('Ctrl Pts',(-4.12463684300107,-4.51211662923934,19.8459736876524));
#5969=CARTESIAN_POINT('Ctrl Pts',(-3.99997527616071,-4.626072835106,19.8536691767108));
#5970=CARTESIAN_POINT('Ctrl Pts',(-3.8706030776783,-4.73484604870215,19.8613646657693));
#5971=CARTESIAN_POINT('Ctrl Pts',(-3.73697560381574,-4.83806148152191,19.8690601548277));
#5972=CARTESIAN_POINT('Ctrl Pts',(-3.60312312372883,-4.94145071179636,19.8767686017974));
#5973=CARTESIAN_POINT('Ctrl Pts',(-3.46495174590424,-5.03930142897327,19.884477048767));
#5974=CARTESIAN_POINT('Ctrl Pts',(-3.32294240358536,-5.13126488742828,19.8921854957366));
#5975=CARTESIAN_POINT('Ctrl Pts',(-3.18096171618241,-5.22320978932126,19.8998923872812));
#5976=CARTESIAN_POINT('Ctrl Pts',(-3.03514487758738,-5.30926962909826,19.9075992788257));
#5977=CARTESIAN_POINT('Ctrl Pts',(-2.88600157662509,-5.38913912069613,19.9153061703702));
#5978=CARTESIAN_POINT('Ctrl Pts',(-2.73685534953163,-5.4690101793011,19.9230132131208));
#5979=CARTESIAN_POINT('Ctrl Pts',(-2.58438280939639,-5.54269049241582,19.9307202558714));
#5980=CARTESIAN_POINT('Ctrl Pts',(-2.42911864174319,-5.60992051519767,19.938427298622));
#5981=CARTESIAN_POINT('Ctrl Pts',(-2.27386281068899,-5.6771469281979,19.9461339275583));
#5982=CARTESIAN_POINT('Ctrl Pts',(-2.11581594560642,-5.7379236174449,19.9538405564947));
#5983=CARTESIAN_POINT('Ctrl Pts',(-1.95553330485704,-5.79203893772262,19.961547185431));
#5984=CARTESIAN_POINT('Ctrl Pts',(-1.79521365570525,-5.84616675293765,19.9692555937867));
#5985=CARTESIAN_POINT('Ctrl Pts',(-1.63265750219451,-5.89363002317083,19.9769640021423));
#5986=CARTESIAN_POINT('Ctrl Pts',(-1.46843667238002,-5.93426653443452,19.984672410498));
#5987=CARTESIAN_POINT('Ctrl Pts',(-1.35958975479145,-5.96120074855098,19.9897816069986));
#5988=CARTESIAN_POINT('Ctrl Pts',(-1.25001184602099,-5.98513689007408,19.9948908034993));
#5989=CARTESIAN_POINT('Ctrl Pts',(-1.13987236463957,-6.00604000609645,20.));
#5990=CARTESIAN_POINT('Ctrl Pts',(3.72323265631121,-4.849283219867,18.4846156531836));
#5991=CARTESIAN_POINT('Ctrl Pts',(4.50011870853811,-4.25236686515347,18.5292637239101));
#5992=CARTESIAN_POINT('Ctrl Pts',(5.78590765134228,-2.64892088143011,18.6202266201722));
#5993=CARTESIAN_POINT('Ctrl Pts',(6.35970660055813,0.406155425428676,18.7575043419702));
#5994=CARTESIAN_POINT('Ctrl Pts',(5.39030758885895,3.39932504877934,18.8964488185774));
#5995=CARTESIAN_POINT('Ctrl Pts',(3.10703361081359,5.56391738475428,19.0353932951846));
#5996=CARTESIAN_POINT('Ctrl Pts',(0.0664258911141372,6.37231582181012,19.1743377717918));
#5997=CARTESIAN_POINT('Ctrl Pts',(-2.99037070298137,5.62747898115738,19.313282248399));
#5998=CARTESIAN_POINT('Ctrl Pts',(-5.31827554245858,3.51095143602872,19.4522267250062));
#5999=CARTESIAN_POINT('Ctrl Pts',(-6.06432482748073,1.36134653944802,19.5527129863934));
#6000=CARTESIAN_POINT('Ctrl Pts',(-6.11361696706913,0.1725691056159,19.6068844222448));
#6001=CARTESIAN_POINT('Ctrl Pts',(-6.11344525254193,0.000143659155656239,
19.6147410325606));
#6002=CARTESIAN_POINT('Origin',(0.,0.,-3.86474103256053));
#6003=CARTESIAN_POINT('',(3.72262360719132,-4.84849058816371,16.7346163843233));
#6004=CARTESIAN_POINT('',(3.72292453512041,-4.84888218750451,16.8801307087023));
#6005=CARTESIAN_POINT('',(3.72292453512038,-4.84888218750453,-3.86474103256053));
#6006=CARTESIAN_POINT('',(-6.11324999839426,-0.000140116351456561,18.0102589674395));
#6007=CARTESIAN_POINT('Ctrl Pts',(3.72292453512041,-4.84888218750451,16.8801307087023));
#6008=CARTESIAN_POINT('Ctrl Pts',(3.85740053234976,-4.74563282608259,16.8878537136735));
#6009=CARTESIAN_POINT('Ctrl Pts',(3.98757637825864,-4.63678758882545,16.8955767186447));
#6010=CARTESIAN_POINT('Ctrl Pts',(4.1129955847594,-4.52273068867136,16.9032997236158));
#6011=CARTESIAN_POINT('Ctrl Pts',(4.23844518939046,-4.40864614429426,16.9110246004288));
#6012=CARTESIAN_POINT('Ctrl Pts',(4.3591356159556,-4.28934762584183,16.9187494772418));
#6013=CARTESIAN_POINT('Ctrl Pts',(4.47464552596157,-4.16525785270158,16.9264743540547));
#6014=CARTESIAN_POINT('Ctrl Pts',(4.55811883171226,-4.07558430371053,16.9320567409171));
#6015=CARTESIAN_POINT('Ctrl Pts',(4.63888747862407,-3.98340945604354,16.9376391277795));
#6016=CARTESIAN_POINT('Ctrl Pts',(4.71680498577818,-3.88890425295329,16.9432215146419));
#6017=CARTESIAN_POINT('Ctrl Pts',(4.82462521105301,-3.75813040431511,16.9509462767789));
#6018=CARTESIAN_POINT('Ctrl Pts',(4.92702260263085,-3.62284664644924,16.9586710389159));
#6019=CARTESIAN_POINT('Ctrl Pts',(5.02363219797993,-3.48352481000486,16.966395801053));
#6020=CARTESIAN_POINT('Ctrl Pts',(5.12022294781536,-3.34423015089788,16.9741190563302));
#6021=CARTESIAN_POINT('Ctrl Pts',(5.2110279737326,-3.20089924524164,16.9818423116075));
#6022=CARTESIAN_POINT('Ctrl Pts',(5.29572486081124,-3.05403401439567,16.9895655668848));
#6023=CARTESIAN_POINT('Ctrl Pts',(5.38042502101611,-2.9071631079168,16.9972891206286));
#6024=CARTESIAN_POINT('Ctrl Pts',(5.45901640827553,-2.75675787549156,17.0050126743725));
#6025=CARTESIAN_POINT('Ctrl Pts',(5.53122152199489,-2.60334669936998,17.0127362281163));
#6026=CARTESIAN_POINT('Ctrl Pts',(5.60342178608984,-2.44994582704192,17.0204592631111));
#6027=CARTESIAN_POINT('Ctrl Pts',(5.66923650003499,-2.29353970182158,17.0281822981059));
#6028=CARTESIAN_POINT('Ctrl Pts',(5.72843538734755,-2.13467879913685,17.0359053331007));
#6029=CARTESIAN_POINT('Ctrl Pts',(5.78765000714097,-1.97577567815672,17.0436304205412));
#6030=CARTESIAN_POINT('Ctrl Pts',(5.84024517420761,-1.81441677253815,17.0513555079816));
#6031=CARTESIAN_POINT('Ctrl Pts',(5.8860394562852,-1.65117082143364,17.0590805954221));
#6032=CARTESIAN_POINT('Ctrl Pts',(5.93165616231051,-1.48855788760185,17.0667757273644));
#6033=CARTESIAN_POINT('Ctrl Pts',(5.97052457975955,-1.32407282631843,17.0744708593068));
#6034=CARTESIAN_POINT('Ctrl Pts',(6.0025151204945,-1.15829089210565,17.0821659912491));
#6035=CARTESIAN_POINT('Ctrl Pts',(6.03462884078278,-0.991870614678331,17.0898907532913));
#6036=CARTESIAN_POINT('Ctrl Pts',(6.05982295693695,-0.824084510481028,17.0976155153334));
#6037=CARTESIAN_POINT('Ctrl Pts',(6.07800272341131,-0.655521515058598,17.1053402773756));
#6038=CARTESIAN_POINT('Ctrl Pts',(6.09617894358047,-0.486991401017124,17.1130635325577));
#6039=CARTESIAN_POINT('Ctrl Pts',(6.10734351031671,-0.317685013049303,17.1207867877398));
#6040=CARTESIAN_POINT('Ctrl Pts',(6.11145343651841,-0.148197354116924,17.1285100429219));
#6041=CARTESIAN_POINT('Ctrl Pts',(6.11556352154921,0.0212968547069763,17.1362335965711));
#6042=CARTESIAN_POINT('Ctrl Pts',(6.11261840885681,0.190972031784622,17.1439571502203));
#6043=CARTESIAN_POINT('Ctrl Pts',(6.10262721144545,0.360231426482325,17.1516807038694));
#6044=CARTESIAN_POINT('Ctrl Pts',(6.0926366850879,0.529479452956983,17.15940373877));
#6045=CARTESIAN_POINT('Ctrl Pts',(6.07560103973935,0.698311436529602,17.1671267736705));
#6046=CARTESIAN_POINT('Ctrl Pts',(6.05158142715187,0.866133819366549,17.1748498085711));
#6047=CARTESIAN_POINT('Ctrl Pts',(6.0275554311944,1.03400080210532,17.1825748959189));
#6048=CARTESIAN_POINT('Ctrl Pts',(5.99654180196561,1.20085733370429,17.1902999832667));
#6049=CARTESIAN_POINT('Ctrl Pts',(5.95865332050269,1.36611718698005,17.1980250706146));
#6050=CARTESIAN_POINT('Ctrl Pts',(5.92091175607884,1.5307362257554,17.2057202030285));
#6051=CARTESIAN_POINT('Ctrl Pts',(5.87634866192639,1.69377064972148,17.2134153354424));
#6052=CARTESIAN_POINT('Ctrl Pts',(5.82512546194225,1.85465331400023,17.2211104678563));
#6053=CARTESIAN_POINT('Ctrl Pts',(5.77370502927614,2.01615544991232,17.2288352300396));
#6054=CARTESIAN_POINT('Ctrl Pts',(5.71555485987603,2.17554641288183,17.2365599922229));
#6055=CARTESIAN_POINT('Ctrl Pts',(5.65087351920439,2.33226371417442,17.2442847544062));
#6056=CARTESIAN_POINT('Ctrl Pts',(5.58620479584162,2.48895044481747,17.2520080097297));
#6057=CARTESIAN_POINT('Ctrl Pts',(5.51500756418546,2.64296426168065,17.2597312650533));
#6058=CARTESIAN_POINT('Ctrl Pts',(5.43752874296885,2.79376211082612,17.2674545203768));
#6059=CARTESIAN_POINT('Ctrl Pts',(5.36004692757343,2.94456578757346,17.2751780741665));
#6060=CARTESIAN_POINT('Ctrl Pts',(5.27628317816278,3.09215296421023,17.2829016279562));
#6061=CARTESIAN_POINT('Ctrl Pts',(5.18653100007008,3.23600397833687,17.2906251817459));
#6062=CARTESIAN_POINT('Ctrl Pts',(5.09678485014641,3.37984533076787,17.2983482167862));
#6063=CARTESIAN_POINT('Ctrl Pts',(5.00105124421418,3.51995075395075,17.3060712518265));
#6064=CARTESIAN_POINT('Ctrl Pts',(4.89966785666064,3.65582828602583,17.3137942868669));
#6065=CARTESIAN_POINT('Ctrl Pts',(4.79825752584036,3.7917419284014,17.3215193743518));
#6066=CARTESIAN_POINT('Ctrl Pts',(4.69119460102203,3.92342517897288,17.3292444618368));
#6067=CARTESIAN_POINT('Ctrl Pts',(4.5788585864185,4.0504172140758,17.3369695493218));
#6068=CARTESIAN_POINT('Ctrl Pts',(4.46695818007797,4.1769168088868,17.3446646810357));
#6069=CARTESIAN_POINT('Ctrl Pts',(4.34982573743811,4.29876129357617,17.3523598127496));
#6070=CARTESIAN_POINT('Ctrl Pts',(4.22787434760758,4.41552987345141,17.3600549444634));
#6071=CARTESIAN_POINT('Ctrl Pts',(4.105453380092,4.53274807443797,17.3677797065254));
#6072=CARTESIAN_POINT('Ctrl Pts',(3.97813290208805,4.64489269664158,17.3755044685874));
#6073=CARTESIAN_POINT('Ctrl Pts',(3.84635639015853,4.75156480355542,17.3832292306495));
#6074=CARTESIAN_POINT('Ctrl Pts',(3.71460558370688,4.85821610207599,17.3909524858519));
#6075=CARTESIAN_POINT('Ctrl Pts',(3.57840072394426,4.95939681610103,17.3986757410543));
#6076=CARTESIAN_POINT('Ctrl Pts',(3.43821844952761,5.05474820894453,17.4063989962567));
#6077=CARTESIAN_POINT('Ctrl Pts',(3.29803075772491,5.15010328667122,17.4141225499267));
#6078=CARTESIAN_POINT('Ctrl Pts',(3.15386560350442,5.23962841090903,17.4218461035966));
#6079=CARTESIAN_POINT('Ctrl Pts',(3.00622934323705,5.32300767408432,17.4295696572666));
#6080=CARTESIAN_POINT('Ctrl Pts',(2.85860299888143,5.40638133713526,17.4372926921881));
#6081=CARTESIAN_POINT('Ctrl Pts',(2.70750629100869,5.48360980931102,17.4450157271096));
#6082=CARTESIAN_POINT('Ctrl Pts',(2.5534711092405,5.55442263937253,17.4527387620311));
#6083=CARTESIAN_POINT('Ctrl Pts',(2.39939499160698,5.6252542884106,17.4604638494001));
#6084=CARTESIAN_POINT('Ctrl Pts',(2.24237912686077,5.68966675387982,17.4681889367691));
#6085=CARTESIAN_POINT('Ctrl Pts',(2.08297723906201,5.74743694041523,17.4759140241381));
#6086=CARTESIAN_POINT('Ctrl Pts',(1.92419345337507,5.80498311533579,17.4836091564489));
#6087=CARTESIAN_POINT('Ctrl Pts',(1.76304242048026,5.85593835633561,17.4913042887597));
#6088=CARTESIAN_POINT('Ctrl Pts',(1.60008820533714,5.90013078648609,17.4989994210706));
#6089=CARTESIAN_POINT('Ctrl Pts',(1.43650654518176,5.94449337682453,17.5067241830071));
#6090=CARTESIAN_POINT('Ctrl Pts',(1.27104984546179,5.98205665631764,17.5144489449435));
#6091=CARTESIAN_POINT('Ctrl Pts',(1.10429839739535,6.01268248055808,17.52217370688));
#6092=CARTESIAN_POINT('Ctrl Pts',(0.93757947735708,6.04330233065145,17.5298969619553));
#6093=CARTESIAN_POINT('Ctrl Pts',(0.769566624453821,6.06698736855961,17.5376202170306));
#6094=CARTESIAN_POINT('Ctrl Pts',(0.600850017635141,6.08365061610279,17.545343472106));
#6095=CARTESIAN_POINT('Ctrl Pts',(0.432126890741339,6.10031450759933,17.5530670256475));
#6096=CARTESIAN_POINT('Ctrl Pts',(0.262700270504094,6.10995603063614,17.560790579189));
#6097=CARTESIAN_POINT('Ctrl Pts',(0.0931659410739898,6.11254003421849,17.5685141327306));
#6098=CARTESIAN_POINT('Ctrl Pts',(-0.0763570016617557,6.11512386424745,
17.5762371675232));
#6099=CARTESIAN_POINT('Ctrl Pts',(-0.245987322192782,6.11065111857973,17.5839602023159));
#6100=CARTESIAN_POINT('Ctrl Pts',(-0.415128562593811,6.09913877846855,17.5916832371085));
#6101=CARTESIAN_POINT('Ctrl Pts',(-0.584314753407991,6.08762337887617,17.5994083243492));
#6102=CARTESIAN_POINT('Ctrl Pts',(-0.753011287801984,6.06906466585127,17.6071334115899));
#6103=CARTESIAN_POINT('Ctrl Pts',(-0.920625190894922,6.04353165131032,17.6148584988305));
#6104=CARTESIAN_POINT('Ctrl Pts',(-1.08758916531128,6.01809764191181,17.6225536317796));
#6105=CARTESIAN_POINT('Ctrl Pts',(-1.25347858560841,5.98574339992642,17.6302487647287));
#6106=CARTESIAN_POINT('Ctrl Pts',(-1.41771590051754,5.94658786094343,17.6379438976778));
#6107=CARTESIAN_POINT('Ctrl Pts',(-1.5825856064655,5.90728155468817,17.6456686605141));
#6108=CARTESIAN_POINT('Ctrl Pts',(-1.74584884389252,5.86110752076091,17.6533934233504));
#6109=CARTESIAN_POINT('Ctrl Pts',(-1.90692995148701,5.80822207931324,17.6611181861868));
#6110=CARTESIAN_POINT('Ctrl Pts',(-2.0679796372646,5.75534695413841,17.6688414421668));
#6111=CARTESIAN_POINT('Ctrl Pts',(-2.22684774163247,5.69576313253178,17.6765646981468));
#6112=CARTESIAN_POINT('Ctrl Pts',(-2.38297440002704,5.62967659562392,17.6842879541268));
#6113=CARTESIAN_POINT('Ctrl Pts',(-2.53910709193791,5.56358750480117,17.6920115085721));
#6114=CARTESIAN_POINT('Ctrl Pts',(-2.69249783248372,5.49099531570375,17.6997350630174));
#6115=CARTESIAN_POINT('Ctrl Pts',(-2.84260663067095,5.41215420195744,17.7074586174627));
#6116=CARTESIAN_POINT('Ctrl Pts',(-2.99270534682735,5.33331838356056,17.7151816531569));
#6117=CARTESIAN_POINT('Ctrl Pts',(-3.13952228113979,5.24823462780715,17.722904688851));
#6118=CARTESIAN_POINT('Ctrl Pts',(-3.28254179254823,5.15720320936399,17.7306277245452));
#6119=CARTESIAN_POINT('Ctrl Pts',(-3.42559931210905,5.06614759886487,17.7383528126748));
#6120=CARTESIAN_POINT('Ctrl Pts',(-3.56485712344945,4.96914133566764,17.7460779008044));
#6121=CARTESIAN_POINT('Ctrl Pts',(-3.69982753705317,4.86652871753194,17.753802988934));
#6122=CARTESIAN_POINT('Ctrl Pts',(-3.83427450416188,4.7643140548731,17.7614981173843));
#6123=CARTESIAN_POINT('Ctrl Pts',(-3.96446704044143,4.65653666005199,17.7691932458347));
#6124=CARTESIAN_POINT('Ctrl Pts',(-4.08995488612825,4.54357729019059,17.776888374285));
#6125=CARTESIAN_POINT('Ctrl Pts',(-4.21592595010033,4.43018294566921,17.7846131345037));
#6126=CARTESIAN_POINT('Ctrl Pts',(-4.33720061386398,4.3115264549399,17.7923378947224));
#6127=CARTESIAN_POINT('Ctrl Pts',(-4.45334816253895,4.18802049967654,17.800062654941));
#6128=CARTESIAN_POINT('Ctrl Pts',(-4.5694730543394,4.06453863669032,17.8077859082926));
#6129=CARTESIAN_POINT('Ctrl Pts',(-4.68047260971287,3.93620942747956,17.8155091616442));
#6130=CARTESIAN_POINT('Ctrl Pts',(-4.78595374457437,3.80348160470042,17.8232324149957));
#6131=CARTESIAN_POINT('Ctrl Pts',(-4.89143895586818,3.67074865251133,17.8309559668207));
#6132=CARTESIAN_POINT('Ctrl Pts',(-4.99140511961486,3.53361699224015,17.8386795186457));
#6133=CARTESIAN_POINT('Ctrl Pts',(-5.08549965992524,3.3925681675392,17.8464030704707));
#6134=CARTESIAN_POINT('Ctrl Pts',(-5.17958788050771,3.25152881618485,17.8541261035542));
#6135=CARTESIAN_POINT('Ctrl Pts',(-5.26780509094031,3.10657309056353,17.8618491366377));
#6136=CARTESIAN_POINT('Ctrl Pts',(-5.34984215373234,2.95821136713531,17.8695721697212));
#6137=CARTESIAN_POINT('Ctrl Pts',(-5.43190101873005,2.80981021503058,17.8772972552813));
#6138=CARTESIAN_POINT('Ctrl Pts',(-5.50777629871879,2.65800153284127,17.8850223408414));
#6139=CARTESIAN_POINT('Ctrl Pts',(-5.57720446312307,2.50332098201971,17.8927474264016));
#6140=CARTESIAN_POINT('Ctrl Pts',(-5.64636350929811,2.3492400056834,17.9004425678984));
#6141=CARTESIAN_POINT('Ctrl Pts',(-5.70912523340383,2.19230968310618,17.9081377093953));
#6142=CARTESIAN_POINT('Ctrl Pts',(-5.7652764148881,2.03307978752312,17.9158328508922));
#6143=CARTESIAN_POINT('Ctrl Pts',(-5.82269509056864,1.87025561372202,17.9237016939378));
#6144=CARTESIAN_POINT('Ctrl Pts',(-5.87322249350811,1.7049664635386,17.9315705369834));
#6145=CARTESIAN_POINT('Ctrl Pts',(-5.91666753870068,1.5378136424761,17.939439380029));
#6146=CARTESIAN_POINT('Ctrl Pts',(-5.95928261330902,1.37385409521363,17.9471578973417));
#6147=CARTESIAN_POINT('Ctrl Pts',(-5.99508342088484,1.20810176362181,17.9548764146544));
#6148=CARTESIAN_POINT('Ctrl Pts',(-6.02394029638027,1.04113825601887,17.9625949319671));
#6149=CARTESIAN_POINT('Ctrl Pts',(-6.053640196018,0.869297080082928,17.9705389378791));
#6150=CARTESIAN_POINT('Ctrl Pts',(-6.07598418494458,0.696173225030384,17.9784829437912));
#6151=CARTESIAN_POINT('Ctrl Pts',(-6.09088764263035,0.522411032954849,17.9864269497033));
#6152=CARTESIAN_POINT('Ctrl Pts',(-6.10579110031611,0.348648840879286,17.9943709556154));
#6153=CARTESIAN_POINT('Ctrl Pts',(-6.11325399540428,0.17424867745491,18.0023149615274));
#6154=CARTESIAN_POINT('Ctrl Pts',(-6.11324999839426,-0.000140116351456561,
18.0102589674395));
#6155=CARTESIAN_POINT('Ctrl Pts',(-6.11298206926134,-0.000140309528671095,
18.0102589765195));
#6156=CARTESIAN_POINT('Ctrl Pts',(-6.11325663468543,-0.325885343511412,
18.0250984268461));
#6157=CARTESIAN_POINT('Ctrl Pts',(-6.00780900954066,-1.6681244042226,18.0862527027085));
#6158=CARTESIAN_POINT('Ctrl Pts',(-5.03941570755938,-3.90065628250744,18.1937218041066));
#6159=CARTESIAN_POINT('Ctrl Pts',(-2.55905445660959,-5.83627165166331,18.3326662807137));
#6160=CARTESIAN_POINT('Ctrl Pts',(0.545070549309975,-6.34930960566648,18.4716107573209));
#6161=CARTESIAN_POINT('Ctrl Pts',(2.66550147956873,-5.61097601765261,18.5707678899492));
#6162=CARTESIAN_POINT('Ctrl Pts',(3.60955744708097,-4.93645179362417,18.6236101970417));
#6163=CARTESIAN_POINT('Ctrl Pts',(3.72309647396852,-4.84910580413568,18.6301376785985));
#6164=CARTESIAN_POINT('',(-6.11277358809404,-6.86038334901315E-5,17.8647410325606));
#6165=CARTESIAN_POINT('Ctrl Pts',(-6.11277358809404,-6.86038334901315E-5,
17.8647410325606));
#6166=CARTESIAN_POINT('Ctrl Pts',(-6.11294404322182,-0.432525236900348,
17.8844398491494));
#6167=CARTESIAN_POINT('Ctrl Pts',(-5.96131848459198,-1.88163345335141,17.950453491274));
#6168=CARTESIAN_POINT('Ctrl Pts',(-4.82844309209128,-4.15896220843452,18.0627819589343));
#6169=CARTESIAN_POINT('Ctrl Pts',(-2.25021276710887,-5.96216166444017,18.2017264355415));
#6170=CARTESIAN_POINT('Ctrl Pts',(0.876501925825786,-6.31209741621358,18.3406709121487));
#6171=CARTESIAN_POINT('Ctrl Pts',(2.85349283772427,-5.50542282114631,18.4349673180294));
#6172=CARTESIAN_POINT('Ctrl Pts',(3.69423076344769,-4.87156667330043,18.4829488983743));
#6173=CARTESIAN_POINT('Ctrl Pts',(3.72323265631121,-4.849283219867,18.4846156531836));
#6174=CARTESIAN_POINT('Ctrl Pts',(3.72262360719331,-4.84849058816218,16.7346163843234));
#6175=CARTESIAN_POINT('Ctrl Pts',(4.17330897152384,-4.50222738608563,16.7605048127054));
#6176=CARTESIAN_POINT('Ctrl Pts',(5.29718827570009,-3.36293425993741,16.8327080666233));
#6177=CARTESIAN_POINT('Ctrl Pts',(6.31182959594577,-0.878428397354582,16.9512261460768));
#6178=CARTESIAN_POINT('Ctrl Pts',(5.96284817531305,2.24839296747554,17.090170622684));
#6179=CARTESIAN_POINT('Ctrl Pts',(4.16043569152321,4.82717351599487,17.2291150992912));
#6180=CARTESIAN_POINT('Ctrl Pts',(1.34392620390646,6.22934118968737,17.3680595758984));
#6181=CARTESIAN_POINT('Ctrl Pts',(-1.80016232579228,6.11312071668258,17.5070040525056));
#6182=CARTESIAN_POINT('Ctrl Pts',(-4.50546526677362,4.50684058160178,17.6459485291127));
#6183=CARTESIAN_POINT('Ctrl Pts',(-5.88472401532739,2.18550210418407,17.7651941891311));
#6184=CARTESIAN_POINT('Ctrl Pts',(-6.11254327805558,0.584244142210199,17.8381250236137));
#6185=CARTESIAN_POINT('Ctrl Pts',(-6.11277358809404,-6.86038334901315E-5,
17.8647410325606));
#6186=CARTESIAN_POINT('Origin',(0.,0.,-3.86474103256053));
#6187=CARTESIAN_POINT('',(3.72292453512039,-4.84888218750452,14.984609455652));
#6188=CARTESIAN_POINT('',(3.7229245351204,-4.84888218750451,15.1301297587947));
#6189=CARTESIAN_POINT('',(3.72292453512038,-4.84888218750453,-3.86474103256053));
#6190=CARTESIAN_POINT('',(-6.11324999939832,8.57698500699812E-5,16.2602589674827));
#6191=CARTESIAN_POINT('Ctrl Pts',(3.7229245351204,-4.84888218750451,15.1301297587947));
#6192=CARTESIAN_POINT('Ctrl Pts',(3.76245440720127,-4.81853153658144,15.132400945446));
#6193=CARTESIAN_POINT('Ctrl Pts',(3.8016112547446,-4.78769889512472,15.1346721320972));
#6194=CARTESIAN_POINT('Ctrl Pts',(3.84038328103664,-4.75639378281848,15.1369433187484));
#6195=CARTESIAN_POINT('Ctrl Pts',(3.9722547321136,-4.6499188063791,15.1446680808516));
#6196=CARTESIAN_POINT('Ctrl Pts',(4.09971876394751,-4.53793737361086,15.1523928429548));
#6197=CARTESIAN_POINT('Ctrl Pts',(4.22232314811218,-4.42083847198877,15.160117605058));
#6198=CARTESIAN_POINT('Ctrl Pts',(4.34490361599038,-4.30376241270545,15.1678408603013));
#6199=CARTESIAN_POINT('Ctrl Pts',(4.46262609868169,-4.18157109521427,15.1755641155446));
#6200=CARTESIAN_POINT('Ctrl Pts',(4.57507401088148,-4.05469152432794,15.183287370788));
#6201=CARTESIAN_POINT('Ctrl Pts',(4.68752626865271,-3.92780705015592,15.191010924498));
#6202=CARTESIAN_POINT('Ctrl Pts',(4.79470333487811,-3.79623419458935,15.1987344782081));
#6203=CARTESIAN_POINT('Ctrl Pts',(4.89622731440188,-3.66043489877978,15.2064580319181));
#6204=CARTESIAN_POINT('Ctrl Pts',(4.99774447511432,-3.52464472386738,15.2141810668792));
#6205=CARTESIAN_POINT('Ctrl Pts',(5.0936091191614,-3.38462893063772,15.2219041018403));
#6206=CARTESIAN_POINT('Ctrl Pts',(5.18348518087997,-3.24088058127691,15.2296271368015));
#6207=CARTESIAN_POINT('Ctrl Pts',(5.27338512774033,-3.09709402986718,15.2373522242088));
#6208=CARTESIAN_POINT('Ctrl Pts',(5.35729314207805,-2.94957320792683,15.2450773116162));
#6209=CARTESIAN_POINT('Ctrl Pts',(5.4349173433979,-2.79883887227055,15.2528023990235));
#6210=CARTESIAN_POINT('Ctrl Pts',(5.51224054411334,-2.64868903378612,15.2604975311342));
#6211=CARTESIAN_POINT('Ctrl Pts',(5.58332846394801,-2.49535085144685,15.2681926632449));
#6212=CARTESIAN_POINT('Ctrl Pts',(5.64793870418822,-2.33936186944917,15.2758877953556));
#6213=CARTESIAN_POINT('Ctrl Pts',(5.71279772520409,-2.18277225418048,15.2836125574588));
#6214=CARTESIAN_POINT('Ctrl Pts',(5.77115202657654,-2.02345591412792,15.291337319562));
#6215=CARTESIAN_POINT('Ctrl Pts',(5.82279059770343,-1.86197078865287,15.2990620816653));
#6216=CARTESIAN_POINT('Ctrl Pts',(5.87441909575774,-1.70051716388269,15.3067853369086));
#6217=CARTESIAN_POINT('Ctrl Pts',(5.91933438107333,-1.53689589953577,15.314508592152));
#6218=CARTESIAN_POINT('Ctrl Pts',(5.95737493080978,-1.37168126627841,15.3222318473954));
#6219=CARTESIAN_POINT('Ctrl Pts',(5.99541695063063,-1.20646024826962,15.3299554011054));
#6220=CARTESIAN_POINT('Ctrl Pts',(6.0265836282697,-1.0396460460813,15.3376789548155));
#6221=CARTESIAN_POINT('Ctrl Pts',(6.05076413028251,-0.871825098392158,15.3454025085256));
#6222=CARTESIAN_POINT('Ctrl Pts',(6.07494300822306,-0.704015422319585,15.3531255434867));
#6223=CARTESIAN_POINT('Ctrl Pts',(6.09213660433438,-0.535199449778643,15.3608485784478));
#6224=CARTESIAN_POINT('Ctrl Pts',(6.10228570595457,-0.365970935188203,15.368571613409));
#6225=CARTESIAN_POINT('Ctrl Pts',(6.1124375047638,-0.196697447031413,15.3762967008163));
#6226=CARTESIAN_POINT('Ctrl Pts',(6.11554104697018,-0.0270115141970811,
15.3840217882237));
#6227=CARTESIAN_POINT('Ctrl Pts',(6.11158916998146,0.142489928996134,15.3917468756311));
#6228=CARTESIAN_POINT('Ctrl Pts',(6.10765261704564,0.311334102469584,15.3994420077416));
#6229=CARTESIAN_POINT('Ctrl Pts',(6.09671530424912,0.479994903183618,15.4071371398522));
#6230=CARTESIAN_POINT('Ctrl Pts',(6.07882155181818,0.64788432891283,15.4148322719628));
#6231=CARTESIAN_POINT('Ctrl Pts',(6.06085889975761,0.816420210397759,15.422557034066));
#6232=CARTESIAN_POINT('Ctrl Pts',(6.03587973868905,0.984238451982329,15.4302817961692));
#6233=CARTESIAN_POINT('Ctrl Pts',(6.00396570920228,1.15074815890495,15.4380065582724));
#6234=CARTESIAN_POINT('Ctrl Pts',(5.97205790514611,1.31722538498324,15.4457298135157));
#6235=CARTESIAN_POINT('Ctrl Pts',(5.93321799156638,1.48239427465142,15.453453068759));
#6236=CARTESIAN_POINT('Ctrl Pts',(5.88757887892222,1.64567326859523,15.4611763240023));
#6237=CARTESIAN_POINT('Ctrl Pts',(5.84193800254567,1.80895857248757,15.4688998777124));
#6238=CARTESIAN_POINT('Ctrl Pts',(5.78949748281174,1.97035352822206,15.4766234314224));
#6239=CARTESIAN_POINT('Ctrl Pts',(5.73044056339439,2.1292901427246,15.4843469851324));
#6240=CARTESIAN_POINT('Ctrl Pts',(5.67138761050764,2.28821608232317,15.4920700200935));
#6241=CARTESIAN_POINT('Ctrl Pts',(5.6057192576342,2.44468371400129,15.4997930550547));
#6242=CARTESIAN_POINT('Ctrl Pts',(5.53366757806885,2.59814331743451,15.5075160900158));
#6243=CARTESIAN_POINT('Ctrl Pts',(5.46159675030623,2.75164370374437,15.5152411774231));
#6244=CARTESIAN_POINT('Ctrl Pts',(5.38313933882879,2.90213417640021,15.5229662648305));
#6245=CARTESIAN_POINT('Ctrl Pts',(5.29857464481329,3.04908712500015,15.5306913522378));
#6246=CARTESIAN_POINT('Ctrl Pts',(5.21433786430333,3.19547023937927,15.5383864843485));
#6247=CARTESIAN_POINT('Ctrl Pts',(5.12404126469462,3.33834296108946,15.5460816164593));
#6248=CARTESIAN_POINT('Ctrl Pts',(5.02800508219621,3.47721015411912,15.55377674857));
#6249=CARTESIAN_POINT('Ctrl Pts',(4.9315991137962,3.61661205322351,15.5615015106732));
#6250=CARTESIAN_POINT('Ctrl Pts',(4.82937510558569,3.75202687088283,15.5692262727764));
#6251=CARTESIAN_POINT('Ctrl Pts',(4.72168744963309,3.88297478622735,15.5769510348796));
#6252=CARTESIAN_POINT('Ctrl Pts',(4.6140208001795,4.01389715772259,15.5846742901229));
#6253=CARTESIAN_POINT('Ctrl Pts',(4.50089283079175,4.140354120929,15.5923975453663));
#6254=CARTESIAN_POINT('Ctrl Pts',(4.38269848859789,4.26189858168185,15.6001208006096));
#6255=CARTESIAN_POINT('Ctrl Pts',(4.26449957876029,4.38344773954444,15.6078443543197));
#6256=CARTESIAN_POINT('Ctrl Pts',(4.14123412242871,4.500083785097,15.6155679080297));
#6257=CARTESIAN_POINT('Ctrl Pts',(4.01333477515508,4.61139561792641,15.6232914617398));
#6258=CARTESIAN_POINT('Ctrl Pts',(3.88544401818213,4.7226999745479,15.6310144967009));
#6259=CARTESIAN_POINT('Ctrl Pts',(3.75292023218975,4.82868062598211,15.6387375316621));
#6260=CARTESIAN_POINT('Ctrl Pts',(3.61623020907674,4.92896587911306,15.6464605666232));
#6261=CARTESIAN_POINT('Ctrl Pts',(3.47950385971076,5.02927778369517,15.6541856540306));
#6262=CARTESIAN_POINT('Ctrl Pts',(3.33860931518214,5.12389107609201,15.6619107414379));
#6263=CARTESIAN_POINT('Ctrl Pts',(3.19404426139221,5.21247607368777,15.6696358288453));
#6264=CARTESIAN_POINT('Ctrl Pts',(3.05003978237056,5.30071756838848,15.6773309609559));
#6265=CARTESIAN_POINT('Ctrl Pts',(2.90239349252378,5.38297730096494,15.6850260930666));
#6266=CARTESIAN_POINT('Ctrl Pts',(2.75162348717553,5.4589736899278,15.6927212251772));
#6267=CARTESIAN_POINT('Ctrl Pts',(2.60027294414747,5.53526270186446,15.7004459872804));
#6268=CARTESIAN_POINT('Ctrl Pts',(2.44572096485065,5.6052670331009,15.7081707493836));
#6269=CARTESIAN_POINT('Ctrl Pts',(2.28850831054869,5.66873489193573,15.7158955114869));
#6270=CARTESIAN_POINT('Ctrl Pts',(2.13132632352709,5.7321903701729,15.7236187667302));
#6271=CARTESIAN_POINT('Ctrl Pts',(1.97148499082358,5.78911180164311,15.7313420219735));
#6272=CARTESIAN_POINT('Ctrl Pts',(1.8095450287456,5.83929553554554,15.7390652772168));
#6273=CARTESIAN_POINT('Ctrl Pts',(1.64759880846544,5.88948120880839,15.7467888309269));
#6274=CARTESIAN_POINT('Ctrl Pts',(1.48355409806413,5.9329285658752,15.7545123846369));
#6275=CARTESIAN_POINT('Ctrl Pts',(1.31798750613703,5.96948360381086,15.762235938347));
#6276=CARTESIAN_POINT('Ctrl Pts',(1.15243203441399,6.0060361865442,15.7699589733081));
#6277=CARTESIAN_POINT('Ctrl Pts',(0.985355195221883,6.03569730819591,15.7776820082692));
#6278=CARTESIAN_POINT('Ctrl Pts',(0.817344719570005,6.05836390223392,15.7854050432304));
#6279=CARTESIAN_POINT('Ctrl Pts',(0.649289594052713,6.08103652006521,15.7931301306377));
#6280=CARTESIAN_POINT('Ctrl Pts',(0.480300650282989,6.09671085130451,15.8008552180451));
#6281=CARTESIAN_POINT('Ctrl Pts',(0.310972649048222,6.10533550053098,15.8085803054525));
#6282=CARTESIAN_POINT('Ctrl Pts',(0.142301244982609,6.11392670626184,15.8162754375631));
#6283=CARTESIAN_POINT('Ctrl Pts',(-0.0267062782955295,6.11552282170934,
15.8239705696738));
#6284=CARTESIAN_POINT('Ctrl Pts',(-0.195460250937893,6.11012445477204,15.8316657017844));
#6285=CARTESIAN_POINT('Ctrl Pts',(-0.364864008257741,6.10470530150263,15.8393904638875));
#6286=CARTESIAN_POINT('Ctrl Pts',(-0.534072255290258,6.09223574530779,15.8471152259906));
#6287=CARTESIAN_POINT('Ctrl Pts',(-0.702489670939348,6.0727533973251,15.8548399880937));
#6288=CARTESIAN_POINT('Ctrl Pts',(-0.870874233610243,6.05327484974007,15.8625632433369));
#6289=CARTESIAN_POINT('Ctrl Pts',(-1.03846795807886,6.0267862763673,15.8702864985802));
#6290=CARTESIAN_POINT('Ctrl Pts',(-1.20468103221891,5.99337710920245,15.8780097538234));
#6291=CARTESIAN_POINT('Ctrl Pts',(-1.37090052969557,5.95996665093384,15.8857333075334));
#6292=CARTESIAN_POINT('Ctrl Pts',(-1.53573895859188,5.91963512226245,15.8934568612434));
#6293=CARTESIAN_POINT('Ctrl Pts',(-1.6986163043397,5.87252315560623,15.9011804149533));
#6294=CARTESIAN_POINT('Ctrl Pts',(-1.86148271050534,5.82541435320363,15.9089034499143));
#6295=CARTESIAN_POINT('Ctrl Pts',(-2.02238799263181,5.77152611223166,15.9166264848753));
#6296=CARTESIAN_POINT('Ctrl Pts',(-2.18076673873388,5.71104911498159,15.9243495198363));
#6297=CARTESIAN_POINT('Ctrl Pts',(-2.33918757500708,5.65055604558026,15.9320746072436));
#6298=CARTESIAN_POINT('Ctrl Pts',(-2.49508023648761,5.58347083206893,15.9397996946509));
#6299=CARTESIAN_POINT('Ctrl Pts',(-2.64789785912929,5.51003289374197,15.9475247820581));
#6300=CARTESIAN_POINT('Ctrl Pts',(-2.80012290632238,5.43687972309099,15.9552199141693));
#6301=CARTESIAN_POINT('Ctrl Pts',(-2.94929645279987,5.35742317179202,15.9629150462804));
#6302=CARTESIAN_POINT('Ctrl Pts',(-3.09490098491087,5.27194588895767,15.9706101783916));
#6303=CARTESIAN_POINT('Ctrl Pts',(-3.24106616511833,5.18613947711053,15.9783349404951));
#6304=CARTESIAN_POINT('Ctrl Pts',(-3.38368654368243,5.09423546024153,15.9860597025986));
#6305=CARTESIAN_POINT('Ctrl Pts',(-3.52225734787587,4.9965516846956,15.9937844647021));
#6306=CARTESIAN_POINT('Ctrl Pts',(-3.6608011212315,4.89888696420466,16.0015077199456));
#6307=CARTESIAN_POINT('Ctrl Pts',(-3.79529663756409,4.79544491719618,16.0092309751892));
#6308=CARTESIAN_POINT('Ctrl Pts',(-3.92526875433068,4.68658625961107,16.0169542304328));
#6309=CARTESIAN_POINT('Ctrl Pts',(-4.0552458938957,4.57772339516137,16.0246777841431));
#6310=CARTESIAN_POINT('Ctrl Pts',(-4.18069903859237,4.46344370171458,16.0324013378534));
#6311=CARTESIAN_POINT('Ctrl Pts',(-4.30118614514863,4.34414816820069,16.0401248915637));
#6312=CARTESIAN_POINT('Ctrl Pts',(-4.42166515924376,4.22486064711649,16.0478479265251));
#6313=CARTESIAN_POINT('Ctrl Pts',(-4.53717857744093,4.1005581831413,16.0555709614865));
#6314=CARTESIAN_POINT('Ctrl Pts',(-4.64732112470052,3.97167872900267,16.0632939964478));
#6315=CARTESIAN_POINT('Ctrl Pts',(-4.75749294305095,3.84276502431962,16.0710190838555));
#6316=CARTESIAN_POINT('Ctrl Pts',(-4.86229083058074,3.7092721385642,16.0787441712631));
#6317=CARTESIAN_POINT('Ctrl Pts',(-4.96134911688746,3.57167194782219,16.0864692586707));
#6318=CARTESIAN_POINT('Ctrl Pts',(-5.06002328838043,3.43460532447378,16.0941643907801));
#6319=CARTESIAN_POINT('Ctrl Pts',(-5.15300213578692,3.29346346521625,16.1018595228894));
#6320=CARTESIAN_POINT('Ctrl Pts',(-5.23996644446237,3.1487421652794,16.1095546549988));
#6321=CARTESIAN_POINT('Ctrl Pts',(-5.32726560793197,3.00346361810126,16.1172794171014));
#6322=CARTESIAN_POINT('Ctrl Pts',(-5.4085347159692,2.85452654155278,16.125004179204));
#6323=CARTESIAN_POINT('Ctrl Pts',(-5.48348258145226,2.70245154284211,16.1327289413066));
#6324=CARTESIAN_POINT('Ctrl Pts',(-5.55841582694723,2.55040620921468,16.1404521965494));
#6325=CARTESIAN_POINT('Ctrl Pts',(-5.62703015030143,2.39522445891001,16.1481754517922));
#6326=CARTESIAN_POINT('Ctrl Pts',(-5.68908089349989,2.23745036810083,16.1558987070349));
#6327=CARTESIAN_POINT('Ctrl Pts',(-5.75113403466138,2.07967018008122,16.1636222607444));
#6328=CARTESIAN_POINT('Ctrl Pts',(-5.80662296841791,1.91929774456649,16.1713458144538));
#6329=CARTESIAN_POINT('Ctrl Pts',(-5.8553513698642,1.75689666683316,16.1790693681633));
#6330=CARTESIAN_POINT('Ctrl Pts',(-5.90407649848985,1.59450649669339,16.1867924031238));
#6331=CARTESIAN_POINT('Ctrl Pts',(-5.94604191238515,1.43008826058703,16.1945154380843));
#6332=CARTESIAN_POINT('Ctrl Pts',(-5.98110125835133,1.26422043166854,16.2022384730448));
#6333=CARTESIAN_POINT('Ctrl Pts',(-6.01616992156442,1.09830852230657,16.2099635604516));
#6334=CARTESIAN_POINT('Ctrl Pts',(-6.04432878169025,0.930946560175674,16.2176886478584));
#6335=CARTESIAN_POINT('Ctrl Pts',(-6.06548249332253,0.762723859399947,16.2254137352652));
#6336=CARTESIAN_POINT('Ctrl Pts',(-6.08655417796907,0.59515346973237,16.2331088673788));
#6337=CARTESIAN_POINT('Ctrl Pts',(-6.100674937807,0.426729318635894,16.2408039994924));
#6338=CARTESIAN_POINT('Ctrl Pts',(-6.10780166506172,0.258039498467358,16.2484991316059));
#6339=CARTESIAN_POINT('Ctrl Pts',(-6.11143206158205,0.172107918056641,16.2524190768838));
#6340=CARTESIAN_POINT('Ctrl Pts',(-6.11324879259944,0.0860994634106513,
16.2563390221616));
#6341=CARTESIAN_POINT('Ctrl Pts',(-6.1132499993983,8.57707989032423E-5,
16.2602589674395));
#6342=CARTESIAN_POINT('Ctrl Pts',(-6.11324999939832,8.5769850077377E-5,
16.2602589674827));
#6343=CARTESIAN_POINT('Ctrl Pts',(-6.11325237018008,-0.168891809259724,
16.2679598676903));
#6344=CARTESIAN_POINT('Ctrl Pts',(-6.10624428268917,-0.337901014722052,
16.2756607678979));
#6345=CARTESIAN_POINT('Ctrl Pts',(-6.09224393255344,-0.506349117473063,
16.2833616681055));
#6346=CARTESIAN_POINT('Ctrl Pts',(-6.07824623187471,-0.674765342735428,
16.2910611109779));
#6347=CARTESIAN_POINT('Ctrl Pts',(-6.05725893532342,-0.842620357625315,
16.2987605538503));
#6348=CARTESIAN_POINT('Ctrl Pts',(-6.02935220866743,-1.00932527281206,16.3064599967226));
#6349=CARTESIAN_POINT('Ctrl Pts',(-6.00144454055709,-1.17603581191415,16.3141596993414));
#6350=CARTESIAN_POINT('Ctrl Pts',(-5.9666170251134,-1.34159585676452,16.3218594019603));
#6351=CARTESIAN_POINT('Ctrl Pts',(-5.92499130018901,-1.5054247424513,16.3295591045791));
#6352=CARTESIAN_POINT('Ctrl Pts',(-5.88336701750354,-1.66924795183102,16.3372585404204));
#6353=CARTESIAN_POINT('Ctrl Pts',(-5.83494507717228,-1.83133981152082,16.3449579762616));
#6354=CARTESIAN_POINT('Ctrl Pts',(-5.77989758545023,-1.99113270883853,16.3526574121029));
#6355=CARTESIAN_POINT('Ctrl Pts',(-5.7248371957853,-2.1509630465481,16.360358651966));
#6356=CARTESIAN_POINT('Ctrl Pts',(-5.66314825791892,-2.3084930423638,16.3680598918293));
#6357=CARTESIAN_POINT('Ctrl Pts',(-5.59505208858061,-2.46317228154462,16.3757611316925));
#6358=CARTESIAN_POINT('Ctrl Pts',(-5.56061902266852,-2.54138637919064,16.3796552905327));
#6359=CARTESIAN_POINT('Ctrl Pts',(-5.5245484894734,-2.61887188728961,16.3835494493729));
#6360=CARTESIAN_POINT('Ctrl Pts',(-5.48687372986159,-2.69555972574432,16.3874436082131));
#6361=CARTESIAN_POINT('Ctrl Pts',(-5.41213909083035,-2.84768379990036,16.3951683703152));
#6362=CARTESIAN_POINT('Ctrl Pts',(-5.33106083836323,-2.99672486023318,16.4028931324173));
#6363=CARTESIAN_POINT('Ctrl Pts',(-5.24391852388584,-3.14215596006101,16.4106178945194));
#6364=CARTESIAN_POINT('Ctrl Pts',(-5.15679320815288,-3.28755869082253,16.4183411497616));
#6365=CARTESIAN_POINT('Ctrl Pts',(-5.06360635353548,-3.42935259449848,16.4260644050038));
#6366=CARTESIAN_POINT('Ctrl Pts',(-4.96468245966836,-3.56703709500775,16.4337876602461));
#6367=CARTESIAN_POINT('Ctrl Pts',(-4.86575474286792,-3.70472691636161,16.441511213955));
#6368=CARTESIAN_POINT('Ctrl Pts',(-4.76108972486681,-3.83830675707666,16.4492347676639));
#6369=CARTESIAN_POINT('Ctrl Pts',(-4.65105452122077,-3.96730606370769,16.4569583213729));
#6370=CARTESIAN_POINT('Ctrl Pts',(-4.54102670803836,-4.09629670615987,16.4646813563329));
#6371=CARTESIAN_POINT('Ctrl Pts',(-4.42562963670314,-4.22070718904318,16.4724043912929));
#6372=CARTESIAN_POINT('Ctrl Pts',(-4.30527001059718,-4.3401008857344,16.4801274262529));
#6373=CARTESIAN_POINT('Ctrl Pts',(-4.18487839814579,-4.45952631206909,16.4878525136592));
#6374=CARTESIAN_POINT('Ctrl Pts',(-4.05952181920495,-4.573932063167,16.4955776010655));
#6375=CARTESIAN_POINT('Ctrl Pts',(-3.92964374318109,-4.68291849322382,16.5033026884717));
#6376=CARTESIAN_POINT('Ctrl Pts',(-3.8002692906423,-4.79148231057025,16.5109978205879));
#6377=CARTESIAN_POINT('Ctrl Pts',(-3.66640860424335,-4.8946685847889,16.5186929527041));
#6378=CARTESIAN_POINT('Ctrl Pts',(-3.52853245062451,-4.99212222480478,16.5263880848203));
#6379=CARTESIAN_POINT('Ctrl Pts',(-3.39012540701131,-5.08995110855236,16.5341128469236));
#6380=CARTESIAN_POINT('Ctrl Pts',(-3.24762287481692,-5.18203774718436,16.5418376090268));
#6381=CARTESIAN_POINT('Ctrl Pts',(-3.1015224421497,-5.2680531606412,16.54956237113));
#6382=CARTESIAN_POINT('Ctrl Pts',(-2.95545050911474,-5.35405179517681,16.5572856263734));
#6383=CARTESIAN_POINT('Ctrl Pts',(-2.80578234896859,-5.43398140695962,16.5650088816168));
#6384=CARTESIAN_POINT('Ctrl Pts',(-2.65304240354883,-5.50755767718068,16.5727321368602));
#6385=CARTESIAN_POINT('Ctrl Pts',(-2.50029655546385,-5.58113679077117,16.5804556905702));
#6386=CARTESIAN_POINT('Ctrl Pts',(-2.34447896835884,-5.64836193038159,16.5881792442803));
#6387=CARTESIAN_POINT('Ctrl Pts',(-2.18613714251705,-5.70899552956625,16.5959027979904));
#6388=CARTESIAN_POINT('Ctrl Pts',(-2.02780595163096,-5.76962505632318,16.6036258329516));
#6389=CARTESIAN_POINT('Ctrl Pts',(-1.86695115728414,-5.82366381526525,16.6113488679128));
#6390=CARTESIAN_POINT('Ctrl Pts',(-1.70413879127973,-5.87092297194876,16.6190719028739));
#6391=CARTESIAN_POINT('Ctrl Pts',(-1.54128315684185,-5.91819468805713,16.6267969902813));
#6392=CARTESIAN_POINT('Ctrl Pts',(-1.37646921515672,-5.95868311112467,16.6345220776887));
#6393=CARTESIAN_POINT('Ctrl Pts',(-1.21027759052793,-5.99224947047149,16.6422471650961));
#6394=CARTESIAN_POINT('Ctrl Pts',(-1.0447304012558,-6.02568567073957,16.6499422972066));
#6395=CARTESIAN_POINT('Ctrl Pts',(-0.877816506823421,-6.05225336453254,
16.657637429317));
#6396=CARTESIAN_POINT('Ctrl Pts',(-0.710119185660943,-6.07186596563661,
16.6653325614275));
#6397=CARTESIAN_POINT('Ctrl Pts',(-0.541776148346675,-6.0915540847825,16.6730573235348));
#6398=CARTESIAN_POINT('Ctrl Pts',(-0.372584013597159,-6.10424038706862,
16.6807820856421));
#6399=CARTESIAN_POINT('Ctrl Pts',(-0.203137120202453,-6.10987404722027,
16.6885068477494));
#6400=CARTESIAN_POINT('Ctrl Pts',(-0.0337232806044481,-6.11550660842078,
16.6962301029969));
#6401=CARTESIAN_POINT('Ctrl Pts',(0.135944901919463,-6.11408926207646,16.7039533582444));
#6402=CARTESIAN_POINT('Ctrl Pts',(0.305270874867088,-6.1056232487321,16.7116766134919));
#6403=CARTESIAN_POINT('Ctrl Pts',(0.474603391450264,-6.09715690821698,16.7194001672061));
#6404=CARTESIAN_POINT('Ctrl Pts',(0.643593355273245,-6.08164136748782,16.7271237209203));
#6405=CARTESIAN_POINT('Ctrl Pts',(0.811646333308634,-6.05912995339485,16.7348472746345));
#6406=CARTESIAN_POINT('Ctrl Pts',(0.979688024142844,-6.03662005127067,16.7425703095997));
#6407=CARTESIAN_POINT('Ctrl Pts',(1.14679254097663,-6.00711525816716,16.750293344565));
#6408=CARTESIAN_POINT('Ctrl Pts',(1.31237249258622,-5.97072055979871,16.7580163795302));
#6409=CARTESIAN_POINT('Ctrl Pts',(1.47799644813229,-5.93431618930523,16.7657414669417));
#6410=CARTESIAN_POINT('Ctrl Pts',(1.64209471861648,-5.89101832064699,16.7734665543531));
#6411=CARTESIAN_POINT('Ctrl Pts',(1.80409105072818,-5.84098288331531,16.7811916417646));
#6412=CARTESIAN_POINT('Ctrl Pts',(1.96545921490648,-5.79114146677939,16.7888867738546));
#6413=CARTESIAN_POINT('Ctrl Pts',(2.12474142420005,-5.73461476372079,16.7965819059447));
#6414=CARTESIAN_POINT('Ctrl Pts',(2.2813840612205,-5.67160579798253,16.8042770380347));
#6415=CARTESIAN_POINT('Ctrl Pts',(2.43863116068549,-5.60835368929046,16.8120018645837));
#6416=CARTESIAN_POINT('Ctrl Pts',(2.59327395733649,-5.53854675995458,16.8197266911327));
#6417=CARTESIAN_POINT('Ctrl Pts',(2.74476621688423,-5.46242473423213,16.8274515176816));
#6418=CARTESIAN_POINT('Ctrl Pts',(2.89622663670497,-5.38631870737674,16.8351747206733));
#6419=CARTESIAN_POINT('Ctrl Pts',(3.04453755791828,-5.30390037524132,16.842897923665));
#6420=CARTESIAN_POINT('Ctrl Pts',(3.18917573645277,-5.21545622975794,16.8506211266566));
#6421=CARTESIAN_POINT('Ctrl Pts',(3.33380274604764,-5.12701891391892,16.8583437332636));
#6422=CARTESIAN_POINT('Ctrl Pts',(3.47475730820949,-5.03255687782452,16.8660663398706));
#6423=CARTESIAN_POINT('Ctrl Pts',(3.6115431297739,-4.93240121890778,16.8737889464777));
#6424=CARTESIAN_POINT('Ctrl Pts',(3.64898571879469,-4.90498545949619,16.8759028672192));
#6425=CARTESIAN_POINT('Ctrl Pts',(3.68611611652612,-4.87714333293649,16.8780167879608));
#6426=CARTESIAN_POINT('Ctrl Pts',(3.72292453512041,-4.84888218750451,16.8801307087023));
#6427=CARTESIAN_POINT('',(-6.11329971010691,-2.18371950135767E-5,16.1147410325606));
#6428=CARTESIAN_POINT('Ctrl Pts',(-6.11376907689637,-2.18388716277662E-5,
16.1147410325606));
#6429=CARTESIAN_POINT('Ctrl Pts',(-6.11377325293236,-0.0206356155618927,
16.1156804505183));
#6430=CARTESIAN_POINT('Ctrl Pts',(-6.10863870970093,-1.05753985300389,16.1629346940117));
#6431=CARTESIAN_POINT('Ctrl Pts',(-5.5648651016231,-3.10533503802479,16.2565037630409));
#6432=CARTESIAN_POINT('Ctrl Pts',(-3.400970216456,-5.38926997694936,16.3954482396481));
#6433=CARTESIAN_POINT('Ctrl Pts',(-0.40809635818025,-6.35958227087845,16.5343927162552));
#6434=CARTESIAN_POINT('Ctrl Pts',(2.10807756387106,-5.88779407064529,16.6474487644803));
#6435=CARTESIAN_POINT('Ctrl Pts',(3.36702541840832,-5.12169796795855,16.7141899871697));
#6436=CARTESIAN_POINT('Ctrl Pts',(3.72262360719331,-4.84849058816218,16.7346163843234));
#6437=CARTESIAN_POINT('Ctrl Pts',(3.72292453512039,-4.84888218750452,14.984609455652));
#6438=CARTESIAN_POINT('Ctrl Pts',(3.84706716304671,-4.75356668642837,14.9917407949601));
#6439=CARTESIAN_POINT('Ctrl Pts',(3.96753323261942,-4.65349207330933,14.9988721342681));
#6440=CARTESIAN_POINT('Ctrl Pts',(4.08396494501409,-4.54896206737274,15.0060034735762));
#6441=CARTESIAN_POINT('Ctrl Pts',(4.21008533287738,-4.43573376710187,15.0137282356794));
#6442=CARTESIAN_POINT('Ctrl Pts',(4.33151625523934,-4.31723713512184,15.0214529977826));
#6443=CARTESIAN_POINT('Ctrl Pts',(4.44782645370979,-4.19388428550185,15.0291777598858));
#6444=CARTESIAN_POINT('Ctrl Pts',(4.56411396369235,-4.07055549817109,15.0369010151291));
#6445=CARTESIAN_POINT('Ctrl Pts',(4.67528252564377,-3.94237261384261,15.0446242703725));
#6446=CARTESIAN_POINT('Ctrl Pts',(4.78093846444182,-3.80978384711267,15.0523475256158));
#6447=CARTESIAN_POINT('Ctrl Pts',(4.88659848633455,-3.67718995646359,15.0600710793258));
#6448=CARTESIAN_POINT('Ctrl Pts',(4.98674525817353,-3.54019008808067,15.0677946330359));
#6449=CARTESIAN_POINT('Ctrl Pts',(5.08102556976984,-3.39926532089584,15.0755181867459));
#6450=CARTESIAN_POINT('Ctrl Pts',(5.17529954907249,-3.25835001885802,15.0832412217071));
#6451=CARTESIAN_POINT('Ctrl Pts',(5.26370768038889,-3.11351060899576,15.0909642566682));
#6452=CARTESIAN_POINT('Ctrl Pts',(5.34594015390214,-2.96525706025578,15.0986872916293));
#6453=CARTESIAN_POINT('Ctrl Pts',(5.42819448122435,-2.8169641121813,15.1064123790367));
#6454=CARTESIAN_POINT('Ctrl Pts',(5.5042697154448,-2.66525548845014,15.114137466444));
#6455=CARTESIAN_POINT('Ctrl Pts',(5.57390162030798,-2.51066650306807,15.1218625538514));
#6456=CARTESIAN_POINT('Ctrl Pts',(5.64326351601011,-2.35667696189673,15.1295576859621));
#6457=CARTESIAN_POINT('Ctrl Pts',(5.70623186484387,-2.19982965540261,15.1372528180727));
#6458=CARTESIAN_POINT('Ctrl Pts',(5.76259272283903,-2.04067407323725,15.1449479501834));
#6459=CARTESIAN_POINT('Ctrl Pts',(5.81917059748546,-1.88090566485343,15.1526727122866));
#6460=CARTESIAN_POINT('Ctrl Pts',(5.86911000608853,-1.71875457430929,15.1603974743898));
#6461=CARTESIAN_POINT('Ctrl Pts',(5.91222941682117,-1.55478901635378,15.168122236493));
#6462=CARTESIAN_POINT('Ctrl Pts',(5.95534041630324,-1.39085544295861,15.1758454917363));
#6463=CARTESIAN_POINT('Ctrl Pts',(5.99163399192148,-1.22510841471985,15.1835687469797));
#6464=CARTESIAN_POINT('Ctrl Pts',(6.02097888624547,-1.05812986626704,15.191292002223));
#6465=CARTESIAN_POINT('Ctrl Pts',(6.0503249146087,-0.891144864895214,15.199015555933));
#6466=CARTESIAN_POINT('Ctrl Pts',(6.07272166557029,-0.722928559523004,15.2067391096431));
#6467=CARTESIAN_POINT('Ctrl Pts',(6.08808913827344,-0.554072384203525,15.2144626633531));
#6468=CARTESIAN_POINT('Ctrl Pts',(6.10345557882736,-0.385227550031262,15.2221856983143));
#6469=CARTESIAN_POINT('Ctrl Pts',(6.11179365718794,-0.215743247568319,15.2299087332754));
#6470=CARTESIAN_POINT('Ctrl Pts',(6.11307530532601,-0.0462155159367491,
15.2376317682365));
#6471=CARTESIAN_POINT('Ctrl Pts',(6.11435729407032,0.123357268780197,15.2453568556439));
#6472=CARTESIAN_POINT('Ctrl Pts',(6.10857910072673,0.292973188604178,15.2530819430512));
#6473=CARTESIAN_POINT('Ctrl Pts',(6.09576480241753,0.462035751979778,15.2608070304586));
#6474=CARTESIAN_POINT('Ctrl Pts',(6.08300019365714,0.630442747466239,15.2685021625693));
#6475=CARTESIAN_POINT('Ctrl Pts',(6.06325400597843,0.798300361477343,15.2761972946799));
#6476=CARTESIAN_POINT('Ctrl Pts',(6.03660126151578,0.965023715753177,15.2838924267906));
#6477=CARTESIAN_POINT('Ctrl Pts',(6.00984589105432,1.13238903584166,15.2916171888938));
#6478=CARTESIAN_POINT('Ctrl Pts',(5.97612116543257,1.29867061503148,15.2993419509969));
#6479=CARTESIAN_POINT('Ctrl Pts',(5.93553952736822,1.46328263898312,15.3070667131001));
#6480=CARTESIAN_POINT('Ctrl Pts',(5.89496580551407,1.62786255226983,15.3147899683434));
#6481=CARTESIAN_POINT('Ctrl Pts',(5.84753791596166,1.79077325263618,15.3225132235868));
#6482=CARTESIAN_POINT('Ctrl Pts',(5.79341901268092,1.95144093069898,15.3302364788301));
#6483=CARTESIAN_POINT('Ctrl Pts',(5.73929801796461,2.1121148177955,15.3379600325402));
#6484=CARTESIAN_POINT('Ctrl Pts',(5.67848558950548,2.27054520753042,15.3456835862502));
#6485=CARTESIAN_POINT('Ctrl Pts',(5.61119443581084,2.42617447147263,15.3534071399603));
#6486=CARTESIAN_POINT('Ctrl Pts',(5.54390780169532,2.58179328264751,15.3611301749214));
#6487=CARTESIAN_POINT('Ctrl Pts',(5.4701434389292,2.73461105359685,15.3688532098825));
#6488=CARTESIAN_POINT('Ctrl Pts',(5.3901618627911,2.88409095824185,15.3765762448437));
#6489=CARTESIAN_POINT('Ctrl Pts',(5.31015903103472,3.03361058813293,15.384301332251));
#6490=CARTESIAN_POINT('Ctrl Pts',(5.22393583198312,3.1797902984944,15.3920264196584));
#6491=CARTESIAN_POINT('Ctrl Pts',(5.13179878739104,3.3221178137194,15.3997515070657));
#6492=CARTESIAN_POINT('Ctrl Pts',(5.04001901933984,3.46389343060063,15.4074466391764));
#6493=CARTESIAN_POINT('Ctrl Pts',(4.94237138475036,3.60184642972867,15.4151417712871));
#6494=CARTESIAN_POINT('Ctrl Pts',(4.83920158538215,3.73549910701835,15.4228369033977));
#6495=CARTESIAN_POINT('Ctrl Pts',(4.73563453222546,3.86966641196766,15.4305616655009));
#6496=CARTESIAN_POINT('Ctrl Pts',(4.6264659997075,3.99954771240799,15.4382864276041));
#6497=CARTESIAN_POINT('Ctrl Pts',(4.51207499742677,4.12468238535965,15.4460111897073));
#6498=CARTESIAN_POINT('Ctrl Pts',(4.39770630925843,4.24979264844428,15.4537344449506));
#6499=CARTESIAN_POINT('Ctrl Pts',(4.27811739778417,4.37015789780446,15.4614577001939));
#6500=CARTESIAN_POINT('Ctrl Pts',(4.15372605995467,4.48535231407227,15.4691809554373));
#6501=CARTESIAN_POINT('Ctrl Pts',(4.02932991499747,4.60055118205093,15.4769045091473));
#6502=CARTESIAN_POINT('Ctrl Pts',(3.900131202141,4.71057859882912,15.4846280628574));
#6503=CARTESIAN_POINT('Ctrl Pts',(3.76658349202819,4.81504666229526,15.4923516165674));
#6504=CARTESIAN_POINT('Ctrl Pts',(3.63304475158556,4.91950770921224,15.5000746515285));
#6505=CARTESIAN_POINT('Ctrl Pts',(3.49515784807595,5.01840995475133,15.5077976864897));
#6506=CARTESIAN_POINT('Ctrl Pts',(3.35340838006248,5.11140663604714,15.5155207214508));
#6507=CARTESIAN_POINT('Ctrl Pts',(3.21162124121586,5.20442803180935,15.5232458088582));
#6508=CARTESIAN_POINT('Ctrl Pts',(3.06596975064604,5.29154055140843,15.5309708962655));
#6509=CARTESIAN_POINT('Ctrl Pts',(2.91696816073999,5.37244100123297,15.5386959836729));
#6510=CARTESIAN_POINT('Ctrl Pts',(2.76854434899991,5.45302774626044,15.5463911157836));
#6511=CARTESIAN_POINT('Ctrl Pts',(2.61679666260055,5.52745039188512,15.5540862478942));
#6512=CARTESIAN_POINT('Ctrl Pts',(2.46225721888687,5.59545484751146,15.5617813800049));
#6513=CARTESIAN_POINT('Ctrl Pts',(2.30712272332804,5.66372115328962,15.5695061421081));
#6514=CARTESIAN_POINT('Ctrl Pts',(2.14911997242034,5.7255438950742,15.5772309042113));
#6515=CARTESIAN_POINT('Ctrl Pts',(1.98880215989118,5.78069991707857,15.5849556663144));
#6516=CARTESIAN_POINT('Ctrl Pts',(1.82851562036121,5.83584517986533,15.5926789215578));
#6517=CARTESIAN_POINT('Ctrl Pts',(1.66591521981019,5.88432621473104,15.6004021768011));
#6518=CARTESIAN_POINT('Ctrl Pts',(1.50157156108632,5.92596898485276,15.6081254320444));
#6519=CARTESIAN_POINT('Ctrl Pts',(1.33722155126887,5.96761336426765,15.6158489857544));
#6520=CARTESIAN_POINT('Ctrl Pts',(1.17112845470606,6.00241886844284,15.6235725394645));
#6521=CARTESIAN_POINT('Ctrl Pts',(1.00387614733472,6.03026187186862,15.6312960931745));
#6522=CARTESIAN_POINT('Ctrl Pts',(0.836635073387881,6.05810300523184,15.6390191281356));
#6523=CARTESIAN_POINT('Ctrl Pts',(0.668235257094541,6.0789825216141,15.6467421630968));
#6524=CARTESIAN_POINT('Ctrl Pts',(0.499269016725837,6.09282824404542,15.6544651980579));
#6525=CARTESIAN_POINT('Ctrl Pts',(0.330257872491124,6.1066776460666,15.6621902854652));
#6526=CARTESIAN_POINT('Ctrl Pts',(0.16068031929641,6.11348949079551,15.6699153728726));
#6527=CARTESIAN_POINT('Ctrl Pts',(-0.00886700772179213,6.11324356938884,
15.67764046028));
#6528=CARTESIAN_POINT('Ctrl Pts',(-0.177756887100845,6.11299860158287,15.6853355923907));
#6529=CARTESIAN_POINT('Ctrl Pts',(-0.346616462158736,6.10575053832936,15.6930307245014));
#6530=CARTESIAN_POINT('Ctrl Pts',(-0.514856902391781,6.09153083654343,15.7007258566121));
#6531=CARTESIAN_POINT('Ctrl Pts',(-0.683745149953988,6.07725638200589,15.7084506187153));
#6532=CARTESIAN_POINT('Ctrl Pts',(-0.852069297951079,6.0559514084714,15.7161753808185));
#6533=CARTESIAN_POINT('Ctrl Pts',(-1.01923680827505,6.0276846210761,15.7239001429217));
#6534=CARTESIAN_POINT('Ctrl Pts',(-1.18637170943766,5.99942334764837,15.731623398165));
#6535=CARTESIAN_POINT('Ctrl Pts',(-1.35235011082691,5.96420302292877,15.7393466534083));
#6536=CARTESIAN_POINT('Ctrl Pts',(-1.51658768688012,5.92214381373026,15.7470699086516));
#6537=CARTESIAN_POINT('Ctrl Pts',(-1.68083160992742,5.88008297914517,15.7547934623617));
#6538=CARTESIAN_POINT('Ctrl Pts',(-1.84333426502474,5.83118280600485,15.7625170160718));
#6539=CARTESIAN_POINT('Ctrl Pts',(-2.00352378941037,5.77561407884622,15.7702405697819));
#6540=CARTESIAN_POINT('Ctrl Pts',(-2.16370255474059,5.72004908393549,15.777963604743));
#6541=CARTESIAN_POINT('Ctrl Pts',(-2.32156820081101,5.65781653519248,15.7856866397042));
#6542=CARTESIAN_POINT('Ctrl Pts',(-2.47656606591191,5.58913643451952,15.7934096746653));
#6543=CARTESIAN_POINT('Ctrl Pts',(-2.63160512269235,5.52043808166809,15.8011347620727));
#6544=CARTESIAN_POINT('Ctrl Pts',(-2.78377458473753,5.44528887943016,15.80885984948));
#6545=CARTESIAN_POINT('Ctrl Pts',(-2.93254086265715,5.36395652959138,15.8165849368874));
#6546=CARTESIAN_POINT('Ctrl Pts',(-3.08073027487097,5.28293955931342,15.824280068998));
#6547=CARTESIAN_POINT('Ctrl Pts',(-3.22554259039452,5.19578748657979,15.8319752011087));
#6548=CARTESIAN_POINT('Ctrl Pts',(-3.36647579169918,5.10280964826274,15.8396703332193));
#6549=CARTESIAN_POINT('Ctrl Pts',(-3.50795165421478,5.00947380015195,15.8473950953225));
#6550=CARTESIAN_POINT('Ctrl Pts',(-3.64556856027343,4.91023415150679,15.8551198574257));
#6551=CARTESIAN_POINT('Ctrl Pts',(-3.77883905724067,4.80543452166112,15.8628446195289));
#6552=CARTESIAN_POINT('Ctrl Pts',(-3.91208355729635,4.70065533495006,15.8705678747723));
#6553=CARTESIAN_POINT('Ctrl Pts',(-4.04098309104772,4.59031852694703,15.8782911300157));
#6554=CARTESIAN_POINT('Ctrl Pts',(-4.16508203828198,4.47480917770589,15.8860143852591));
#6555=CARTESIAN_POINT('Ctrl Pts',(-4.28918578134367,4.35929536458396,15.8937379389692));
#6556=CARTESIAN_POINT('Ctrl Pts',(-4.40848833197411,4.2386088232472,15.9014614926792));
#6557=CARTESIAN_POINT('Ctrl Pts',(-4.52256923087092,4.11317311992573,15.9091850463893));
#6558=CARTESIAN_POINT('Ctrl Pts',(-4.63664246757641,3.98774584143584,15.9169080813504));
#6559=CARTESIAN_POINT('Ctrl Pts',(-4.74549454112277,3.85757027377182,15.9246311163115));
#6560=CARTESIAN_POINT('Ctrl Pts',(-4.84874364392741,3.72310497273089,15.9323541512726));
#6561=CARTESIAN_POINT('Ctrl Pts',(-4.95202018584586,3.58860393667051,15.94007923868));
#6562=CARTESIAN_POINT('Ctrl Pts',(-5.04969058670783,3.44981113940905,15.9478043260874));
#6563=CARTESIAN_POINT('Ctrl Pts',(-5.14141436410374,3.30721694164259,15.9555294134948));
#6564=CARTESIAN_POINT('Ctrl Pts',(-5.23278246746901,3.16517567632729,15.9632245456053));
#6565=CARTESIAN_POINT('Ctrl Pts',(-5.31824984162882,3.01936271921126,15.9709196777159));
#6566=CARTESIAN_POINT('Ctrl Pts',(-5.39752364769265,2.87028988694499,15.9786148098265));
#6567=CARTESIAN_POINT('Ctrl Pts',(-5.4770292568796,2.72078115346736,15.9863324431357));
#6568=CARTESIAN_POINT('Ctrl Pts',(-5.55033365351206,2.56793952772914,15.9940500764449));
#6569=CARTESIAN_POINT('Ctrl Pts',(-5.6171735517017,2.41229908024748,16.0017677097541));
#6570=CARTESIAN_POINT('Ctrl Pts',(-5.68400019521871,2.25668949701362,16.0094838126196));
#6571=CARTESIAN_POINT('Ctrl Pts',(-5.74436477270071,2.09828249158631,16.0171999154851));
#6572=CARTESIAN_POINT('Ctrl Pts',(-5.79805168318064,1.93763315456412,16.0249160183505));
#6573=CARTESIAN_POINT('Ctrl Pts',(-5.85174033065206,1.77697861987778,16.0326323708635));
#6574=CARTESIAN_POINT('Ctrl Pts',(-5.8987507742332,1.61408190886903,16.0403487233766));
#6575=CARTESIAN_POINT('Ctrl Pts',(-5.93891670190994,1.44951508107891,16.0480650758896));
#6576=CARTESIAN_POINT('Ctrl Pts',(-5.97908014906332,1.28495841642665,16.0557809518645));
#6577=CARTESIAN_POINT('Ctrl Pts',(-6.01239985098338,1.11873215051005,16.0634968278395));
#6578=CARTESIAN_POINT('Ctrl Pts',(-6.03876017516021,0.95142057440389,16.0712127038145));
#6579=CARTESIAN_POINT('Ctrl Pts',(-6.0651272466124,0.784066172675864,16.0789305547705));
#6580=CARTESIAN_POINT('Ctrl Pts',(-6.08453132973179,0.615626219838155,16.0866484057265));
#6581=CARTESIAN_POINT('Ctrl Pts',(-6.09690830023527,0.446693117276577,16.0943662566825));
#6582=CARTESIAN_POINT('Ctrl Pts',(-6.10779984683707,0.298034545405651,16.1011578486418));
#6583=CARTESIAN_POINT('Ctrl Pts',(-6.11325053225869,0.148994340849137,16.1079494406012));
#6584=CARTESIAN_POINT('Ctrl Pts',(-6.113249999961,-2.1837017445121E-5,16.1147410325606));
#6585=CARTESIAN_POINT('Origin',(0.,0.,-3.86474103256053));
#6586=CARTESIAN_POINT('',(3.72288481551393,-4.8488307603735,13.2346211120867));
#6587=CARTESIAN_POINT('',(3.72270802987534,-4.84860079634452,13.3801373157199));
#6588=CARTESIAN_POINT('',(3.72292453512038,-4.84888218750453,-3.86474103256053));
#6589=CARTESIAN_POINT('',(-6.11319871911702,9.79097444517703E-6,14.5102589673365));
#6590=CARTESIAN_POINT('Ctrl Pts',(3.72270802987534,-4.84860079634452,13.3801373157199));
#6591=CARTESIAN_POINT('Ctrl Pts',(4.24171171221953,-4.44951091176983,13.4099614103007));
#6592=CARTESIAN_POINT('Ctrl Pts',(5.40481509300789,-3.21922256216121,13.4861003304172));
#6593=CARTESIAN_POINT('Ctrl Pts',(6.34339259002546,-0.610081612305798,13.6085540760694));
#6594=CARTESIAN_POINT('Ctrl Pts',(5.86217951430019,2.49913594407806,13.7474985526766));
#6595=CARTESIAN_POINT('Ctrl Pts',(3.9520731391245,4.99919463792661,13.8864430292838));
#6596=CARTESIAN_POINT('Ctrl Pts',(1.07865767154433,6.28071068848758,14.025387505891));
#6597=CARTESIAN_POINT('Ctrl Pts',(-2.05767821932051,6.03131739096838,14.1643319824981));
#6598=CARTESIAN_POINT('Ctrl Pts',(-4.69245959230686,4.31180381040591,14.3032764591053));
#6599=CARTESIAN_POINT('Ctrl Pts',(-5.92983339331411,2.01258115915036,14.4185854537362));
#6600=CARTESIAN_POINT('Ctrl Pts',(-6.11275550933371,0.497909914167423,14.4875796228312));
#6601=CARTESIAN_POINT('Ctrl Pts',(-6.11272776669357,9.81098628248876E-6,
14.5102589663906));
#6602=CARTESIAN_POINT('Ctrl Pts',(-6.11324999999216,9.78879540440889E-6,
14.5102589674395));
#6603=CARTESIAN_POINT('Ctrl Pts',(-6.11325027459207,-0.171481984661658,
14.5180697483018));
#6604=CARTESIAN_POINT('Ctrl Pts',(-6.10603005521547,-0.342959526338876,
14.5258805291642));
#6605=CARTESIAN_POINT('Ctrl Pts',(-6.0916189476117,-0.513813350934067,14.5336913100265));
#6606=CARTESIAN_POINT('Ctrl Pts',(-6.0770204414231,-0.686888917662023,14.5416036604087));
#6607=CARTESIAN_POINT('Ctrl Pts',(-6.05504273155774,-0.859324115509616,
14.5495160107909));
#6608=CARTESIAN_POINT('Ctrl Pts',(-6.02577085604886,-1.0304907340157,14.5574283611731));
#6609=CARTESIAN_POINT('Ctrl Pts',(-5.99649898053998,-1.20165735252176,14.5653407115553));
#6610=CARTESIAN_POINT('Ctrl Pts',(-5.95993300206572,-1.37155507669805,14.5732530619375));
#6611=CARTESIAN_POINT('Ctrl Pts',(-5.91621184517902,-1.53956583667718,14.5811654123197));
#6612=CARTESIAN_POINT('Ctrl Pts',(-5.873527242057,-1.70359334922727,14.5888901744229));
#6613=CARTESIAN_POINT('Ctrl Pts',(-5.82400936005968,-1.86587366244741,14.5966149365261));
#6614=CARTESIAN_POINT('Ctrl Pts',(-5.76782631097592,-2.02583444755831,14.6043396986293));
#6615=CARTESIAN_POINT('Ctrl Pts',(-5.71165422145075,-2.18576402931476,14.6120629538727));
#6616=CARTESIAN_POINT('Ctrl Pts',(-5.64881966409654,-2.3433746869595,14.619786209116));
#6617=CARTESIAN_POINT('Ctrl Pts',(-5.57954007672257,-2.49811090521352,14.6275094643593));
#6618=CARTESIAN_POINT('Ctrl Pts',(-5.51025781202523,-2.65285310327934,14.6352330180694));
#6619=CARTESIAN_POINT('Ctrl Pts',(-5.43453014479446,-2.80472034880149,14.6429565717794));
#6620=CARTESIAN_POINT('Ctrl Pts',(-5.35262228694381,-2.95317798579977,14.6506801254895));
#6621=CARTESIAN_POINT('Ctrl Pts',(-5.27071993039675,-3.10162565170919,14.6584031604506));
#6622=CARTESIAN_POINT('Ctrl Pts',(-5.18263836701313,-3.24666388985333,14.6661261954117));
#6623=CARTESIAN_POINT('Ctrl Pts',(-5.0886883998481,-3.38778333601064,14.6738492303728));
#6624=CARTESIAN_POINT('Ctrl Pts',(-4.99471346487469,-3.52894028556893,14.6815743177802));
#6625=CARTESIAN_POINT('Ctrl Pts',(-4.89486718366908,-3.66617609687749,14.6892994051876));
#6626=CARTESIAN_POINT('Ctrl Pts',(-4.78950379893765,-3.79901025564051,14.6970244925949));
#6627=CARTESIAN_POINT('Ctrl Pts',(-4.68454897805601,-3.93132932811027,14.7047196247056));
#6628=CARTESIAN_POINT('Ctrl Pts',(-4.57411998380422,-4.05928059906078,14.7124147568162));
#6629=CARTESIAN_POINT('Ctrl Pts',(-4.45860674238751,-4.18242172422111,14.7201098889269));
#6630=CARTESIAN_POINT('Ctrl Pts',(-4.3426487189408,-4.30603700246513,14.7278346510301));
#6631=CARTESIAN_POINT('Ctrl Pts',(-4.22152612618802,-4.42484877890641,14.7355594131333));
#6632=CARTESIAN_POINT('Ctrl Pts',(-4.09566040630592,-4.53843490629953,14.7432841752365));
#6633=CARTESIAN_POINT('Ctrl Pts',(-3.96981923889555,-4.65199887658597,14.7510074304798));
#6634=CARTESIAN_POINT('Ctrl Pts',(-3.83923702567417,-4.76033901961392,14.7587306857232));
#6635=CARTESIAN_POINT('Ctrl Pts',(-3.70437047921442,-4.86307155152222,14.7664539409665));
#6636=CARTESIAN_POINT('Ctrl Pts',(-3.56949872081038,-4.96580805354948,14.7741774946765));
#6637=CARTESIAN_POINT('Ctrl Pts',(-3.43034254756137,-5.06293631562267,14.7819010483866));
#6638=CARTESIAN_POINT('Ctrl Pts',(-3.2873906440296,-5.15411372750414,14.7896246020966));
#6639=CARTESIAN_POINT('Ctrl Pts',(-3.1444483417965,-5.24528501549679,14.7973476370577));
#6640=CARTESIAN_POINT('Ctrl Pts',(-2.99771108668624,-5.33050608269726,14.8050706720189));
#6641=CARTESIAN_POINT('Ctrl Pts',(-2.84769549771557,-5.4094783403569,14.81279370698));
#6642=CARTESIAN_POINT('Ctrl Pts',(-2.69764004113689,-5.48847158540215,14.8205187943874));
#6643=CARTESIAN_POINT('Ctrl Pts',(-2.54430478937575,-5.56121255283737,14.8282438817947));
#6644=CARTESIAN_POINT('Ctrl Pts',(-2.38823070429244,-5.62744877058644,14.8359689692021));
#6645=CARTESIAN_POINT('Ctrl Pts',(-2.23276182213772,-5.69342814650979,14.8436641013128));
#6646=CARTESIAN_POINT('Ctrl Pts',(-2.0745756094302,-5.75295303725884,14.8513592334234));
#6647=CARTESIAN_POINT('Ctrl Pts',(-1.91422610098583,-5.8058215608822,14.8590543655341));
#6648=CARTESIAN_POINT('Ctrl Pts',(-1.75325916912747,-5.85889365397492,14.8667791276373));
#6649=CARTESIAN_POINT('Ctrl Pts',(-1.59005522988538,-5.90527678573933,14.8745038897405));
#6650=CARTESIAN_POINT('Ctrl Pts',(-1.42518633022512,-5.94480188792187,14.8822286518438));
#6651=CARTESIAN_POINT('Ctrl Pts',(-1.26034959133956,-5.98431927999105,14.8899519070871));
#6652=CARTESIAN_POINT('Ctrl Pts',(-1.09384884809832,-6.01698123800301,14.8976751623304));
#6653=CARTESIAN_POINT('Ctrl Pts',(-0.926268765157316,-6.04266925598232,
14.9053984175737));
#6654=CARTESIAN_POINT('Ctrl Pts',(-0.758682206050966,-6.06835826668016,
14.9131219712838));
#6655=CARTESIAN_POINT('Ctrl Pts',(-0.590016536436749,-6.08707274610645,
14.9208455249938));
#6656=CARTESIAN_POINT('Ctrl Pts',(-0.420864797743603,-6.09874564025425,
14.9285690787038));
#6657=CARTESIAN_POINT('Ctrl Pts',(-0.251724420048848,-6.11041775039751,
14.936292113665));
#6658=CARTESIAN_POINT('Ctrl Pts',(-0.0820983548121702,-6.11504919988803,
14.9440151486261));
#6659=CARTESIAN_POINT('Ctrl Pts',(0.0874168877315281,-6.11262495579758,
14.9517381835872));
#6660=CARTESIAN_POINT('Ctrl Pts',(0.256977180041634,-6.11020006744866,14.9594632709946));
#6661=CARTESIAN_POINT('Ctrl Pts',(0.426426273658079,-6.10071574097748,14.9671883584019));
#6662=CARTESIAN_POINT('Ctrl Pts',(0.595168345824421,-6.0842090860381,14.9749134458093));
#6663=CARTESIAN_POINT('Ctrl Pts',(0.763256092859132,-6.0677664383675,14.9826085779199));
#6664=CARTESIAN_POINT('Ctrl Pts',(0.930641984313115,-6.04435588836248,14.9903037100306));
#6665=CARTESIAN_POINT('Ctrl Pts',(1.09674292152156,-6.01406522467061,14.9979988421413));
#6666=CARTESIAN_POINT('Ctrl Pts',(1.26348285838097,-5.98365803109124,15.0057235778581));
#6667=CARTESIAN_POINT('Ctrl Pts',(1.4289869835453,-5.94630688366497,15.013448313575));
#6668=CARTESIAN_POINT('Ctrl Pts',(1.59267208640143,-5.90213700177298,15.0211730492918));
#6669=CARTESIAN_POINT('Ctrl Pts',(1.75632506302105,-5.8579757890393,15.0288962688861));
#6670=CARTESIAN_POINT('Ctrl Pts',(1.91815942393135,-5.80699859479505,15.0366194884803));
#6671=CARTESIAN_POINT('Ctrl Pts',(2.07760507091788,-5.74938107380232,15.0443427080746));
#6672=CARTESIAN_POINT('Ctrl Pts',(2.23705274244332,-5.69176282121914,15.0520660257333));
#6673=CARTESIAN_POINT('Ctrl Pts',(2.39411133999764,-5.62750417717528,15.0597893433921));
#6674=CARTESIAN_POINT('Ctrl Pts',(2.54822806804752,-5.55682996642104,15.0675126610508));
#6675=CARTESIAN_POINT('Ctrl Pts',(2.70233483408483,-5.48616032400525,15.075235479479));
#6676=CARTESIAN_POINT('Ctrl Pts',(2.85349982309663,-5.40907607686579,15.0829582979071));
#6677=CARTESIAN_POINT('Ctrl Pts',(3.0011920750816,-5.3258493868084,15.0906811163352));
#6678=CARTESIAN_POINT('Ctrl Pts',(3.14891480881972,-5.24260551984844,15.0984055286523));
#6679=CARTESIAN_POINT('Ctrl Pts',(3.29316309677674,-5.15321683176344,15.1061299409694));
#6680=CARTESIAN_POINT('Ctrl Pts',(3.433431615175,-5.05800088042863,15.1138543532864));
#6681=CARTESIAN_POINT('Ctrl Pts',(3.53194728744746,-4.9911272614304,15.1192794884559));
#6682=CARTESIAN_POINT('Ctrl Pts',(3.62850037180794,-4.92138014078745,15.1247046236253));
#6683=CARTESIAN_POINT('Ctrl Pts',(3.7229245351204,-4.84888218750451,15.1301297587947));
#6684=CARTESIAN_POINT('',(-6.11324999916302,0.000101159726426482,14.3647410325606));
#6685=CARTESIAN_POINT('Ctrl Pts',(-6.11324999916302,0.000101159726426482,
14.3647410325606));
#6686=CARTESIAN_POINT('Ctrl Pts',(-6.11325281292563,-0.169939180116824,
14.3724862375428));
#6687=CARTESIAN_POINT('Ctrl Pts',(-6.10615676234947,-0.339980975408143,
14.3802314425249));
#6688=CARTESIAN_POINT('Ctrl Pts',(-6.09198753638617,-0.509424596005636,
14.3879766475071));
#6689=CARTESIAN_POINT('Ctrl Pts',(-6.07781849764592,-0.67886597768408,14.3957217501491));
#6690=CARTESIAN_POINT('Ctrl Pts',(-6.05657649931014,-0.847708888657797,
14.4034668527911));
#6691=CARTESIAN_POINT('Ctrl Pts',(-6.02833915632798,-1.01535834993506,14.4112119554332));
#6692=CARTESIAN_POINT('Ctrl Pts',(-6.00009448276363,-1.18305133400965,14.4189590687499));
#6693=CARTESIAN_POINT('Ctrl Pts',(-5.96485088767088,-1.34954994037174,14.4267061820666));
#6694=CARTESIAN_POINT('Ctrl Pts',(-5.92273736991832,-1.51426801111066,14.4344532953833));
#6695=CARTESIAN_POINT('Ctrl Pts',(-5.89415787113032,-1.6260506442002,14.4397107193047));
#6696=CARTESIAN_POINT('Ctrl Pts',(-5.8624155724781,-1.73701346732266,14.4449681432261));
#6697=CARTESIAN_POINT('Ctrl Pts',(-5.82756400566072,-1.84697680614231,14.4502255671475));
#6698=CARTESIAN_POINT('Ctrl Pts',(-5.77635640539604,-2.00854654926322,14.4579503292507));
#6699=CARTESIAN_POINT('Ctrl Pts',(-5.71841629279437,-2.16801398809637,14.4656750913539));
#6700=CARTESIAN_POINT('Ctrl Pts',(-5.65394149203249,-2.32481637278591,14.4733998534571));
#6701=CARTESIAN_POINT('Ctrl Pts',(-5.58947926829106,-2.48158817022624,14.4811231087004));
#6702=CARTESIAN_POINT('Ctrl Pts',(-5.51848502035082,-2.6356956579108,14.4888463639437));
#6703=CARTESIAN_POINT('Ctrl Pts',(-5.44120495122343,-2.78659545705537,14.496569619187));
#6704=CARTESIAN_POINT('Ctrl Pts',(-5.36392189559249,-2.93750108775251,14.504293172897));
#6705=CARTESIAN_POINT('Ctrl Pts',(-5.2803526736176,-3.08519849797062,14.5120167266071));
#6706=CARTESIAN_POINT('Ctrl Pts',(-5.19079010568986,-3.22916763906309,14.5197402803171));
#6707=CARTESIAN_POINT('Ctrl Pts',(-5.10123355319063,-3.37312711053468,14.5274633152782));
#6708=CARTESIAN_POINT('Ctrl Pts',(-5.00568462771779,-3.51335854486044,14.5351863502394));
#6709=CARTESIAN_POINT('Ctrl Pts',(-4.90448035517501,-3.64936953571468,14.5429093852005));
#6710=CARTESIAN_POINT('Ctrl Pts',(-4.80324918694549,-3.78541667236505,14.5506344726078));
#6711=CARTESIAN_POINT('Ctrl Pts',(-4.69635985597466,-3.91724086855353,14.5583595600152));
#6712=CARTESIAN_POINT('Ctrl Pts',(-4.58419125898163,-4.04438080100977,14.5660846474226));
#6713=CARTESIAN_POINT('Ctrl Pts',(-4.47245761416772,-4.17102772747184,14.5737797795333));
#6714=CARTESIAN_POINT('Ctrl Pts',(-4.35548580370585,-4.29302644085327,14.5814749116439));
#6715=CARTESIAN_POINT('Ctrl Pts',(-4.23368836199903,-4.40995560249465,14.5891700437546));
#6716=CARTESIAN_POINT('Ctrl Pts',(-4.11142194104218,-4.52733499814559,14.5968948058578));
#6717=CARTESIAN_POINT('Ctrl Pts',(-3.98424932910431,-4.63964727471922,14.604619567961));
#6718=CARTESIAN_POINT('Ctrl Pts',(-3.8526134767485,-4.74649291174819,14.6123443300642));
#6719=CARTESIAN_POINT('Ctrl Pts',(-3.72100330243681,-4.85331770652992,14.6200675853075));
#6720=CARTESIAN_POINT('Ctrl Pts',(-3.5849318708643,-4.95467778995039,14.6277908405509));
#6721=CARTESIAN_POINT('Ctrl Pts',(-3.44487534762473,-5.05021379763544,14.6355140957942));
#6722=CARTESIAN_POINT('Ctrl Pts',(-3.30481341187349,-5.14575349732815,14.6432376495042));
#6723=CARTESIAN_POINT('Ctrl Pts',(-3.16076633585919,-5.23546848904279,14.6509612032143));
#6724=CARTESIAN_POINT('Ctrl Pts',(-3.01324005929328,-5.31904219832577,14.6586847569243));
#6725=CARTESIAN_POINT('Ctrl Pts',(-2.86572369126158,-5.40261029441918,14.6664077918855));
#6726=CARTESIAN_POINT('Ctrl Pts',(-2.71472886609083,-5.48003777729016,14.6741308268466));
#6727=CARTESIAN_POINT('Ctrl Pts',(-2.56078711661227,-5.55105349513879,14.6818538618077));
#6728=CARTESIAN_POINT('Ctrl Pts',(-2.40680445612331,-5.62208808587137,14.6895789492151));
#6729=CARTESIAN_POINT('Ctrl Pts',(-2.24987359344524,-5.68670737180964,14.6973040366224));
#6730=CARTESIAN_POINT('Ctrl Pts',(-2.09054795822268,-5.74468752821866,14.7050291240298));
#6731=CARTESIAN_POINT('Ctrl Pts',(-1.93184013434901,-5.80244285703738,14.7127242561405));
#6732=CARTESIAN_POINT('Ctrl Pts',(-1.77075638155635,-5.85361037696616,14.7204193882511));
#6733=CARTESIAN_POINT('Ctrl Pts',(-1.60786053781036,-5.89801746805248,14.7281145203618));
#6734=CARTESIAN_POINT('Ctrl Pts',(-1.44433746602451,-5.94259554798699,14.735839282465));
#6735=CARTESIAN_POINT('Ctrl Pts',(-1.27893039782108,-5.9803767931299,14.7435640445682));
#6736=CARTESIAN_POINT('Ctrl Pts',(-1.11221944192877,-6.01122229463323,14.7512888066714));
#6737=CARTESIAN_POINT('Ctrl Pts',(-0.945541006138027,-6.04206177914244,
14.7590120619147));
#6738=CARTESIAN_POINT('Ctrl Pts',(-0.777559501621107,-6.06596816200061,
14.766735317158));
#6739=CARTESIAN_POINT('Ctrl Pts',(-0.608864992242848,-6.08285368751552,
14.7744585724014));
#6740=CARTESIAN_POINT('Ctrl Pts',(-0.440163963631982,-6.09973986557489,
14.7821821261114));
#6741=CARTESIAN_POINT('Ctrl Pts',(-0.270750189969728,-6.10960460785247,
14.7899056798215));
#6742=CARTESIAN_POINT('Ctrl Pts',(-0.101219408601492,-6.11241197841101,
14.7976292335315));
#6743=CARTESIAN_POINT('Ctrl Pts',(0.0682999863096924,-6.11521916041379,
14.8053522684926));
#6744=CARTESIAN_POINT('Ctrl Pts',(0.237936056286156,-6.11096991401799,14.8130753034537));
#6745=CARTESIAN_POINT('Ctrl Pts',(0.407092321521854,-6.0996804346013,14.8207983384149));
#6746=CARTESIAN_POINT('Ctrl Pts',(0.576293541123662,-6.08838795493281,14.8285234258222));
#6747=CARTESIAN_POINT('Ctrl Pts',(0.74501438459519,-6.07005152250148,14.8362485132296));
#6748=CARTESIAN_POINT('Ctrl Pts',(0.912661786618967,-6.04473936789217,14.8439736006369));
#6749=CARTESIAN_POINT('Ctrl Pts',(1.07965910827491,-6.01952536532448,14.8516687327476));
#6750=CARTESIAN_POINT('Ctrl Pts',(1.24559099469841,-5.98738972191345,14.8593638648583));
#6751=CARTESIAN_POINT('Ctrl Pts',(1.40987973861898,-5.94845061214529,14.867058996969));
#6752=CARTESIAN_POINT('Ctrl Pts',(1.57479970578628,-5.90936189218044,14.87478369499));
#6753=CARTESIAN_POINT('Ctrl Pts',(1.73812228136712,-5.86340344921617,14.8825083930111));
#6754=CARTESIAN_POINT('Ctrl Pts',(1.89927161296279,-5.8107308406683,14.8902330910321));
#6755=CARTESIAN_POINT('Ctrl Pts',(2.06334154419179,-5.75710361692166,14.8980977880838));
#6756=CARTESIAN_POINT('Ctrl Pts',(2.2251583716967,-5.69651659285686,14.9059624851354));
#6757=CARTESIAN_POINT('Ctrl Pts',(2.38413079366924,-5.62918696804237,14.9138271821871));
#6758=CARTESIAN_POINT('Ctrl Pts',(2.54023647548796,-5.56307149431523,14.9215500556284));
#6759=CARTESIAN_POINT('Ctrl Pts',(2.69359917291047,-5.49045467698622,14.9292729290696));
#6760=CARTESIAN_POINT('Ctrl Pts',(2.84367910684593,-5.41159077349608,14.9369958025109));
#6761=CARTESIAN_POINT('Ctrl Pts',(2.99789316486852,-5.33055447324061,14.9449314113678));
#6762=CARTESIAN_POINT('Ctrl Pts',(3.14864068572877,-5.24292211613975,14.9528670202246));
#6763=CARTESIAN_POINT('Ctrl Pts',(3.29536275830877,-5.14902028095167,14.9608026290815));
#6764=CARTESIAN_POINT('Ctrl Pts',(3.44208483088875,-5.0551184457636,14.9687382379383));
#6765=CARTESIAN_POINT('Ctrl Pts',(3.58478115207154,-4.95494733205319,14.9766738467952));
#6766=CARTESIAN_POINT('Ctrl Pts',(3.72292453512039,-4.84888218750452,14.984609455652));
#6767=CARTESIAN_POINT('Ctrl Pts',(3.72288481551393,-4.8488307603735,13.2346211120867));
#6768=CARTESIAN_POINT('Ctrl Pts',(4.32622015324387,-4.38460469236938,13.2693039928211));
#6769=CARTESIAN_POINT('Ctrl Pts',(5.53405973259451,-3.03738285194378,13.3503016990913));
#6770=CARTESIAN_POINT('Ctrl Pts',(6.36662318807926,-0.277377862609176,13.4776142308971));
#6771=CARTESIAN_POINT('Ctrl Pts',(5.72340370477089,2.80240598947921,13.6165587075043));
#6772=CARTESIAN_POINT('Ctrl Pts',(3.68511721884909,5.19910957578276,13.7555031841115));
#6773=CARTESIAN_POINT('Ctrl Pts',(0.748591556037913,6.32854169456779,13.8944476607187));
#6774=CARTESIAN_POINT('Ctrl Pts',(-2.3704016439475,5.9154057632613,14.0333921373259));
#6775=CARTESIAN_POINT('Ctrl Pts',(-4.91161468251336,4.06040275196602,14.1723366139331));
#6776=CARTESIAN_POINT('Ctrl Pts',(-5.98000021356576,1.79908250121632,14.2827862424113));
#6777=CARTESIAN_POINT('Ctrl Pts',(-6.11306665977086,0.391299537207678,14.3469210453537));
#6778=CARTESIAN_POINT('Ctrl Pts',(-6.11283634071177,0.000101368021089277,
14.3647410227605));
#6779=CARTESIAN_POINT('Origin',(0.,0.,-3.86474103256053));
#6780=CARTESIAN_POINT('',(3.72292453512038,-4.84888218750453,11.484610425966));
#6781=CARTESIAN_POINT('',(3.72292453512038,-4.84888218750453,11.6301271545495));
#6782=CARTESIAN_POINT('',(3.72292453512038,-4.84888218750453,-3.86474103256053));
#6783=CARTESIAN_POINT('',(-6.11324999912966,-0.000103156033837302,12.7602589674395));
#6784=CARTESIAN_POINT('Ctrl Pts',(3.72292453512038,-4.84888218750453,11.6301271545495));
#6785=CARTESIAN_POINT('Ctrl Pts',(3.8574118287249,-4.74562415283574,11.6378518926703));
#6786=CARTESIAN_POINT('Ctrl Pts',(3.98758795371617,-4.63677720859856,11.6455766307911));
#6787=CARTESIAN_POINT('Ctrl Pts',(4.11299847765816,-4.52272805785199,11.6533013689119));
#6788=CARTESIAN_POINT('Ctrl Pts',(4.16727742242853,-4.47336643045504,11.6566447137975));
#6789=CARTESIAN_POINT('Ctrl Pts',(4.22066408427948,-4.42303080373098,11.6599880586832));
#6790=CARTESIAN_POINT('Ctrl Pts',(4.27312366791289,-4.37175475995883,11.6633314035688));
#6791=CARTESIAN_POINT('Ctrl Pts',(4.39433096702921,-4.2532820168577,11.671056165672));
#6792=CARTESIAN_POINT('Ctrl Pts',(4.51062969223976,-4.1297444630101,11.6787809277752));
#6793=CARTESIAN_POINT('Ctrl Pts',(4.62160644222549,-4.00157212301363,11.6865056898784));
#6794=CARTESIAN_POINT('Ctrl Pts',(4.73256154411224,-3.87342478543887,11.6942289451217));
#6795=CARTESIAN_POINT('Ctrl Pts',(4.83819653493191,-3.74064470517301,11.701952200365));
#6796=CARTESIAN_POINT('Ctrl Pts',(4.93813709314584,-3.60369638174432,11.7096754556083));
#6797=CARTESIAN_POINT('Ctrl Pts',(5.03808151358274,-3.46674276592013,11.7173990093183));
#6798=CARTESIAN_POINT('Ctrl Pts',(5.13233087103584,-3.32562083826061,11.7251225630284));
#6799=CARTESIAN_POINT('Ctrl Pts',(5.22055266564044,-3.18082621778909,11.7328461167384));
#6800=CARTESIAN_POINT('Ctrl Pts',(5.30876853486909,-3.03604132238117,11.7405691516996));
#6801=CARTESIAN_POINT('Ctrl Pts',(5.39095748648467,-2.8875844984743,11.7482921866607));
#6802=CARTESIAN_POINT('Ctrl Pts',(5.46683160662606,-2.73597838940558,11.7560152216218));
#6803=CARTESIAN_POINT('Ctrl Pts',(5.54272589080293,-2.58433199003818,11.7637403090292));
#6804=CARTESIAN_POINT('Ctrl Pts',(5.61230184615108,-2.42953491573295,11.7714653964366));
#6805=CARTESIAN_POINT('Ctrl Pts',(5.67531816577891,-2.27213320025035,11.7791904838439));
#6806=CARTESIAN_POINT('Ctrl Pts',(5.73809012926561,-2.11534183580111,11.7868856159546));
#6807=CARTESIAN_POINT('Ctrl Pts',(5.79435315262763,-1.95596629592201,11.7945807480653));
#6808=CARTESIAN_POINT('Ctrl Pts',(5.84391677695614,-1.79456464539747,11.802275880176));
#6809=CARTESIAN_POINT('Ctrl Pts',(5.89367124528793,-1.63254152020196,11.8100006422792));
#6810=CARTESIAN_POINT('Ctrl Pts',(5.93669221314727,-1.46841925778513,11.8177254043824));
#6811=CARTESIAN_POINT('Ctrl Pts',(5.972822398388,-1.30277325725339,11.8254501664856));
#6812=CARTESIAN_POINT('Ctrl Pts',(6.00894553575759,-1.13715956908482,11.8331734217289));
#6813=CARTESIAN_POINT('Ctrl Pts',(6.03818050512413,-0.970023045347367,11.8408966769722));
#6814=CARTESIAN_POINT('Ctrl Pts',(6.06042083513189,-0.801950661574166,11.8486199322155));
#6815=CARTESIAN_POINT('Ctrl Pts',(6.08266202462166,-0.633871782610093,11.8563434859256));
#6816=CARTESIAN_POINT('Ctrl Pts',(6.09790798834629,-0.464857284898449,11.8640670396356));
#6817=CARTESIAN_POINT('Ctrl Pts',(6.10610386813031,-0.295501462101399,11.8717905933457));
#6818=CARTESIAN_POINT('Ctrl Pts',(6.11429919744185,-0.126157014009869,11.8795136283068));
#6819=CARTESIAN_POINT('Ctrl Pts',(6.11544537508058,0.0435283967033413,11.8872366632679));
#6820=CARTESIAN_POINT('Ctrl Pts',(6.10953962422672,0.212958076868715,11.894959698229));
#6821=CARTESIAN_POINT('Ctrl Pts',(6.10363230388156,0.382432784061904,11.9026847856364));
#6822=CARTESIAN_POINT('Ctrl Pts',(6.09066931901598,0.551651307869135,11.9104098730438));
#6823=CARTESIAN_POINT('Ctrl Pts',(6.07070001026945,0.720018713516863,11.9181349604511));
#6824=CARTESIAN_POINT('Ctrl Pts',(6.0508081358012,0.887733246863995,11.9258300925618));
#6825=CARTESIAN_POINT('Ctrl Pts',(6.02396424599014,1.05460294480008,11.9335252246725));
#6826=CARTESIAN_POINT('Ctrl Pts',(5.9902680884105,1.22004663495739,11.9412203567832));
#6827=CARTESIAN_POINT('Ctrl Pts',(5.95644218427393,1.38612736359938,11.9489451188864));
#6828=CARTESIAN_POINT('Ctrl Pts',(5.91569912895541,1.55082989587953,11.9566698809895));
#6829=CARTESIAN_POINT('Ctrl Pts',(5.86817609665716,1.71357371044303,11.9643946430927));
#6830=CARTESIAN_POINT('Ctrl Pts',(5.82066233461842,1.87628577877065,11.9721178983361));
#6831=CARTESIAN_POINT('Ctrl Pts',(5.76637132336642,2.03703958774093,11.9798411535794));
#6832=CARTESIAN_POINT('Ctrl Pts',(5.70549039388603,2.19526875980466,11.9875644088227));
#6833=CARTESIAN_POINT('Ctrl Pts',(5.64460711165028,2.35350404666548,11.9952879625328));
#6834=CARTESIAN_POINT('Ctrl Pts',(5.57713351168681,2.50921420418439,12.0030115162428));
#6835=CARTESIAN_POINT('Ctrl Pts',(5.50330574906832,2.66185112182698,12.0107350699528));
#6836=CARTESIAN_POINT('Ctrl Pts',(5.42948294505744,2.81447778768144,12.0184581049139));
#6837=CARTESIAN_POINT('Ctrl Pts',(5.34930697045353,2.96403134139491,12.0261811398751));
#6838=CARTESIAN_POINT('Ctrl Pts',(5.26306086232182,3.10998648260668,12.0339041748362));
#6839=CARTESIAN_POINT('Ctrl Pts',(5.1767918337319,3.25598041233643,12.0416292622435));
#6840=CARTESIAN_POINT('Ctrl Pts',(5.08444960756162,3.39837374449056,12.0493543496509));
#6841=CARTESIAN_POINT('Ctrl Pts',(4.9863621453097,3.53666765731846,12.0570794370582));
#6842=CARTESIAN_POINT('Ctrl Pts',(4.88865503332114,3.67442531275977,12.0647745691689));
#6843=CARTESIAN_POINT('Ctrl Pts',(4.78524736914535,3.80811504871322,12.0724697012796));
#6844=CARTESIAN_POINT('Ctrl Pts',(4.67650479358892,3.93727424470785,12.0801648333903));
#6845=CARTESIAN_POINT('Ctrl Pts',(4.56734350635197,4.06693076627836,12.0878895954935));
#6846=CARTESIAN_POINT('Ctrl Pts',(4.45276745753514,4.19206769022086,12.0956143575967));
#6847=CARTESIAN_POINT('Ctrl Pts',(4.33317484178046,4.31224087372921,12.1033391196999));
#6848=CARTESIAN_POINT('Ctrl Pts',(4.2136055548106,4.43239061520211,12.1110623749432));
#6849=CARTESIAN_POINT('Ctrl Pts',(4.08902187693335,4.54757832378144,12.1187856301866));
#6850=CARTESIAN_POINT('Ctrl Pts',(3.95985927996066,4.65739627317769,12.1265088854299));
#6851=CARTESIAN_POINT('Ctrl Pts',(3.83069169147391,4.76721846651028,12.13423243914));
#6852=CARTESIAN_POINT('Ctrl Pts',(3.69694506867638,4.87167027710725,12.14195599285));
#6853=CARTESIAN_POINT('Ctrl Pts',(3.55908901761198,4.97038337829324,12.1496795465601));
#6854=CARTESIAN_POINT('Ctrl Pts',(3.42124222558574,5.06908984945928,12.1574025815212));
#6855=CARTESIAN_POINT('Ctrl Pts',(3.27928681533585,5.16205819801352,12.1651256164823));
#6856=CARTESIAN_POINT('Ctrl Pts',(3.13372264815355,5.2489625572059,12.1728486514435));
#6857=CARTESIAN_POINT('Ctrl Pts',(2.98811979635727,5.33589001179087,12.1805737388508));
#6858=CARTESIAN_POINT('Ctrl Pts',(2.83890654240731,5.41675009231119,12.1882988262582));
#6859=CARTESIAN_POINT('Ctrl Pts',(2.68660952877123,5.49126167673838,12.1960239136655));
#6860=CARTESIAN_POINT('Ctrl Pts',(2.53490307184868,5.56548433024455,12.2037190457762));
#6861=CARTESIAN_POINT('Ctrl Pts',(2.38013702289031,5.63340752656996,12.2114141778868));
#6862=CARTESIAN_POINT('Ctrl Pts',(2.22285379179657,5.69479995985773,12.2191093099975));
#6863=CARTESIAN_POINT('Ctrl Pts',(2.06496494394432,5.7564287838032,12.2268340721007));
#6864=CARTESIAN_POINT('Ctrl Pts',(1.90448356028117,5.81149825078665,12.2345588342039));
#6865=CARTESIAN_POINT('Ctrl Pts',(1.74197179682505,5.85980885537797,12.2422835963071));
#6866=CARTESIAN_POINT('Ctrl Pts',(1.57949173433975,5.90811003607877,12.2500068515504));
#6867=CARTESIAN_POINT('Ctrl Pts',(1.41498238595332,5.94965489490004,12.2577301067937));
#6868=CARTESIAN_POINT('Ctrl Pts',(1.24902121901313,5.98429373919387,12.265453362037));
#6869=CARTESIAN_POINT('Ctrl Pts',(1.08305363847061,6.01893392211273,12.2731769157471));
#6870=CARTESIAN_POINT('Ctrl Pts',(0.915634436526519,6.04666748782398,12.2809004694571));
#6871=CARTESIAN_POINT('Ctrl Pts',(0.747352204760735,6.06739567232427,12.2886240231672));
#6872=CARTESIAN_POINT('Ctrl Pts',(0.579081275593571,6.08812246462559,12.2963470581283));
#6873=CARTESIAN_POINT('Ctrl Pts',(0.409947747182909,6.10184477854802,12.3040700930894));
#6874=CARTESIAN_POINT('Ctrl Pts',(0.240546464961092,6.10851561025219,12.3117931280505));
#6875=CARTESIAN_POINT('Ctrl Pts',(0.071100163258296,6.11518821477283,12.3195182154579));
#6876=CARTESIAN_POINT('Ctrl Pts',(-0.0986137176265944,6.11480557775733,
12.3272433028653));
#6877=CARTESIAN_POINT('Ctrl Pts',(-0.267998222194625,6.10737279977246,12.3349683902726));
#6878=CARTESIAN_POINT('Ctrl Pts',(-0.436725910494112,6.09996884360641,12.3426635223833));
#6879=CARTESIAN_POINT('Ctrl Pts',(-0.605126461881987,6.08556937133074,12.350358654494));
#6880=CARTESIAN_POINT('Ctrl Pts',(-0.772612908578236,6.06423077199395,12.3580537866047));
#6881=CARTESIAN_POINT('Ctrl Pts',(-0.940744259362647,6.04281000869571,12.3657785487079));
#6882=CARTESIAN_POINT('Ctrl Pts',(-1.10801399531538,6.01438895786286,12.3735033108111));
#6883=CARTESIAN_POINT('Ctrl Pts',(-1.27383302332941,5.9790613804489,12.3812280729142));
#6884=CARTESIAN_POINT('Ctrl Pts',(-1.43961970523002,5.94374069434191,12.3889513281576));
#6885=CARTESIAN_POINT('Ctrl Pts',(-1.60395593407248,5.90151623589398,12.396674583401));
#6886=CARTESIAN_POINT('Ctrl Pts',(-1.76626300336345,5.85253283335083,12.4043978386443));
#6887=CARTESIAN_POINT('Ctrl Pts',(-1.92857634504233,5.80354753783468,12.4121213923544));
#6888=CARTESIAN_POINT('Ctrl Pts',(-2.08886006570547,5.74780286331757,12.4198449460644));
#6889=CARTESIAN_POINT('Ctrl Pts',(-2.24655005613366,5.68549368197572,12.4275684997745));
#6890=CARTESIAN_POINT('Ctrl Pts',(-2.40422945538646,5.62318868560126,12.4352915347356));
#6891=CARTESIAN_POINT('Ctrl Pts',(-2.5593151782436,5.55432018120364,12.4430145696967));
#6892=CARTESIAN_POINT('Ctrl Pts',(-2.71126238739099,5.47913148493618,12.4507376046578));
#6893=CARTESIAN_POINT('Ctrl Pts',(-2.8632499774869,5.40392280678889,12.4584626920652));
#6894=CARTESIAN_POINT('Ctrl Pts',(-3.01209710195909,5.32239071916427,12.4661877794726));
#6895=CARTESIAN_POINT('Ctrl Pts',(-3.15728199886066,5.2348253019724,12.4739128668799));
#6896=CARTESIAN_POINT('Ctrl Pts',(-3.30190391745105,5.14759943408449,12.4816079989906));
#6897=CARTESIAN_POINT('Ctrl Pts',(-3.44289170908152,5.05438713274775,12.4893031311012));
#6898=CARTESIAN_POINT('Ctrl Pts',(-3.57975692019151,4.95551873721016,12.4969982632119));
#6899=CARTESIAN_POINT('Ctrl Pts',(-3.71714912877526,4.85626965037592,12.5047230253151));
#6900=CARTESIAN_POINT('Ctrl Pts',(-3.85043558859554,4.75128565004825,12.5124477874183));
#6901=CARTESIAN_POINT('Ctrl Pts',(-3.979143859599,4.64093090953911,12.5201725495215));
#6902=CARTESIAN_POINT('Ctrl Pts',(-4.10782702363795,4.53059769579382,12.5278958047648));
#6903=CARTESIAN_POINT('Ctrl Pts',(-4.2319335403864,4.41489603849501,12.5356190600081));
#6904=CARTESIAN_POINT('Ctrl Pts',(-4.35102452263382,4.29422998521727,12.5433423152515));
#6905=CARTESIAN_POINT('Ctrl Pts',(-4.47012010717551,4.17355926877634,12.5510658689615));
#6906=CARTESIAN_POINT('Ctrl Pts',(-4.5841995439207,4.04792399523236,12.5587894226715));
#6907=CARTESIAN_POINT('Ctrl Pts',(-4.69286070638614,3.91776517327889,12.5665129763816));
#6908=CARTESIAN_POINT('Ctrl Pts',(-4.80151457067522,3.78761509338206,12.5742360113427));
#6909=CARTESIAN_POINT('Ctrl Pts',(-4.9047506858181,3.65294231639115,12.5819590463039));
#6910=CARTESIAN_POINT('Ctrl Pts',(-5.00220702551001,3.51422117067755,12.589682081265));
#6911=CARTESIAN_POINT('Ctrl Pts',(-5.09968926485099,3.37546315892729,12.5974071686724));
#6912=CARTESIAN_POINT('Ctrl Pts',(-5.1913884753169,3.23265488684195,12.6051322560797));
#6913=CARTESIAN_POINT('Ctrl Pts',(-5.27698526683414,3.08630070733806,12.6128573434871));
#6914=CARTESIAN_POINT('Ctrl Pts',(-5.36225014271723,2.94051404023082,12.6205524755977));
#6915=CARTESIAN_POINT('Ctrl Pts',(-5.44145971200606,2.79120920225685,12.6282476077084));
#6916=CARTESIAN_POINT('Ctrl Pts',(-5.51434309483528,2.63890996340202,12.6359427398191));
#6917=CARTESIAN_POINT('Ctrl Pts',(-5.58725262910215,2.48655607774165,12.643640633036));
#6918=CARTESIAN_POINT('Ctrl Pts',(-5.65385889793136,2.33114811101626,12.651338526253));
#6919=CARTESIAN_POINT('Ctrl Pts',(-5.71392213225727,2.17322788243676,12.65903641947));
#6920=CARTESIAN_POINT('Ctrl Pts',(-5.77397291614694,2.01534038895316,12.6667327169998));
#6921=CARTESIAN_POINT('Ctrl Pts',(-5.8274832574358,1.85494197281612,12.6744290145297));
#6922=CARTESIAN_POINT('Ctrl Pts',(-5.87426190130256,1.69259347671116,12.6821253120596));
#6923=CARTESIAN_POINT('Ctrl Pts',(-5.92104057981929,1.53024486035111,12.6898216152902));
#6924=CARTESIAN_POINT('Ctrl Pts',(-5.96108745831491,1.36594646882379,12.6975179185209));
#6925=CARTESIAN_POINT('Ctrl Pts',(-5.99426125300097,1.20027396592247,12.7052142217516));
#6926=CARTESIAN_POINT('Ctrl Pts',(-6.02743352763924,1.03460905425766,12.712910172332));
#6927=CARTESIAN_POINT('Ctrl Pts',(-6.05373328646756,0.86757047246313,12.7206061229124));
#6928=CARTESIAN_POINT('Ctrl Pts',(-6.07307039063346,0.69974394810615,12.7283020734927));
#6929=CARTESIAN_POINT('Ctrl Pts',(-6.0924113036645,0.531884366648455,12.7359995399587));
#6930=CARTESIAN_POINT('Ctrl Pts',(-6.10478678589844,0.363236851908962,12.7436970064247));
#6931=CARTESIAN_POINT('Ctrl Pts',(-6.11015850685667,0.194392858889112,12.7513944728907));
#6932=CARTESIAN_POINT('Ctrl Pts',(-6.11222055291481,0.129578604210711,12.754349304407));
#6933=CARTESIAN_POINT('Ctrl Pts',(-6.1132510932271,0.0647354281208469,12.7573041359232));
#6934=CARTESIAN_POINT('Ctrl Pts',(-6.11324999912966,-0.000103156033837302,
12.7602589674395));
#6935=CARTESIAN_POINT('Ctrl Pts',(-6.11362854109631,-0.000103162421420267,
12.7602589674395));
#6936=CARTESIAN_POINT('Ctrl Pts',(-6.11371354863409,-0.107106860351694,
12.7651350504351));
#6937=CARTESIAN_POINT('Ctrl Pts',(-6.08482838106602,-1.23042505733209,12.8163259589664));
#6938=CARTESIAN_POINT('Ctrl Pts',(-5.42822856457523,-3.3384373253954,12.9138316930335));
#6939=CARTESIAN_POINT('Ctrl Pts',(-3.16946315476177,-5.52859226525806,13.0527761696406));
#6940=CARTESIAN_POINT('Ctrl Pts',(-0.138148106431394,-6.37116506029729,
13.1917206462478));
#6941=CARTESIAN_POINT('Ctrl Pts',(2.26894793050691,-5.81326278514897,13.3008410282742));
#6942=CARTESIAN_POINT('Ctrl Pts',(3.43573368210399,-5.06927082860839,13.363646584765));
#6943=CARTESIAN_POINT('Ctrl Pts',(3.72270802987534,-4.84860079634452,13.3801373157199));
#6944=CARTESIAN_POINT('',(-6.11324999800781,-0.000156069087590843,12.6147410325606));
#6945=CARTESIAN_POINT('Ctrl Pts',(-6.11331623078485,-0.000156070778496338,
12.6147410325606));
#6946=CARTESIAN_POINT('Ctrl Pts',(-6.11353700954689,-0.21382808103462,12.6244764787917));
#6947=CARTESIAN_POINT('Ctrl Pts',(-6.05029720305683,-1.44388040587524,12.6805267505586));
#6948=CARTESIAN_POINT('Ctrl Pts',(-5.24613718046346,-3.6178548867268,12.7828918478612));
#6949=CARTESIAN_POINT('Ctrl Pts',(-2.8758824236554,-5.68683827649109,12.9218363244684));
#6950=CARTESIAN_POINT('Ctrl Pts',(0.195362317363167,-6.36966740596466,13.0607808010756));
#6951=CARTESIAN_POINT('Ctrl Pts',(2.46424006555832,-5.71701172825789,13.1650423969484));
#6952=CARTESIAN_POINT('Ctrl Pts',(3.52053820541315,-5.00452290254849,13.2229891672854));
#6953=CARTESIAN_POINT('Ctrl Pts',(3.72288481551393,-4.8488307603735,13.2346211120867));
#6954=CARTESIAN_POINT('Ctrl Pts',(3.72292453512039,-4.84888218750453,11.484610425966));
#6955=CARTESIAN_POINT('Ctrl Pts',(3.86158194725542,-4.74242237642805,11.4925739480377));
#6956=CARTESIAN_POINT('Ctrl Pts',(3.99566183533874,-4.63001736623254,11.5005374701095));
#6957=CARTESIAN_POINT('Ctrl Pts',(4.12466559379199,-4.51209034726573,11.5085009921812));
#6958=CARTESIAN_POINT('Ctrl Pts',(4.25366935224525,-4.39416332829891,11.516464514253));
#6959=CARTESIAN_POINT('Ctrl Pts',(4.37759671475846,-4.27071455614831,11.5244280363247));
#6960=CARTESIAN_POINT('Ctrl Pts',(4.49598948302034,-4.14221005395315,11.5323915583965));
#6961=CARTESIAN_POINT('Ctrl Pts',(4.61083263424427,-4.01755833581853,11.5401163204997));
#6962=CARTESIAN_POINT('Ctrl Pts',(4.72050895726609,-3.88810554571865,11.5478410826029));
#6963=CARTESIAN_POINT('Ctrl Pts',(4.82462811457528,-3.75430274732203,11.5555658447061));
#6964=CARTESIAN_POINT('Ctrl Pts',(4.92872696148876,-3.62052604967242,11.5632890999494));
#6965=CARTESIAN_POINT('Ctrl Pts',(5.02727061120222,-3.48240128685783,11.5710123551928));
#6966=CARTESIAN_POINT('Ctrl Pts',(5.11990955609688,-3.34041190572179,11.5787356104362));
#6967=CARTESIAN_POINT('Ctrl Pts',(5.21255208104128,-3.19841703737895,11.5864591641462));
#6968=CARTESIAN_POINT('Ctrl Pts',(5.29928926805948,-3.05255751511587,11.5941827178563));
#6969=CARTESIAN_POINT('Ctrl Pts',(5.37981500201618,-2.90334567466253,11.6019062715663));
#6970=CARTESIAN_POINT('Ctrl Pts',(5.46033532749914,-2.75414385595356,11.6096293065274));
#6971=CARTESIAN_POINT('Ctrl Pts',(5.53464488425912,-2.60159044856381,11.6173523414886));
#6972=CARTESIAN_POINT('Ctrl Pts',(5.60248349593993,-2.44622244291494,11.6250753764497));
#6973=CARTESIAN_POINT('Ctrl Pts',(5.6703401361683,-2.29081314721885,11.6328004638571));
#6974=CARTESIAN_POINT('Ctrl Pts',(5.73172226604339,-2.13258804836254,11.6405255512644));
#6975=CARTESIAN_POINT('Ctrl Pts',(5.78641747607167,-1.97210505681425,11.6482506386718));
#6976=CARTESIAN_POINT('Ctrl Pts',(5.84090059642908,-1.81224436445526,11.6559457707824));
#6977=CARTESIAN_POINT('Ctrl Pts',(5.8887484938185,-1.65014356487504,11.6636409028931));
#6978=CARTESIAN_POINT('Ctrl Pts',(5.92980016652284,-1.4863699228677,11.6713360350037));
#6979=CARTESIAN_POINT('Ctrl Pts',(5.97100990808674,-1.32196567287013,11.6790607971069));
#6980=CARTESIAN_POINT('Ctrl Pts',(6.00538554968506,-1.15581743796826,11.6867855592101));
#6981=CARTESIAN_POINT('Ctrl Pts',(6.03280012781083,-0.988508057825365,11.6945103213133));
#6982=CARTESIAN_POINT('Ctrl Pts',(6.06020935820837,-0.821231314518607,11.7022335765566));
#6983=CARTESIAN_POINT('Ctrl Pts',(6.08066018338688,-0.652794190491557,11.7099568317999));
#6984=CARTESIAN_POINT('Ctrl Pts',(6.09407698669119,-0.483788427704495,11.7176800870432));
#6985=CARTESIAN_POINT('Ctrl Pts',(6.10749430849052,-0.314776133656291,11.7254036407533));
#6986=CARTESIAN_POINT('Ctrl Pts',(6.11387703543591,-0.145195472484922,11.7331271944633));
#6987=CARTESIAN_POINT('Ctrl Pts',(6.11320147623289,0.0243572059971047,11.7408507481733));
#6988=CARTESIAN_POINT('Ctrl Pts',(6.1125259624035,0.193898496552499,11.7485737831345));
#6989=CARTESIAN_POINT('Ctrl Pts',(6.10479311237982,0.363411491224797,11.7562968180956));
#6990=CARTESIAN_POINT('Ctrl Pts',(6.0900313704341,0.532300168728613,11.7640198530568));
#6991=CARTESIAN_POINT('Ctrl Pts',(6.07526570546054,0.701233729484569,11.7717449404641));
#6992=CARTESIAN_POINT('Ctrl Pts',(6.05346744134481,0.869542325395739,11.7794700278715));
#6993=CARTESIAN_POINT('Ctrl Pts',(6.02471697645032,1.0366344178018,11.7871951152789));
#6994=CARTESIAN_POINT('Ctrl Pts',(5.99607799621096,1.20307858314427,11.7948902473895));
#6995=CARTESIAN_POINT('Ctrl Pts',(5.96054072066098,1.36831536039421,11.8025853795002));
#6996=CARTESIAN_POINT('Ctrl Pts',(5.91823516605736,1.53176959159725,11.8102805116109));
#6997=CARTESIAN_POINT('Ctrl Pts',(5.87576671454066,1.69585320090303,11.8180052737141));
#6998=CARTESIAN_POINT('Ctrl Pts',(5.82646268805614,1.85819861558642,11.8257300358173));
#6999=CARTESIAN_POINT('Ctrl Pts',(5.77049044417457,2.01823328586911,11.8334547979205));
#7000=CARTESIAN_POINT('Ctrl Pts',(5.71452911872981,2.17823673838537,11.8411780531639));
#7001=CARTESIAN_POINT('Ctrl Pts',(5.65190227593882,2.33593004694149,11.8489013084072));
#7002=CARTESIAN_POINT('Ctrl Pts',(5.58282662150262,2.4907574102553,11.8566245636506));
#7003=CARTESIAN_POINT('Ctrl Pts',(5.51374829762438,2.64559075690253,11.8643481173606));
#7004=CARTESIAN_POINT('Ctrl Pts',(5.43822078891153,2.7975576456458,11.8720716710707));
#7005=CARTESIAN_POINT('Ctrl Pts',(5.3565086026111,2.94612307153881,11.8797952247807));
#7006=CARTESIAN_POINT('Ctrl Pts',(5.27480190447206,3.09467851910336,11.8875182597419));
#7007=CARTESIAN_POINT('Ctrl Pts',(5.18691151276608,3.23983268327991,11.895241294703));
#7008=CARTESIAN_POINT('Ctrl Pts',(5.09314755916535,3.38107579079027,11.9029643296641));
#7009=CARTESIAN_POINT('Ctrl Pts',(4.99935868719056,3.52235643456537,11.9106894170714));
#7010=CARTESIAN_POINT('Ctrl Pts',(4.89969330778148,3.65972367929024,11.9184145044788));
#7011=CARTESIAN_POINT('Ctrl Pts',(4.79450503023508,3.79269654435344,11.9261395918862));
#7012=CARTESIAN_POINT('Ctrl Pts',(4.68972463753176,3.92515378526663,11.9338347239968));
#7013=CARTESIAN_POINT('Ctrl Pts',(4.57946432140999,4.05325044095243,11.9415298561074));
#7014=CARTESIAN_POINT('Ctrl Pts',(4.46411342492558,4.17654365377631,11.9492249882181));
#7015=CARTESIAN_POINT('Ctrl Pts',(4.34831837151762,4.30031160529552,11.9569497503213));
#7016=CARTESIAN_POINT('Ctrl Pts',(4.22735242442935,4.41928286376296,11.9646745124245));
#7017=CARTESIAN_POINT('Ctrl Pts',(4.10163646927133,4.53303472702818,11.9723992745277));
#7018=CARTESIAN_POINT('Ctrl Pts',(3.9759450373703,4.64676440085713,11.980122529771));
#7019=CARTESIAN_POINT('Ctrl Pts',(3.84550568111629,4.75527649852969,11.9878457850144));
#7020=CARTESIAN_POINT('Ctrl Pts',(3.71077460703088,4.85818663477586,11.9955690402577));
#7021=CARTESIAN_POINT('Ctrl Pts',(3.57603832623683,4.96110074800433,12.0032925939678));
#7022=CARTESIAN_POINT('Ctrl Pts',(3.43701024517634,5.05841227108009,12.0110161476778));
#7023=CARTESIAN_POINT('Ctrl Pts',(3.29417859658111,5.14977795019619,12.0187397013879));
#7024=CARTESIAN_POINT('Ctrl Pts',(3.15135654120784,5.24113749277849,12.026462736349));
#7025=CARTESIAN_POINT('Ctrl Pts',(3.00473169653404,5.32655181977587,12.0341857713101));
#7026=CARTESIAN_POINT('Ctrl Pts',(2.85482028772225,5.40572166202714,12.0419088062712));
#7027=CARTESIAN_POINT('Ctrl Pts',(2.70486903898894,5.48491254417341,12.0496338936786));
#7028=CARTESIAN_POINT('Ctrl Pts',(2.55162976022748,5.55785547543274,12.0573589810859));
#7029=CARTESIAN_POINT('Ctrl Pts',(2.39564308018388,5.6242972712035,12.0650840684933));
#7030=CARTESIAN_POINT('Ctrl Pts',(2.24026126414162,5.69048142798587,12.072779200604));
#7031=CARTESIAN_POINT('Ctrl Pts',(2.08215361579399,5.75021468541692,12.0804743327146));
#7032=CARTESIAN_POINT('Ctrl Pts',(1.92187390348632,5.80329443175152,12.0881694648253));
#7033=CARTESIAN_POINT('Ctrl Pts',(1.76097703651381,5.85657856086538,12.0958942269285));
#7034=CARTESIAN_POINT('Ctrl Pts',(1.59783435105387,5.90317668182732,12.1036189890317));
#7035=CARTESIAN_POINT('Ctrl Pts',(1.43301767081955,5.94291897282968,12.1113437511349));
#7036=CARTESIAN_POINT('Ctrl Pts',(1.26823314117254,5.98265351135215,12.1190670063782));
#7037=CARTESIAN_POINT('Ctrl Pts',(1.10177557623251,6.0155348141777,12.1267902616215));
#7038=CARTESIAN_POINT('Ctrl Pts',(0.934229484010322,6.04144360510845,12.1345135168649));
#7039=CARTESIAN_POINT('Ctrl Pts',(0.766676916936759,6.06735339728948,12.1422370705749));
#7040=CARTESIAN_POINT('Ctrl Pts',(0.59803605099373,6.08629008603538,12.149960624285));
#7041=CARTESIAN_POINT('Ctrl Pts',(0.428899838748377,6.0981858360353,12.157684177995));
#7042=CARTESIAN_POINT('Ctrl Pts',(0.259774986458183,6.1100807870627,12.1654072129562));
#7043=CARTESIAN_POINT('Ctrl Pts',(0.0901551706205841,6.11493572346633,12.1731302479173));
#7044=CARTESIAN_POINT('Ctrl Pts',(-0.0793631188539132,6.11273482639855,
12.1808532828785));
#7045=CARTESIAN_POINT('Ctrl Pts',(-0.248926458904212,6.11053334442823,12.1885783702858));
#7046=CARTESIAN_POINT('Ctrl Pts',(-0.418387901524658,6.10127228395309,12.1963034576932));
#7047=CARTESIAN_POINT('Ctrl Pts',(-0.587151575582146,6.08498796956834,12.2040285451006));
#7048=CARTESIAN_POINT('Ctrl Pts',(-0.755260840741822,6.06876680029042,12.2117236772112));
#7049=CARTESIAN_POINT('Ctrl Pts',(-0.922677431494252,6.04557680999582,12.2194188093218));
#7050=CARTESIAN_POINT('Ctrl Pts',(-1.08881813401474,6.01550501899389,12.2271139414324));
#7051=CARTESIAN_POINT('Ctrl Pts',(-1.25559855885688,5.98531743700477,12.2348387035356));
#7052=CARTESIAN_POINT('Ctrl Pts',(-1.4211523137012,5.94818423147259,12.2425634656388));
#7053=CARTESIAN_POINT('Ctrl Pts',(-1.58489601749832,5.9042298546227,12.250288227742));
#7054=CARTESIAN_POINT('Ctrl Pts',(-1.74860778001208,5.86028405189916,12.2580114829853));
#7055=CARTESIAN_POINT('Ctrl Pts',(-1.91050989010417,5.80951981499163,12.2657347382286));
#7056=CARTESIAN_POINT('Ctrl Pts',(-2.07003201081014,5.75211205008398,12.2734579934719));
#7057=CARTESIAN_POINT('Ctrl Pts',(-2.2295602962801,5.69470206664187,12.281181547182));
#7058=CARTESIAN_POINT('Ctrl Pts',(-2.3867081087786,5.63064814503191,12.288905100892));
#7059=CARTESIAN_POINT('Ctrl Pts',(-2.54092230678068,5.56017440314639,12.2966286546021));
#7060=CARTESIAN_POINT('Ctrl Pts',(-2.69512614705694,5.48970539459741,12.3043516895632));
#7061=CARTESIAN_POINT('Ctrl Pts',(-2.84639647885681,5.41281756038992,12.3120747245243));
#7062=CARTESIAN_POINT('Ctrl Pts',(-2.99420194061909,5.32978238779904,12.3197977594854));
#7063=CARTESIAN_POINT('Ctrl Pts',(-3.14204668263394,5.24672514807673,12.3275228468927));
#7064=CARTESIAN_POINT('Ctrl Pts',(-3.28642443703427,5.15751745888855,12.3352479343001));
#7065=CARTESIAN_POINT('Ctrl Pts',(-3.42682933257148,5.06247629998677,12.3429730217074));
#7066=CARTESIAN_POINT('Ctrl Pts',(-3.56668978504021,4.96780367880574,12.3506681538182));
#7067=CARTESIAN_POINT('Ctrl Pts',(-3.70260789424474,4.8673429496621,12.3583632859289));
#7068=CARTESIAN_POINT('Ctrl Pts',(-3.8341131579617,4.7614495539116,12.3660584180396));
#7069=CARTESIAN_POINT('Ctrl Pts',(-3.96612478075329,4.65514841720559,12.3737831801428));
#7070=CARTESIAN_POINT('Ctrl Pts',(-4.09373624316244,4.54333502195203,12.381507942246));
#7071=CARTESIAN_POINT('Ctrl Pts',(-4.2164948046448,4.42639775945445,12.3892327043492));
#7072=CARTESIAN_POINT('Ctrl Pts',(-4.33922941976432,4.30948330776602,12.3969559595925));
#7073=CARTESIAN_POINT('Ctrl Pts',(-4.4571127935254,4.18744720166812,12.4046792148358));
#7074=CARTESIAN_POINT('Ctrl Pts',(-4.56972777838454,4.06071589673061,12.4124024700791));
#7075=CARTESIAN_POINT('Ctrl Pts',(-4.68234711527243,3.93397969423632,12.4201260237892));
#7076=CARTESIAN_POINT('Ctrl Pts',(-4.78969744237316,3.8025481640848,12.4278495774992));
#7077=CARTESIAN_POINT('Ctrl Pts',(-4.89140025622809,3.66688274913063,12.4355731312092));
#7078=CARTESIAN_POINT('Ctrl Pts',(-4.99309623926017,3.53122644608183,12.4432961661703));
#7079=CARTESIAN_POINT('Ctrl Pts',(-5.08914527799931,3.39133708090647,12.4510192011314));
#7080=CARTESIAN_POINT('Ctrl Pts',(-5.17921065743964,3.24770727257917,12.4587422360925));
#7081=CARTESIAN_POINT('Ctrl Pts',(-5.26929997233436,3.10403929370568,12.4664673234999));
#7082=CARTESIAN_POINT('Ctrl Pts',(-5.35340227999785,2.9566291528682,12.4741924109073));
#7083=CARTESIAN_POINT('Ctrl Pts',(-5.43122501406473,2.80599722186206,12.4819174983146));
#7084=CARTESIAN_POINT('Ctrl Pts',(-5.50874597768429,2.65594939093599,12.4896126304254));
#7085=CARTESIAN_POINT('Ctrl Pts',(-5.58003586663959,2.50270500362402,12.4973077625361));
#7086=CARTESIAN_POINT('Ctrl Pts',(-5.6448515741856,2.34680128428343,12.5050028946468));
#7087=CARTESIAN_POINT('Ctrl Pts',(-5.70967202129114,2.19088616469765,12.5126985894535));
#7088=CARTESIAN_POINT('Ctrl Pts',(-5.76804186624444,2.03225215979232,12.5203942842602));
#7089=CARTESIAN_POINT('Ctrl Pts',(-5.81975006970807,1.87145256114946,12.5280899790669));
#7090=CARTESIAN_POINT('Ctrl Pts',(-5.87145192307247,1.71067270972931,12.5357847287929));
#7091=CARTESIAN_POINT('Ctrl Pts',(-5.91649366547352,1.54772810027992,12.5434794785189));
#7092=CARTESIAN_POINT('Ctrl Pts',(-5.95471365910835,1.3831886351935,12.5511742282449));
#7093=CARTESIAN_POINT('Ctrl Pts',(-5.99292850060074,1.21867135040279,12.558867940701));
#7094=CARTESIAN_POINT('Ctrl Pts',(-6.02432335703991,1.05255995264312,12.5665616531572));
#7095=CARTESIAN_POINT('Ctrl Pts',(-6.04878732671191,0.885436298504514,12.5742553656133));
#7096=CARTESIAN_POINT('Ctrl Pts',(-6.07325456934187,0.718290285415124,12.5819501073872));
#7097=CARTESIAN_POINT('Ctrl Pts',(-6.09078902373148,0.550132063452321,12.5896448491611));
#7098=CARTESIAN_POINT('Ctrl Pts',(-6.10133135165719,0.381551175840124,12.5973395909349));
#7099=CARTESIAN_POINT('Ctrl Pts',(-6.10927841080438,0.254470867356085,12.6031400714768));
#7100=CARTESIAN_POINT('Ctrl Pts',(-6.11325324810064,0.127150563502077,12.6089405520187));
#7101=CARTESIAN_POINT('Ctrl Pts',(-6.11324999800781,-0.000156069087590843,
12.6147410325606));
#7102=CARTESIAN_POINT('Origin',(0.,0.,-3.86474103256053));
#7103=CARTESIAN_POINT('',(3.72292453512039,-4.84888218750452,9.73461637809168));
#7104=CARTESIAN_POINT('',(3.72292453512037,-4.84888218750454,9.88013638533173));
#7105=CARTESIAN_POINT('',(3.72292453512038,-4.84888218750453,-3.86474103256053));
#7106=CARTESIAN_POINT('',(-6.1132499981976,0.000148448865203969,11.0102589674072));
#7107=CARTESIAN_POINT('Ctrl Pts',(3.72292453512037,-4.84888218750454,9.88013638533173));
#7108=CARTESIAN_POINT('Ctrl Pts',(3.85737370293807,-4.74565342544368,9.88785964524372));
#7109=CARTESIAN_POINT('Ctrl Pts',(3.98754260366794,-4.63681706701032,9.89558290515572));
#7110=CARTESIAN_POINT('Ctrl Pts',(4.11297118110572,-4.52275288136482,9.90330616506772));
#7111=CARTESIAN_POINT('Ctrl Pts',(4.23841654062291,-4.4086734341716,9.91103045833562));
#7112=CARTESIAN_POINT('Ctrl Pts',(4.35912007031516,-4.28936497025535,9.91875475160352));
#7113=CARTESIAN_POINT('Ctrl Pts',(4.47465630588625,-4.16524627203391,9.92647904487143));
#7114=CARTESIAN_POINT('Ctrl Pts',(4.59017373171417,-4.04114778081355,9.9342020805947));
#7115=CARTESIAN_POINT('Ctrl Pts',(4.70052533083415,-3.91224085440095,9.94192511631798));
#7116=CARTESIAN_POINT('Ctrl Pts',(4.80532400580619,-3.77897959265762,9.94964815204125));
#7117=CARTESIAN_POINT('Ctrl Pts',(4.91015056888418,-3.64568286859392,9.95737324295118));
#7118=CARTESIAN_POINT('Ctrl Pts',(5.00942105723682,-3.50802974169527,9.96509833386111));
#7119=CARTESIAN_POINT('Ctrl Pts',(5.10278932642359,-3.36650659477113,9.97282342477104));
#7120=CARTESIAN_POINT('Ctrl Pts',(5.19615351356833,-3.22498963521062,9.98054817794154));
#7121=CARTESIAN_POINT('Ctrl Pts',(5.28361582994328,-3.07960326306029,9.98827293111204));
#7122=CARTESIAN_POINT('Ctrl Pts',(5.36487414676132,-2.93086181044279,9.99599768428254));
#7123=CARTESIAN_POINT('Ctrl Pts',(5.44613255754426,-2.78212018582472,10.0037224463857));
#7124=CARTESIAN_POINT('Ctrl Pts',(5.52121573322926,-2.62997079402401,10.0114472084889));
#7125=CARTESIAN_POINT('Ctrl Pts',(5.58985411552551,-2.47494576296988,10.0191719705921));
#7126=CARTESIAN_POINT('Ctrl Pts',(5.65847910861668,-2.31995097245847,10.0268952258355));
#7127=CARTESIAN_POINT('Ctrl Pts',(5.7206616886098,-2.1620819516009,10.0346184810788));
#7128=CARTESIAN_POINT('Ctrl Pts',(5.77617975100661,-2.00189236637769,10.0423417363221));
#7129=CARTESIAN_POINT('Ctrl Pts',(5.83169995890988,-1.84169659059638,10.0500652900322));
#7130=CARTESIAN_POINT('Ctrl Pts',(5.88055502631713,-1.67918036914357,10.0577888437422));
#7131=CARTESIAN_POINT('Ctrl Pts',(5.92257194317969,-1.51491489541849,10.0655123974523));
#7132=CARTESIAN_POINT('Ctrl Pts',(5.96458603799538,-1.35066045450827,10.0732354324134));
#7133=CARTESIAN_POINT('Ctrl Pts',(5.99976282282497,-1.18465730351075,10.0809584673745));
#7134=CARTESIAN_POINT('Ctrl Pts',(6.02797982783107,-1.01748943864871,10.0886815023356));
#7135=CARTESIAN_POINT('Ctrl Pts',(6.05620433168782,-0.850277147850894,10.096406589743));
#7136=CARTESIAN_POINT('Ctrl Pts',(6.07746530482299,-0.681899837035541,10.1041316771503));
#7137=CARTESIAN_POINT('Ctrl Pts',(6.09169168742327,-0.512950239183375,10.1118567645577));
#7138=CARTESIAN_POINT('Ctrl Pts',(6.10586290488572,-0.344655771177826,10.1195518966684));
#7139=CARTESIAN_POINT('Ctrl Pts',(6.11305399632487,-0.175793760313002,10.127247028779));
#7140=CARTESIAN_POINT('Ctrl Pts',(6.11324604529533,-0.00695357325546233,
10.1349421608897));
#7141=CARTESIAN_POINT('Ctrl Pts',(6.11343883374751,0.162536730448309,10.1426669229929));
#7142=CARTESIAN_POINT('Ctrl Pts',(6.10657861157093,0.332065070403449,10.1503916850961));
#7143=CARTESIAN_POINT('Ctrl Pts',(6.09268325815753,0.501035206614228,10.1581164471993));
#7144=CARTESIAN_POINT('Ctrl Pts',(6.07879061529368,0.669972382027743,10.1658397024426));
#7145=CARTESIAN_POINT('Ctrl Pts',(6.05786560545085,0.838351255299317,10.1735629576859));
#7146=CARTESIAN_POINT('Ctrl Pts',(6.02997808286865,1.00557937659029,10.1812862129293));
#7147=CARTESIAN_POINT('Ctrl Pts',(6.00208948256765,1.17281396044494,10.1890097666393));
#7148=CARTESIAN_POINT('Ctrl Pts',(5.96723787932955,1.33889739007713,10.1967333203494));
#7149=CARTESIAN_POINT('Ctrl Pts',(5.92554462414148,1.50324531258475,10.2044568740594));
#7150=CARTESIAN_POINT('Ctrl Pts',(5.88385416926168,1.6675821967399,10.2121799090205));
#7151=CARTESIAN_POINT('Ctrl Pts',(5.8353230599455,1.83018349981151,10.2199029439816));
#7152=CARTESIAN_POINT('Ctrl Pts',(5.78012315310418,1.99047780631912,10.2276259789428));
#7153=CARTESIAN_POINT('Ctrl Pts',(5.72490857653243,2.15081471207011,10.2353510663501));
#7154=CARTESIAN_POINT('Ctrl Pts',(5.66302176220145,2.3088430955587,10.2430761537575));
#7155=CARTESIAN_POINT('Ctrl Pts',(5.59468389142722,2.46400846538822,10.2508012411648));
#7156=CARTESIAN_POINT('Ctrl Pts',(5.5266110119838,2.61857215598217,10.2584963732755));
#7157=CARTESIAN_POINT('Ctrl Pts',(5.45213717255982,2.77029472434611,10.2661915053862));
#7158=CARTESIAN_POINT('Ctrl Pts',(5.37152773238069,2.91864958204393,10.2738866374969));
#7159=CARTESIAN_POINT('Ctrl Pts',(5.29060790674295,3.06757567792972,10.2816113996001));
#7160=CARTESIAN_POINT('Ctrl Pts',(5.20347645069713,3.21316080788342,10.2893361617033));
#7161=CARTESIAN_POINT('Ctrl Pts',(5.11043432325565,3.35488995202385,10.2970609238065));
#7162=CARTESIAN_POINT('Ctrl Pts',(5.01741034542794,3.49659144923383,10.3047841790498));
#7163=CARTESIAN_POINT('Ctrl Pts',(4.91847817064782,3.63443819672686,10.3125074342932));
#7164=CARTESIAN_POINT('Ctrl Pts',(4.81398258507628,3.7679433691448,10.3202306895365));
#7165=CARTESIAN_POINT('Ctrl Pts',(4.70948296125224,3.90145370089646,10.3279542432465));
#7166=CARTESIAN_POINT('Ctrl Pts',(4.5994196886256,4.03062186982901,10.3356777969566));
#7167=CARTESIAN_POINT('Ctrl Pts',(4.48417890018445,4.15499279826579,10.3434013506666));
#7168=CARTESIAN_POINT('Ctrl Pts',(4.36894585183767,4.27935537338655,10.3511243856278));
#7169=CARTESIAN_POINT('Ctrl Pts',(4.24853619900322,4.39892112030591,10.3588474205889));
#7170=CARTESIAN_POINT('Ctrl Pts',(4.12337423559869,4.51327048554603,10.36657045555));
#7171=CARTESIAN_POINT('Ctrl Pts',(3.99817900959706,4.62765023986573,10.3742955429574));
#7172=CARTESIAN_POINT('Ctrl Pts',(3.86822918200473,4.736810626842,10.3820206303647));
#7173=CARTESIAN_POINT('Ctrl Pts',(3.73398426281008,4.8403705527146,10.3897457177721));
#7174=CARTESIAN_POINT('Ctrl Pts',(3.60025990036412,4.94352890794579,10.3974408498828));
#7175=CARTESIAN_POINT('Ctrl Pts',(3.46227396382763,5.04112999312155,10.4051359819934));
#7176=CARTESIAN_POINT('Ctrl Pts',(3.32051140737212,5.13283835280361,10.4128311141041));
#7177=CARTESIAN_POINT('Ctrl Pts',(3.17820299628681,5.22489983417008,10.4205558762073));
#7178=CARTESIAN_POINT('Ctrl Pts',(3.03203840619653,5.31105570048242,10.4282806383105));
#7179=CARTESIAN_POINT('Ctrl Pts',(2.88252831764012,5.39099768693169,10.4360054004137));
#7180=CARTESIAN_POINT('Ctrl Pts',(2.73304739383332,5.47092407919571,10.443728655657));
#7181=CARTESIAN_POINT('Ctrl Pts',(2.58022255304897,5.5446388608911,10.4514519109004));
#7182=CARTESIAN_POINT('Ctrl Pts',(2.42458947250475,5.61187949374531,10.4591751661437));
#7183=CARTESIAN_POINT('Ctrl Pts',(2.26895037748954,5.67912272512699,10.4668987198538));
#7184=CARTESIAN_POINT('Ctrl Pts',(2.11050311490458,5.73989117768262,10.4746222735638));
#7185=CARTESIAN_POINT('Ctrl Pts',(1.94980448067649,5.79396997313879,10.4823458272738));
#7186=CARTESIAN_POINT('Ctrl Pts',(1.78911663969801,5.84804513641761,10.490068862235));
#7187=CARTESIAN_POINT('Ctrl Pts',(1.6261780300826,5.89543144064883,10.4977918971961));
#7188=CARTESIAN_POINT('Ctrl Pts',(1.46156196204963,5.93596345959016,10.5055149321572));
#7189=CARTESIAN_POINT('Ctrl Pts',(1.29690214623741,5.97650625017632,10.5132400195646));
#7190=CARTESIAN_POINT('Ctrl Pts',(1.13056428863167,6.01019103759166,10.520965106972));
#7191=CARTESIAN_POINT('Ctrl Pts',(0.963134223349178,6.03690301647406,10.5286901943793));
#7192=CARTESIAN_POINT('Ctrl Pts',(0.796353395676169,6.06351141526596,10.53638532649));
#7193=CARTESIAN_POINT('Ctrl Pts',(0.628489129067831,6.0832009684698,10.5440804586006));
#7194=CARTESIAN_POINT('Ctrl Pts',(0.460127766134396,6.09590912016675,10.5517755907113));
#7195=CARTESIAN_POINT('Ctrl Pts',(0.291118130259757,6.1086662044141,10.5595003528145));
#7196=CARTESIAN_POINT('Ctrl Pts',(0.121547701892418,6.11439250510157,10.5672251149177));
#7197=CARTESIAN_POINT('Ctrl Pts',(-0.0479875941549688,6.11306165135828,
10.5749498770209));
#7198=CARTESIAN_POINT('Ctrl Pts',(-0.217489819160041,6.111731057223,10.5826731322642));
#7199=CARTESIAN_POINT('Ctrl Pts',(-0.386956608795583,6.10334605801405,10.5903963875075));
#7200=CARTESIAN_POINT('Ctrl Pts',(-0.555791964925009,6.08793239566807,10.5981196427509));
#7201=CARTESIAN_POINT('Ctrl Pts',(-0.724633845730077,6.07251813765807,10.6058431964609));
#7202=CARTESIAN_POINT('Ctrl Pts',(-0.892843928233819,6.05007469784273,10.613566750171));
#7203=CARTESIAN_POINT('Ctrl Pts',(-1.0598304713475,6.02067977345609,10.621290303881));
#7204=CARTESIAN_POINT('Ctrl Pts',(-1.22680579888697,5.99128682336601,10.6290133388421));
#7205=CARTESIAN_POINT('Ctrl Pts',(-1.39255743933224,5.95494337799063,10.6367363738032));
#7206=CARTESIAN_POINT('Ctrl Pts',(-1.55650280926096,5.91177846060411,10.6444594087644));
#7207=CARTESIAN_POINT('Ctrl Pts',(-1.72049174872666,5.86860207186305,10.6521844961717));
#7208=CARTESIAN_POINT('Ctrl Pts',(-1.8826731512105,5.81860066723842,10.6599095835791));
#7209=CARTESIAN_POINT('Ctrl Pts',(-2.04247765423843,5.76195371331953,10.6676346709864));
#7210=CARTESIAN_POINT('Ctrl Pts',(-2.20166248902901,5.70552641727898,10.6753298030971));
#7211=CARTESIAN_POINT('Ctrl Pts',(-2.35848854175393,5.64250515343708,10.6830249352078));
#7212=CARTESIAN_POINT('Ctrl Pts',(-2.5124110010795,5.57311551326139,10.6907200673185));
#7213=CARTESIAN_POINT('Ctrl Pts',(-2.6669261365608,5.50345868930129,10.6984448294217));
#7214=CARTESIAN_POINT('Ctrl Pts',(-2.81856998609195,5.42735965122814,10.7061695915249));
#7215=CARTESIAN_POINT('Ctrl Pts',(-2.9668066359424,5.34508034995061,10.7138943536281));
#7216=CARTESIAN_POINT('Ctrl Pts',(-3.1150143694511,5.26281709879562,10.7216176088714));
#7217=CARTESIAN_POINT('Ctrl Pts',(-3.25981595253619,5.17437614370629,10.7293408641148));
#7218=CARTESIAN_POINT('Ctrl Pts',(-3.40070033937066,5.08006523228829,10.7370641193581));
#7219=CARTESIAN_POINT('Ctrl Pts',(-3.54159017071021,4.98575067620641,10.7447876730681));
#7220=CARTESIAN_POINT('Ctrl Pts',(-3.67856223731683,4.88556588286836,10.7525112267782));
#7221=CARTESIAN_POINT('Ctrl Pts',(-3.81113408852214,4.7798621864866,10.7602347804882));
#7222=CARTESIAN_POINT('Ctrl Pts',(-3.94369703560019,4.67416558964487,10.7679578154493));
#7223=CARTESIAN_POINT('Ctrl Pts',(-4.07186011087741,4.56295102914326,10.7756808504105));
#7224=CARTESIAN_POINT('Ctrl Pts',(-4.19517346114997,4.44661052863447,10.7834038853716));
#7225=CARTESIAN_POINT('Ctrl Pts',(-4.31851958273881,4.33023910988911,10.7911289727789));
#7226=CARTESIAN_POINT('Ctrl Pts',(-4.43701317171454,4.20873924508374,10.7988540601863));
#7227=CARTESIAN_POINT('Ctrl Pts',(-4.5502401180904,4.08254092817459,10.8065791475937));
#7228=CARTESIAN_POINT('Ctrl Pts',(-4.66302800836339,3.95683196599049,10.8142742797043));
#7229=CARTESIAN_POINT('Ctrl Pts',(-4.77058984348464,3.82646117886875,10.821969411815));
#7230=CARTESIAN_POINT('Ctrl Pts',(-4.8725551399554,3.69188731824174,10.8296645439257));
#7231=CARTESIAN_POINT('Ctrl Pts',(-4.97491305229397,3.55679528295234,10.8373893060289));
#7232=CARTESIAN_POINT('Ctrl Pts',(-5.0716674698435,3.41741987844759,10.8451140681321));
#7233=CARTESIAN_POINT('Ctrl Pts',(-5.16247311774284,3.2742475274607,10.8528388302353));
#7234=CARTESIAN_POINT('Ctrl Pts',(-5.25326105229573,3.13110310492886,10.8605620854786));
#7235=CARTESIAN_POINT('Ctrl Pts',(-5.33810236300809,2.98416348128143,10.8682853407219));
#7236=CARTESIAN_POINT('Ctrl Pts',(-5.41669552265323,2.83394339699445,10.8760085959652));
#7237=CARTESIAN_POINT('Ctrl Pts',(-5.49529171954659,2.68371750742258,10.8837321496752));
#7238=CARTESIAN_POINT('Ctrl Pts',(-5.56763913176966,2.53021118249997,10.8914557033853));
#7239=CARTESIAN_POINT('Ctrl Pts',(-5.63348219535846,2.3739637564797,10.8991792570953));
#7240=CARTESIAN_POINT('Ctrl Pts',(-5.69932083662819,2.21772682474591,10.9069022920564));
#7241=CARTESIAN_POINT('Ctrl Pts',(-5.75865588041691,2.05874945242341,10.9146253270175));
#7242=CARTESIAN_POINT('Ctrl Pts',(-5.81127985446346,1.89759110864463,10.9223483619787));
#7243=CARTESIAN_POINT('Ctrl Pts',(-5.86391781366978,1.73638993599882,10.930073449386));
#7244=CARTESIAN_POINT('Ctrl Pts',(-5.90984103873066,1.57300693450831,10.9377985367934));
#7245=CARTESIAN_POINT('Ctrl Pts',(-5.9488916105406,1.40801781541984,10.9455236242007));
#7246=CARTESIAN_POINT('Ctrl Pts',(-5.9877907573374,1.24366846876924,10.9532187563114));
#7247=CARTESIAN_POINT('Ctrl Pts',(-6.01987041528838,1.07772574956919,10.9609138884221));
#7248=CARTESIAN_POINT('Ctrl Pts',(-6.04502473326368,0.910769749569233,10.9686090205329));
#7249=CARTESIAN_POINT('Ctrl Pts',(-6.07131356640451,0.73628366609961,10.9766512200572));
#7250=CARTESIAN_POINT('Ctrl Pts',(-6.09004507716572,0.560647910903114,10.9846934195815));
#7251=CARTESIAN_POINT('Ctrl Pts',(-6.10114591531853,0.3845049837025,10.9927356191058));
#7252=CARTESIAN_POINT('Ctrl Pts',(-6.10920854597905,0.256570917289429,10.9985767352062));
#7253=CARTESIAN_POINT('Ctrl Pts',(-6.11324688458893,0.128369490857254,11.0044178513067));
#7254=CARTESIAN_POINT('Ctrl Pts',(-6.1132499981976,0.000148448865220258,
11.0102589674072));
#7255=CARTESIAN_POINT('Ctrl Pts',(-6.11324999819761,0.000148448155509828,
11.0102589674395));
#7256=CARTESIAN_POINT('Ctrl Pts',(-6.11325432008344,-0.177831321518247,
11.0183668449145));
#7257=CARTESIAN_POINT('Ctrl Pts',(-6.1054808407098,-0.355826038601997,11.0264747223896));
#7258=CARTESIAN_POINT('Ctrl Pts',(-6.08995748975051,-0.533144760390352,
11.0345825998646));
#7259=CARTESIAN_POINT('Ctrl Pts',(-6.07519299148024,-0.701795328685575,
11.0422941270516));
#7260=CARTESIAN_POINT('Ctrl Pts',(-6.05341828534077,-0.869834073479806,
11.0500056542386));
#7261=CARTESIAN_POINT('Ctrl Pts',(-6.02471068005017,-1.03667101058602,11.0577171814256));
#7262=CARTESIAN_POINT('Ctrl Pts',(-5.99600293607759,-1.20350875365554,11.0654287458658));
#7263=CARTESIAN_POINT('Ctrl Pts',(-5.96036228338477,-1.36914436384791,11.073140310306));
#7264=CARTESIAN_POINT('Ctrl Pts',(-5.91791733732643,-1.5329970486179,11.0808518747462));
#7265=CARTESIAN_POINT('Ctrl Pts',(-5.87546318887851,-1.69688525790565,11.0885651111127));
#7266=CARTESIAN_POINT('Ctrl Pts',(-5.82620188186118,-1.85898946144971,11.0962783474791));
#7267=CARTESIAN_POINT('Ctrl Pts',(-5.77031237251077,-2.01874235259212,11.1039915838456));
#7268=CARTESIAN_POINT('Ctrl Pts',(-5.76170925716808,-2.04333323851688,11.1051788882771));
#7269=CARTESIAN_POINT('Ctrl Pts',(-5.75294918397543,-2.06786844275859,11.1063661927086));
#7270=CARTESIAN_POINT('Ctrl Pts',(-5.74403290914135,-2.09234593248851,11.1075534971401));
#7271=CARTESIAN_POINT('Ctrl Pts',(-5.68602242748835,-2.25159976834616,11.1152782592433));
#7272=CARTESIAN_POINT('Ctrl Pts',(-5.62137460129056,-2.40846779971063,11.1230030213465));
#7273=CARTESIAN_POINT('Ctrl Pts',(-5.55031093176515,-2.56239616828239,11.1307277834497));
#7274=CARTESIAN_POINT('Ctrl Pts',(-5.47926112454274,-2.71629451023577,11.138451038693));
#7275=CARTESIAN_POINT('Ctrl Pts',(-5.40179810400514,-2.86725404603998,11.1461742939363));
#7276=CARTESIAN_POINT('Ctrl Pts',(-5.31819088558314,-3.0147423218246,11.1538975491796));
#7277=CARTESIAN_POINT('Ctrl Pts',(-5.23458043614362,-3.16223629732286,11.1616211028896));
#7278=CARTESIAN_POINT('Ctrl Pts',(-5.14482546652191,-3.30625846670951,11.1693446565997));
#7279=CARTESIAN_POINT('Ctrl Pts',(-5.04924057866619,-3.44630166138292,11.1770682103097));
#7280=CARTESIAN_POINT('Ctrl Pts',(-4.95366211072529,-3.58633545011988,11.1847912452708));
#7281=CARTESIAN_POINT('Ctrl Pts',(-4.85225468682151,-3.72239053715926,11.192514280232));
#7282=CARTESIAN_POINT('Ctrl Pts',(-4.74537590292885,-3.85398924523697,11.2002373151931));
#7283=CARTESIAN_POINT('Ctrl Pts',(-4.63846871531182,-3.98562292651792,11.2079624026004));
#7284=CARTESIAN_POINT('Ctrl Pts',(-4.52608746041239,-4.1127976147355,11.2156874900078));
#7285=CARTESIAN_POINT('Ctrl Pts',(-4.40863024977982,-4.23506846263744,11.2234125774151));
#7286=CARTESIAN_POINT('Ctrl Pts',(-4.29162849879485,-4.35686518522179,11.2311077095258));
#7287=CARTESIAN_POINT('Ctrl Pts',(-4.16959032732782,-4.47379582797459,11.2388028416365));
#7288=CARTESIAN_POINT('Ctrl Pts',(-4.04294575943689,-4.58545691820906,11.2464979737472));
#7289=CARTESIAN_POINT('Ctrl Pts',(-3.91581354850853,-4.69754795782161,11.2542227358504));
#7290=CARTESIAN_POINT('Ctrl Pts',(-3.78399435071139,-4.80436846048071,11.2619474979536));
#7291=CARTESIAN_POINT('Ctrl Pts',(-3.64794765405522,-4.90553804141534,11.2696722600568));
#7292=CARTESIAN_POINT('Ctrl Pts',(-3.51192749586135,-5.00668788732386,11.2773955153001));
#7293=CARTESIAN_POINT('Ctrl Pts',(-3.3716817384477,-5.1021888220238,11.2851187705434));
#7294=CARTESIAN_POINT('Ctrl Pts',(-3.22770135279048,-5.19170198872147,11.2928420257868));
#7295=CARTESIAN_POINT('Ctrl Pts',(-3.08371540298281,-5.28121861467317,11.3005655794968));
#7296=CARTESIAN_POINT('Ctrl Pts',(-2.93599480317987,-5.36474683888825,11.3082891332069));
#7297=CARTESIAN_POINT('Ctrl Pts',(-2.78505845785681,-5.4419918181508,11.3160126869169));
#7298=CARTESIAN_POINT('Ctrl Pts',(-2.63413225010372,-5.51923160928996,11.323735721878));
#7299=CARTESIAN_POINT('Ctrl Pts',(-2.47999101120721,-5.59018885559742,11.3314587568391));
#7300=CARTESIAN_POINT('Ctrl Pts',(-2.32317729030046,-5.65461518056996,11.3391817918003));
#7301=CARTESIAN_POINT('Ctrl Pts',(-2.16632189513849,-5.71905862725286,11.3469068792076));
#7302=CARTESIAN_POINT('Ctrl Pts',(-2.00679289128386,-5.77696756184149,11.354631966615));
#7303=CARTESIAN_POINT('Ctrl Pts',(-1.84515269881625,-5.8281418205592,11.3623570540223));
#7304=CARTESIAN_POINT('Ctrl Pts',(-1.68413929277372,-5.87911764267406,11.370052186133));
#7305=CARTESIAN_POINT('Ctrl Pts',(-1.52103134933433,-5.92341086220521,11.3777473182437));
#7306=CARTESIAN_POINT('Ctrl Pts',(-1.3563995169827,-5.96087291533959,11.3854424503544));
#7307=CARTESIAN_POINT('Ctrl Pts',(-1.19113377219271,-5.99847921555614,11.3931672124576));
#7308=CARTESIAN_POINT('Ctrl Pts',(-1.02427384089955,-6.02921492809192,11.4008919745608));
#7309=CARTESIAN_POINT('Ctrl Pts',(-0.856405198718806,-6.05296585965156,
11.408616736664));
#7310=CARTESIAN_POINT('Ctrl Pts',(-0.688569302468551,-6.07671215814607,
11.4163399919073));
#7311=CARTESIAN_POINT('Ctrl Pts',(-0.519725401563922,-6.09347634999393,
11.4240632471506));
#7312=CARTESIAN_POINT('Ctrl Pts',(-0.350466749436321,-6.10319577107269,
11.4317865023939));
#7313=CARTESIAN_POINT('Ctrl Pts',(-0.181201556274503,-6.1129155677604,11.439510056104));
#7314=CARTESIAN_POINT('Ctrl Pts',(-0.011521895986023,-6.11559002677367,
11.447233609814));
#7315=CARTESIAN_POINT('Ctrl Pts',(0.15797550624594,-6.11120849766446,11.454957163524));
#7316=CARTESIAN_POINT('Ctrl Pts',(0.327461524263035,-6.10682726283863,11.4626801984852));
#7317=CARTESIAN_POINT('Ctrl Pts',(0.496764991869067,-6.09539099646342,11.4704032334463));
#7318=CARTESIAN_POINT('Ctrl Pts',(0.665290651923686,-6.07694116402018,11.4781262684074));
#7319=CARTESIAN_POINT('Ctrl Pts',(0.833861098756827,-6.05848642841525,11.4858513558147));
#7320=CARTESIAN_POINT('Ctrl Pts',(1.00165300948352,-6.03301443456494,11.4935764432221));
#7321=CARTESIAN_POINT('Ctrl Pts',(1.16807674414498,-6.00061849164631,11.5013015306295));
#7322=CARTESIAN_POINT('Ctrl Pts',(1.3338551434107,-5.96834816932313,11.5089966627402));
#7323=CARTESIAN_POINT('Ctrl Pts',(1.49827565812717,-5.92920759127325,11.5166917948509));
#7324=CARTESIAN_POINT('Ctrl Pts',(1.66076610969009,-5.88333931465837,11.5243869269616));
#7325=CARTESIAN_POINT('Ctrl Pts',(1.82388062639612,-5.83729487512232,11.532111613201));
#7326=CARTESIAN_POINT('Ctrl Pts',(1.98510798689638,-5.78445462130408,11.5398362994405));
#7327=CARTESIAN_POINT('Ctrl Pts',(2.1438794530364,-5.72499838020486,11.5475609856799));
#7328=CARTESIAN_POINT('Ctrl Pts',(2.30263024492791,-5.66554988113345,11.555284666058));
#7329=CARTESIAN_POINT('Ctrl Pts',(2.45892548300991,-5.59948722248188,11.5630083464361));
#7330=CARTESIAN_POINT('Ctrl Pts',(2.61221414498486,-5.52703924567585,11.5707320268142));
#7331=CARTESIAN_POINT('Ctrl Pts',(2.76548164713755,-5.45460126952017,11.5784546410227));
#7332=CARTESIAN_POINT('Ctrl Pts',(2.91574311557921,-5.37577987086759,11.5861772552312));
#7333=CARTESIAN_POINT('Ctrl Pts',(3.06246964751821,-5.29085108659559,11.5938998694397));
#7334=CARTESIAN_POINT('Ctrl Pts',(3.20920613520849,-5.20591653969945,11.6016230076464));
#7335=CARTESIAN_POINT('Ctrl Pts',(3.35240693209947,-5.11487393661046,11.609346145853));
#7336=CARTESIAN_POINT('Ctrl Pts',(3.49156914352686,-5.01804448749422,11.6170692840597));
#7337=CARTESIAN_POINT('Ctrl Pts',(3.56999849375895,-4.96347313008603,11.6214219075563));
#7338=CARTESIAN_POINT('Ctrl Pts',(3.6471455837845,-4.90706452856059,11.6257745310529));
#7339=CARTESIAN_POINT('Ctrl Pts',(3.72292453512038,-4.84888218750453,11.6301271545495));
#7340=CARTESIAN_POINT('',(-6.11324999809968,0.000152427850000879,10.8647410325957));
#7341=CARTESIAN_POINT('Ctrl Pts',(-6.11324999809968,0.000152427850000879,
10.8647410325958));
#7342=CARTESIAN_POINT('Ctrl Pts',(-6.11325420804908,-0.168691212844257,
10.8724343082978));
#7343=CARTESIAN_POINT('Ctrl Pts',(-6.10625906233778,-0.337560295901734,
10.8801275839998));
#7344=CARTESIAN_POINT('Ctrl Pts',(-6.09228430785177,-0.505863098874644,
10.8878208597019));
#7345=CARTESIAN_POINT('Ctrl Pts',(-6.07830951280065,-0.674166390387332,
10.8955141577355));
#7346=CARTESIAN_POINT('Ctrl Pts',(-6.05735509004427,-0.84190307733042,10.9032074557691));
#7347=CARTESIAN_POINT('Ctrl Pts',(-6.02949277637401,-1.00848521166826,10.9109007538028));
#7348=CARTESIAN_POINT('Ctrl Pts',(-6.00163240587938,-1.17505572822209,10.9185935152898));
#7349=CARTESIAN_POINT('Ctrl Pts',(-5.96686516142572,-1.340471535738,10.9262862767769));
#7350=CARTESIAN_POINT('Ctrl Pts',(-5.92531418314416,-1.50415338098566,10.933979038264));
#7351=CARTESIAN_POINT('Ctrl Pts',(-5.88375244490362,-1.66787761295956,10.9416737918533));
#7352=CARTESIAN_POINT('Ctrl Pts',(-5.83540354042846,-1.82986667285239,10.9493685454426));
#7353=CARTESIAN_POINT('Ctrl Pts',(-5.78044114402197,-1.98955415683966,10.957063299032));
#7354=CARTESIAN_POINT('Ctrl Pts',(-5.73389279409895,-2.12479551036418,10.9635800833439));
#7355=CARTESIAN_POINT('Ctrl Pts',(-5.68260173604348,-2.25838616153482,10.9700968676558));
#7356=CARTESIAN_POINT('Ctrl Pts',(-5.62670098309795,-2.38999196846026,10.9766136519677));
#7357=CARTESIAN_POINT('Ctrl Pts',(-5.5604382379733,-2.54599276597585,10.9843384140709));
#7358=CARTESIAN_POINT('Ctrl Pts',(-5.48767205651953,-2.69926377932432,10.9920631761741));
#7359=CARTESIAN_POINT('Ctrl Pts',(-5.40865261290302,-2.84926349701766,10.9997879382773));
#7360=CARTESIAN_POINT('Ctrl Pts',(-5.32964858351237,-2.99923395445022,11.0075111935207));
#7361=CARTESIAN_POINT('Ctrl Pts',(-5.24439387355246,-3.14593410929278,11.015234448764));
#7362=CARTESIAN_POINT('Ctrl Pts',(-5.15318498651466,-3.288846310982,11.0229577040073));
#7363=CARTESIAN_POINT('Ctrl Pts',(-5.06197257469154,-3.43176403554126,11.0306812577174));
#7364=CARTESIAN_POINT('Ctrl Pts',(-4.96480569250414,-3.57089324474132,11.0384048114274));
#7365=CARTESIAN_POINT('Ctrl Pts',(-4.86202504467805,-3.70574392361687,11.0461283651375));
#7366=CARTESIAN_POINT('Ctrl Pts',(-4.75925130006677,-3.84058554530878,11.0538514000986));
#7367=CARTESIAN_POINT('Ctrl Pts',(-4.6508647364867,-3.97114895966124,11.0615744350597));
#7368=CARTESIAN_POINT('Ctrl Pts',(-4.53724745090694,-4.09697585198381,11.0692974700209));
#7369=CARTESIAN_POINT('Ctrl Pts',(-4.42359997080255,-4.22283618361256,11.0770225574282));
#7370=CARTESIAN_POINT('Ctrl Pts',(-4.30471920187486,-4.34395724105177,11.0847476448356));
#7371=CARTESIAN_POINT('Ctrl Pts',(-4.18102598361013,-4.45991561432242,11.0924727322429));
#7372=CARTESIAN_POINT('Ctrl Pts',(-4.05781240613828,-4.57542433993351,11.1001678643536));
#7373=CARTESIAN_POINT('Ctrl Pts',(-3.92982388491662,-4.6858101585198,11.1078629964643));
#7374=CARTESIAN_POINT('Ctrl Pts',(-3.79751096363715,-4.79069264757777,11.115558128575));
#7375=CARTESIAN_POINT('Ctrl Pts',(-3.66468857340899,-4.89597898511039,11.1232828906782));
#7376=CARTESIAN_POINT('Ctrl Pts',(-3.52746135454797,-4.9957567937649,11.1310076527814));
#7377=CARTESIAN_POINT('Ctrl Pts',(-3.38630806645332,-5.08967024880524,11.1387324148845));
#7378=CARTESIAN_POINT('Ctrl Pts',(-3.24518231295707,-5.18356538426334,11.1464556701279));
#7379=CARTESIAN_POINT('Ctrl Pts',(-3.10013228208042,-5.2715982732535,11.1541789253712));
#7380=CARTESIAN_POINT('Ctrl Pts',(-2.95166600044813,-5.3534562092445,11.1619021806146));
#7381=CARTESIAN_POINT('Ctrl Pts',(-2.80319398130754,-5.43531730865135,11.1696257343246));
#7382=CARTESIAN_POINT('Ctrl Pts',(-2.6513057228446,-5.51100282105464,11.1773492880347));
#7383=CARTESIAN_POINT('Ctrl Pts',(-2.49653484426342,-5.5802454546264,11.1850728417447));
#7384=CARTESIAN_POINT('Ctrl Pts',(-2.3417743607967,-5.64948343754871,11.1927958767058));
#7385=CARTESIAN_POINT('Ctrl Pts',(-2.18413193398178,-5.71227927817567,11.200518911667));
#7386=CARTESIAN_POINT('Ctrl Pts',(-2.02416236429372,-5.76841332477804,11.2082419466281));
#7387=CARTESIAN_POINT('Ctrl Pts',(-1.86415028166353,-5.82456228936437,11.2159670340355));
#7388=CARTESIAN_POINT('Ctrl Pts',(-1.70181011887905,-5.87404581513944,11.2236921214428));
#7389=CARTESIAN_POINT('Ctrl Pts',(-1.53771399779626,-5.91669343666557,11.2314172088502));
#7390=CARTESIAN_POINT('Ctrl Pts',(-1.37425418640611,-5.95917568502648,11.2391123409608));
#7391=CARTESIAN_POINT('Ctrl Pts',(-1.20905232080402,-5.99487490225665,11.2468074730715));
#7392=CARTESIAN_POINT('Ctrl Pts',(-1.04268604041893,-6.02367258270364,11.2545026051821));
#7393=CARTESIAN_POINT('Ctrl Pts',(-0.875679169128143,-6.05258114819389,
11.2622273672853));
#7394=CARTESIAN_POINT('Ctrl Pts',(-0.707439744144012,-6.07454513183358,
11.2699521293885));
#7395=CARTESIAN_POINT('Ctrl Pts',(-0.538558413553295,-6.08948112713152,
11.2776768914917));
#7396=CARTESIAN_POINT('Ctrl Pts',(-0.369710026436769,-6.10441420888316,
11.285400146735));
#7397=CARTESIAN_POINT('Ctrl Pts',(-0.200220299066371,-6.11232200990819,
11.2931234019784));
#7398=CARTESIAN_POINT('Ctrl Pts',(-0.0306849508333739,-6.11317298923336,
11.3008466572217));
#7399=CARTESIAN_POINT('Ctrl Pts',(0.138856949126425,-6.1140240014448,11.3085702109317));
#7400=CARTESIAN_POINT('Ctrl Pts',(0.308444156582704,-6.10781764069055,11.3162937646418));
#7401=CARTESIAN_POINT('Ctrl Pts',(0.477480206354419,-6.09457449007227,11.3240173183518));
#7402=CARTESIAN_POINT('Ctrl Pts',(0.646504902897834,-6.0813322289241,11.3317403533129));
#7403=CARTESIAN_POINT('Ctrl Pts',(0.814978199847684,-6.06105414847014,11.3394633882741));
#7404=CARTESIAN_POINT('Ctrl Pts',(0.98230782461247,-6.03381279956589,11.3471864232352));
#7405=CARTESIAN_POINT('Ctrl Pts',(1.14968191830179,-6.00656421109787,11.3549115106425));
#7406=CARTESIAN_POINT('Ctrl Pts',(1.31591141908453,-5.97234870517448,11.3626365980499));
#7407=CARTESIAN_POINT('Ctrl Pts',(1.48041237617283,-5.93129031147307,11.3703616854573));
#7408=CARTESIAN_POINT('Ctrl Pts',(1.64427545375064,-5.8903911284446,11.3780568175679));
#7409=CARTESIAN_POINT('Ctrl Pts',(1.80642307413885,-5.84270213902499,11.3857519496786));
#7410=CARTESIAN_POINT('Ctrl Pts',(1.96629130050559,-5.78839563990369,11.3934470817893));
#7411=CARTESIAN_POINT('Ctrl Pts',(2.12678130988935,-5.73387792395942,11.4011721429395));
#7412=CARTESIAN_POINT('Ctrl Pts',(2.28503099222204,-5.67267178152857,11.4088972040896));
#7413=CARTESIAN_POINT('Ctrl Pts',(2.44048171537531,-5.60498657977152,11.4166222652398));
#7414=CARTESIAN_POINT('Ctrl Pts',(2.59589888624497,-5.53731598710112,11.4243456590227));
#7415=CARTESIAN_POINT('Ctrl Pts',(2.74851801325822,-5.4631692526716,11.4320690528057));
#7416=CARTESIAN_POINT('Ctrl Pts',(2.89780086164218,-5.38280370520474,11.4397924465886));
#7417=CARTESIAN_POINT('Ctrl Pts',(3.04708476294043,-5.30243759090763,11.4475158948458));
#7418=CARTESIAN_POINT('Ctrl Pts',(3.19303205762039,-5.21585272257969,11.455239343103));
#7419=CARTESIAN_POINT('Ctrl Pts',(3.33512884395811,-5.12335253097995,11.4629627913602));
#7420=CARTESIAN_POINT('Ctrl Pts',(3.46788730481097,-5.03693127275254,11.4701786695621));
#7421=CARTESIAN_POINT('Ctrl Pts',(3.59728477563354,-4.94534717161686,11.477394547764));
#7422=CARTESIAN_POINT('Ctrl Pts',(3.72292453512039,-4.84888218750453,11.484610425966));
#7423=CARTESIAN_POINT('Ctrl Pts',(3.72292453512039,-4.84888218750452,9.73461637809168));
#7424=CARTESIAN_POINT('Ctrl Pts',(3.85736574640416,-4.74565953439295,9.74234051282505));
#7425=CARTESIAN_POINT('Ctrl Pts',(3.98753222395988,-4.63682608808731,9.75006464755842));
#7426=CARTESIAN_POINT('Ctrl Pts',(4.112962928074,-4.52276038662109,9.75778878229179));
#7427=CARTESIAN_POINT('Ctrl Pts',(4.23837298429734,-4.40871346218528,9.76551164550961));
#7428=CARTESIAN_POINT('Ctrl Pts',(4.35904858845556,-4.28943621450911,9.77323450872743));
#7429=CARTESIAN_POINT('Ctrl Pts',(4.47456347729856,-4.16534599404729,9.78095737194525));
#7430=CARTESIAN_POINT('Ctrl Pts',(4.59008473161228,-4.04124893556941,9.78868066073298));
#7431=CARTESIAN_POINT('Ctrl Pts',(4.70044448374109,-3.91233860380513,9.7964039495207));
#7432=CARTESIAN_POINT('Ctrl Pts',(4.80525437749419,-3.7790681298533,9.80412723830842));
#7433=CARTESIAN_POINT('Ctrl Pts',(4.910060430352,-3.64580253977185,9.81185024406615));
#7434=CARTESIAN_POINT('Ctrl Pts',(5.00931683705915,-3.50817737726526,9.81957324982388));
#7435=CARTESIAN_POINT('Ctrl Pts',(5.1026763534931,-3.36667782747361,9.82729625558161));
#7436=CARTESIAN_POINT('Ctrl Pts',(5.19605783455074,-3.22514498718856,9.83502107832513));
#7437=CARTESIAN_POINT('Ctrl Pts',(5.28353947846812,-3.07973620280037,9.84274590106866));
#7438=CARTESIAN_POINT('Ctrl Pts',(5.36481763811116,-2.93096524583821,9.85047072381218));
#7439=CARTESIAN_POINT('Ctrl Pts',(5.41597798725634,-2.83732171190149,9.85533309557822));
#7440=CARTESIAN_POINT('Ctrl Pts',(5.46468137364533,-2.74234662089777,9.86019546734425));
#7441=CARTESIAN_POINT('Ctrl Pts',(5.51086141100289,-2.64617309925469,9.86505783911028));
#7442=CARTESIAN_POINT('Ctrl Pts',(5.58422680132456,-2.49338396443177,9.87278260121348));
#7443=CARTESIAN_POINT('Ctrl Pts',(5.65124712872478,-2.33751480002962,9.88050736331668));
#7444=CARTESIAN_POINT('Ctrl Pts',(5.71168104348704,-2.17911110776178,9.88823212541987));
#7445=CARTESIAN_POINT('Ctrl Pts',(5.77210316947964,-2.020738315108,9.8959553806632));
#7446=CARTESIAN_POINT('Ctrl Pts',(5.82594133357522,-1.85983227703631,9.90367863590652));
#7447=CARTESIAN_POINT('Ctrl Pts',(5.87300270167234,-1.69695752116821,9.91140189114985));
#7448=CARTESIAN_POINT('Ctrl Pts',(5.92006588846532,-1.53407647097304,9.9191254448599));
#7449=CARTESIAN_POINT('Ctrl Pts',(5.96035166342292,-1.3692268541014,9.92684899856995));
#7450=CARTESIAN_POINT('Ctrl Pts',(5.99371713664409,-1.20298813310812,9.93457255227999));
#7451=CARTESIAN_POINT('Ctrl Pts',(6.02708036888863,-1.03676057746192,9.94229558724112));
#7452=CARTESIAN_POINT('Ctrl Pts',(6.05352416716979,-0.869144415160902,9.95001862220223));
#7453=CARTESIAN_POINT('Ctrl Pts',(6.07295678239129,-0.700729249930136,9.95774165716336));
#7454=CARTESIAN_POINT('Ctrl Pts',(6.09239456195533,-0.532269327285528,9.96546674457071));
#7455=CARTESIAN_POINT('Ctrl Pts',(6.10481739668134,-0.363010292213752,9.97319183197807));
#7456=CARTESIAN_POINT('Ctrl Pts',(6.11018533417448,-0.193547783606798,9.98091691938543));
#7457=CARTESIAN_POINT('Ctrl Pts',(6.11553245660733,-0.0247423937419612,
9.98861205149611));
#7458=CARTESIAN_POINT('Ctrl Pts',(6.11387931993266,0.144264581405888,9.9963071836068));
#7459=CARTESIAN_POINT('Ctrl Pts',(6.10523786759826,0.312883592641504,10.0040023157175));
#7460=CARTESIAN_POINT('Ctrl Pts',(6.0965631414793,0.48215186888887,10.0117270778207));
#7461=CARTESIAN_POINT('Ctrl Pts',(6.08084307374087,0.65108913584488,10.0194518399239));
#7462=CARTESIAN_POINT('Ctrl Pts',(6.05812671286995,0.819100905451548,10.0271766020271));
#7463=CARTESIAN_POINT('Ctrl Pts',(6.03541478325168,0.987079901208335,10.0348998572704));
#7464=CARTESIAN_POINT('Ctrl Pts',(6.00570932612104,1.15413344597106,10.0426231125137));
#7465=CARTESIAN_POINT('Ctrl Pts',(5.9691110953439,1.31967355582444,10.050346367757));
#7466=CARTESIAN_POINT('Ctrl Pts',(5.93251145022092,1.48522006300799,10.0580699214671));
#7467=CARTESIAN_POINT('Ctrl Pts',(5.88901856296916,1.64925270794545,10.0657934751771));
#7468=CARTESIAN_POINT('Ctrl Pts',(5.83878419006957,1.81119428673283,10.0735170288872));
#7469=CARTESIAN_POINT('Ctrl Pts',(5.78855319113848,1.97312498878872,10.0812400638483));
#7470=CARTESIAN_POINT('Ctrl Pts',(5.73158170657638,2.13296460302393,10.0889630988094));
#7471=CARTESIAN_POINT('Ctrl Pts',(5.66807125277237,2.29015148756484,10.0966861337705));
#7472=CARTESIAN_POINT('Ctrl Pts',(5.60454392065661,2.44738014553172,10.1044112211779));
#7473=CARTESIAN_POINT('Ctrl Pts',(5.53447426359638,2.60195437021206,10.1121363085853));
#7474=CARTESIAN_POINT('Ctrl Pts',(5.45811216941679,2.75333200115139,10.1198613959926));
#7475=CARTESIAN_POINT('Ctrl Pts',(5.3820461818139,2.90412264043515,10.1275565281033));
#7476=CARTESIAN_POINT('Ctrl Pts',(5.29973663965096,3.05174116833154,10.135251660214));
#7477=CARTESIAN_POINT('Ctrl Pts',(5.21147608835822,3.19567560039665,10.1429467923246));
#7478=CARTESIAN_POINT('Ctrl Pts',(5.12287569111643,3.34016424986636,10.1506715544278));
#7479=CARTESIAN_POINT('Ctrl Pts',(5.02824696000459,3.48099153395726,10.158396316531));
#7480=CARTESIAN_POINT('Ctrl Pts',(4.92791738625288,3.61765888341708,10.1661210786342));
#7481=CARTESIAN_POINT('Ctrl Pts',(4.82760738366812,3.7542995733446,10.1738443338775));
#7482=CARTESIAN_POINT('Ctrl Pts',(4.72159894482899,3.88678169250037,10.1815675891209));
#7483=CARTESIAN_POINT('Ctrl Pts',(4.61026185303658,4.01463712045506,10.1892908443642));
#7484=CARTESIAN_POINT('Ctrl Pts',(4.49892045860029,4.14249748940799,10.1970143980743));
#7485=CARTESIAN_POINT('Ctrl Pts',(4.38225020427461,4.26573056776866,10.2047379517843));
#7486=CARTESIAN_POINT('Ctrl Pts',(4.26066050261565,4.38390210245974,10.2124615054943));
#7487=CARTESIAN_POINT('Ctrl Pts',(4.13907896747297,4.50206570021416,10.2201845404555));
#7488=CARTESIAN_POINT('Ctrl Pts',(4.01257887350575,4.61516821370677,10.2279075754166));
#7489=CARTESIAN_POINT('Ctrl Pts',(3.88160588341402,4.72281286188069,10.2356306103777));
#7490=CARTESIAN_POINT('Ctrl Pts',(3.75059808640744,4.83048611731249,10.2433556977851));
#7491=CARTESIAN_POINT('Ctrl Pts',(3.61511526159468,4.93269840599053,10.2510807851924));
#7492=CARTESIAN_POINT('Ctrl Pts',(3.47563622741577,5.02909319631035,10.2588058725998));
#7493=CARTESIAN_POINT('Ctrl Pts',(3.33669804612664,5.12511419998037,10.2665010047105));
#7494=CARTESIAN_POINT('Ctrl Pts',(3.19379486744877,5.21536259073196,10.2741961368212));
#7495=CARTESIAN_POINT('Ctrl Pts',(3.0474285314929,5.29952874394913,10.2818912689319));
#7496=CARTESIAN_POINT('Ctrl Pts',(2.9004986141226,5.38401897769593,10.2896160310351));
#7497=CARTESIAN_POINT('Ctrl Pts',(2.75002676368807,5.46240993969483,10.2973407931383));
#7498=CARTESIAN_POINT('Ctrl Pts',(2.59653908889921,5.53442050465254,10.3050655552415));
#7499=CARTESIAN_POINT('Ctrl Pts',(2.44308135476278,5.60641702259767,10.3127888104848));
#7500=CARTESIAN_POINT('Ctrl Pts',(2.28660925687176,5.67203549242728,10.3205120657281));
#7501=CARTESIAN_POINT('Ctrl Pts',(2.12767147410012,5.73104176051794,10.3282353209715));
#7502=CARTESIAN_POINT('Ctrl Pts',(1.96872754914669,5.79005030891742,10.3359588746815));
#7503=CARTESIAN_POINT('Ctrl Pts',(1.80731804436292,5.84244603023263,10.3436824283916));
#7504=CARTESIAN_POINT('Ctrl Pts',(1.64401023497448,5.88804347044068,10.3514059821016));
#7505=CARTESIAN_POINT('Ctrl Pts',(1.48071339407973,5.9336378481177,10.3591290170627));
#7506=CARTESIAN_POINT('Ctrl Pts',(1.31551880900891,5.97243477319408,10.3668520520239));
#7507=CARTESIAN_POINT('Ctrl Pts',(1.14900765947488,6.00429903993531,10.374575086985));
#7508=CARTESIAN_POINT('Ctrl Pts',(0.982452258531474,6.03617177481044,10.3823001743923));
#7509=CARTESIAN_POINT('Ctrl Pts',(0.814579905056783,6.06110810804048,10.3900252617997));
#7510=CARTESIAN_POINT('Ctrl Pts',(0.645981637169343,6.07902404066146,10.3977503492071));
#7511=CARTESIAN_POINT('Ctrl Pts',(0.478037136789328,6.09687050130768,10.4054454813177));
#7512=CARTESIAN_POINT('Ctrl Pts',(0.309372655541613,6.10775090914417,10.4131406134284));
#7513=CARTESIAN_POINT('Ctrl Pts',(0.140577005799611,6.11163346969862,10.420835745539));
#7514=CARTESIAN_POINT('Ctrl Pts',(-0.0288685890988558,6.11553097999515,
10.4285605076422));
#7515=CARTESIAN_POINT('Ctrl Pts',(-0.198506377900037,6.11237799618206,10.4362852697454));
#7516=CARTESIAN_POINT('Ctrl Pts',(-0.367739872249517,6.10217936059388,10.4440100318486));
#7517=CARTESIAN_POINT('Ctrl Pts',(-0.536940354428697,6.09198271444104,10.4517332870919));
#7518=CARTESIAN_POINT('Ctrl Pts',(-0.705736383360155,6.07474317795971,10.4594565423353));
#7519=CARTESIAN_POINT('Ctrl Pts',(-0.873534123859799,6.05051763876055,10.4671797975786));
#7520=CARTESIAN_POINT('Ctrl Pts',(-1.04133834893615,6.02629116336065,10.4749033512886));
#7521=CARTESIAN_POINT('Ctrl Pts',(-1.20814389414981,5.99507818636999,10.4826269049987));
#7522=CARTESIAN_POINT('Ctrl Pts',(-1.37336389368796,5.95698725682826,10.4903504587087));
#7523=CARTESIAN_POINT('Ctrl Pts',(-1.53857279630091,5.91889888564627,10.4980734936698));
#7524=CARTESIAN_POINT('Ctrl Pts',(-1.70219605749311,5.87393355757187,10.5057965286309));
#7525=CARTESIAN_POINT('Ctrl Pts',(-1.86365864180932,5.82225059829182,10.5135195635921));
#7526=CARTESIAN_POINT('Ctrl Pts',(-2.02516413584634,5.77055390393275,10.5212446509994));
#7527=CARTESIAN_POINT('Ctrl Pts',(-2.18450750287111,5.71213610560674,10.5289697384068));
#7528=CARTESIAN_POINT('Ctrl Pts',(-2.34112954932161,5.64720621155215,10.5366948258141));
#7529=CARTESIAN_POINT('Ctrl Pts',(-2.49714426803351,5.58252809383823,10.5443899579248));
#7530=CARTESIAN_POINT('Ctrl Pts',(-2.65045845734697,5.51138844339849,10.5520850900355));
#7531=CARTESIAN_POINT('Ctrl Pts',(-2.80053985434043,5.43404104573667,10.5597802221462));
#7532=CARTESIAN_POINT('Ctrl Pts',(-2.95119913753571,5.35639582306288,10.5675049842494));
#7533=CARTESIAN_POINT('Ctrl Pts',(-3.09865402863322,5.27246742627327,10.5752297463526));
#7534=CARTESIAN_POINT('Ctrl Pts',(-3.24238305235198,5.18254548502188,10.5829545084558));
#7535=CARTESIAN_POINT('Ctrl Pts',(-3.38608403902615,5.09264108473341,10.5906777636991));
#7536=CARTESIAN_POINT('Ctrl Pts',(-3.52606034003548,4.99674564085416,10.5984010189424));
#7537=CARTESIAN_POINT('Ctrl Pts',(-3.66181770989931,4.89519321599952,10.6061242741858));
#7538=CARTESIAN_POINT('Ctrl Pts',(-3.79758032613371,4.79363686663122,10.6138478278958));
#7539=CARTESIAN_POINT('Ctrl Pts',(-3.92912342882153,4.68642328548612,10.6215713816059));
#7540=CARTESIAN_POINT('Ctrl Pts',(-4.05598360880754,4.57392856607802,10.6292949353159));
#7541=CARTESIAN_POINT('Ctrl Pts',(-4.18283526828806,4.46144140232588,10.637017970277));
#7542=CARTESIAN_POINT('Ctrl Pts',(-4.3050043973426,4.34367402043189,10.6447410052382));
#7543=CARTESIAN_POINT('Ctrl Pts',(-4.42206226839468,4.22104144222016,10.6524640401993));
#7544=CARTESIAN_POINT('Ctrl Pts',(-4.53915124832916,4.09837627361174,10.6601891276067));
#7545=CARTESIAN_POINT('Ctrl Pts',(-4.65112603538813,3.97084355295081,10.667914215014));
#7546=CARTESIAN_POINT('Ctrl Pts',(-4.75759558276085,3.83889435038194,10.6756393024214));
#7547=CARTESIAN_POINT('Ctrl Pts',(-4.86365227695647,3.70745680254293,10.683334434532));
#7548=CARTESIAN_POINT('Ctrl Pts',(-4.96424617955939,3.5716372263821,10.6910295666427));
#7549=CARTESIAN_POINT('Ctrl Pts',(-5.05903131501063,3.43191312772364,10.6987246987534));
#7550=CARTESIAN_POINT('Ctrl Pts',(-5.15418141922566,3.29165102348744,10.7064494608566));
#7551=CARTESIAN_POINT('Ctrl Pts',(-5.24351160883361,3.14740457493227,10.7141742229598));
#7552=CARTESIAN_POINT('Ctrl Pts',(-5.32670253007409,2.99967760244368,10.721898985063));
#7553=CARTESIAN_POINT('Ctrl Pts',(-5.40987722336353,2.85197944687454,10.7296222403063));
#7554=CARTESIAN_POINT('Ctrl Pts',(-5.48691488246913,2.70080239808559,10.7373454955496));
#7555=CARTESIAN_POINT('Ctrl Pts',(-5.55754132285721,2.54667626667281,10.7450687507929));
#7556=CARTESIAN_POINT('Ctrl Pts',(-5.62817049261808,2.39254417902511,10.7527923045029));
#7557=CARTESIAN_POINT('Ctrl Pts',(-5.69238781224909,2.23546306715605,10.760515858213));
#7558=CARTESIAN_POINT('Ctrl Pts',(-5.74996628420993,2.07598489709079,10.768239411923));
#7559=CARTESIAN_POINT('Ctrl Pts',(-5.80754088893923,1.91651743830334,10.7759624468841));
#7560=CARTESIAN_POINT('Ctrl Pts',(-5.85847743067887,1.75465354162588,10.7836854818453));
#7561=CARTESIAN_POINT('Ctrl Pts',(-5.90259799113035,1.59096276436752,10.7914085168064));
#7562=CARTESIAN_POINT('Ctrl Pts',(-5.94673027690468,1.42722848523175,10.7991336042137));
#7563=CARTESIAN_POINT('Ctrl Pts',(-5.98404287714979,1.26166666101199,10.8068586916211));
#7564=CARTESIAN_POINT('Ctrl Pts',(-6.014408208602,1.09486047640825,10.8145837790284));
#7565=CARTESIAN_POINT('Ctrl Pts',(-6.04465579348868,0.928701110212442,10.8222789111392));
#7566=CARTESIAN_POINT('Ctrl Pts',(-6.06800986796465,0.76130732981663,10.8299740432499));
#7567=CARTESIAN_POINT('Ctrl Pts',(-6.08439507461123,0.593263970376244,10.8376691753606));
#7568=CARTESIAN_POINT('Ctrl Pts',(-6.10189384394049,0.413800137689429,10.8458872799392));
#7569=CARTESIAN_POINT('Ctrl Pts',(-6.11144867149434,0.23355642126168,10.8541053845179));
#7570=CARTESIAN_POINT('Ctrl Pts',(-6.11301843917963,0.053208314667885,10.8623234890965));
#7571=CARTESIAN_POINT('Ctrl Pts',(-6.11317236687149,0.0355238075657486,
10.8631293369179));
#7572=CARTESIAN_POINT('Ctrl Pts',(-6.11324955711771,0.0178382994096718,
10.8639351847392));
#7573=CARTESIAN_POINT('Ctrl Pts',(-6.11324999809966,0.000152428621332483,
10.8647410325606));
#7574=CARTESIAN_POINT('Origin',(0.,0.,-3.86474103256053));
#7575=CARTESIAN_POINT('',(3.72292453512037,-4.84888218750454,7.98461472294509));
#7576=CARTESIAN_POINT('',(3.72292453512038,-4.84888218750453,8.13013011411225));
#7577=CARTESIAN_POINT('',(3.72292453512038,-4.84888218750453,-3.86474103256053));
#7578=CARTESIAN_POINT('',(-6.11324999816031,-0.000149976428034001,9.26025896747021));
#7579=CARTESIAN_POINT('Ctrl Pts',(3.72292453512038,-4.84888218750453,8.13013011411225));
#7580=CARTESIAN_POINT('Ctrl Pts',(3.8573997599122,-4.74563341915264,8.13785312315989));
#7581=CARTESIAN_POINT('Ctrl Pts',(3.9875736773476,-4.63678976520587,8.14557613220753));
#7582=CARTESIAN_POINT('Ctrl Pts',(4.11299006133295,-4.52273571169888,8.15329914125517));
#7583=CARTESIAN_POINT('Ctrl Pts',(4.23843542662074,-4.40865530250443,8.16102393494095));
#7584=CARTESIAN_POINT('Ctrl Pts',(4.35912082733167,-4.28936230135537,8.16874872862672));
#7585=CARTESIAN_POINT('Ctrl Pts',(4.4746252444227,-4.16527964060939,8.17647352231249));
#7586=CARTESIAN_POINT('Ctrl Pts',(4.54064502664269,-4.09435672314841,8.18088884433803));
#7587=CARTESIAN_POINT('Ctrl Pts',(4.60497284510067,-4.02186970029884,8.18530416636357));
#7588=CARTESIAN_POINT('Ctrl Pts',(4.66753571967432,-3.94790271765457,8.1897194883891));
#7589=CARTESIAN_POINT('Ctrl Pts',(4.77699168229202,-3.81849486447602,8.19744425049228));
#7590=CARTESIAN_POINT('Ctrl Pts',(4.88108194442947,-3.6845092756081,8.20516901259547));
#7591=CARTESIAN_POINT('Ctrl Pts',(4.97943563993126,-3.54641315560982,8.21289377469864));
#7592=CARTESIAN_POINT('Ctrl Pts',(5.07777014969844,-3.4083439738521,8.22061702994196));
#7593=CARTESIAN_POINT('Ctrl Pts',(5.17037014194221,-3.26616611890436,8.22834028518528));
#7594=CARTESIAN_POINT('Ctrl Pts',(5.25690691641525,-3.12037741862191,8.2360635404286));
#7595=CARTESIAN_POINT('Ctrl Pts',(5.34344703511902,-2.97458308430636,8.24378709413865));
#7596=CARTESIAN_POINT('Ctrl Pts',(5.42392330200462,-2.82517789592657,8.2515106478487));
#7597=CARTESIAN_POINT('Ctrl Pts',(5.49805159489902,-2.67268670485868,8.25923420155874));
#7598=CARTESIAN_POINT('Ctrl Pts',(5.57217490900077,-2.52020575579142,8.26695723651986));
#7599=CARTESIAN_POINT('Ctrl Pts',(5.63995096375848,-2.36463950388084,8.27468027148098));
#7600=CARTESIAN_POINT('Ctrl Pts',(5.70114257959357,-2.20653548569816,8.28240330644209));
#7601=CARTESIAN_POINT('Ctrl Pts',(5.7623504574944,-2.04838945035507,8.29012839384946));
#7602=CARTESIAN_POINT('Ctrl Pts',(5.81697028332761,-1.88770459605305,8.29785348125682));
#7603=CARTESIAN_POINT('Ctrl Pts',(5.86481348823859,-1.72504733577798,8.30557856866419));
#7604=CARTESIAN_POINT('Ctrl Pts',(5.91247117325567,-1.56302080577533,8.31327370077489));
#7605=CARTESIAN_POINT('Ctrl Pts',(5.953404641684,-1.39903744786339,8.3209688328856));
#7606=CARTESIAN_POINT('Ctrl Pts',(5.98747708276542,-1.23367084178031,8.32866396499631));
#7607=CARTESIAN_POINT('Ctrl Pts',(6.02168071927778,-1.06766749402391,8.33638872709951));
#7608=CARTESIAN_POINT('Ctrl Pts',(6.04898247149159,-0.900211425091387,8.34411348920271));
#7609=CARTESIAN_POINT('Ctrl Pts',(6.0692801964792,-0.731890332717556,8.35183825130591));
#7610=CARTESIAN_POINT('Ctrl Pts',(6.08957396201447,-0.56360207453292,8.35956150654923));
#7611=CARTESIAN_POINT('Ctrl Pts',(6.10286638859551,-0.394449444057672,8.36728476179255));
#7612=CARTESIAN_POINT('Ctrl Pts',(6.10910701135986,-0.225026856738937,8.37500801703588));
#7613=CARTESIAN_POINT('Ctrl Pts',(6.1153478752943,-0.0555977220509368,8.38273157074592));
#7614=CARTESIAN_POINT('Ctrl Pts',(6.11453637446197,0.11410107379936,8.39045512445596));
#7615=CARTESIAN_POINT('Ctrl Pts',(6.10667411801386,0.283472712760192,8.39817867816601));
#7616=CARTESIAN_POINT('Ctrl Pts',(6.09881238963058,0.452832975953017,8.40590171312713));
#7617=CARTESIAN_POINT('Ctrl Pts',(6.08390086800804,0.621865809612514,8.41362474808825));
#7618=CARTESIAN_POINT('Ctrl Pts',(6.06199323707562,0.789976933935036,8.42134778304937));
#7619=CARTESIAN_POINT('Ctrl Pts',(6.0400797840493,0.958132734870672,8.42907287045674));
#7620=CARTESIAN_POINT('Ctrl Pts',(6.01116654528001,1.12536602222688,8.4367979578641));
#7621=CARTESIAN_POINT('Ctrl Pts',(5.97535892207165,1.29108919711951,8.44452304527146));
#7622=CARTESIAN_POINT('Ctrl Pts',(5.93969014881027,1.45616975315099,8.45221817738213));
#7623=CARTESIAN_POINT('Ctrl Pts',(5.89718046172444,1.61975158898021,8.4599133094928));
#7624=CARTESIAN_POINT('Ctrl Pts',(5.84798414103763,1.78126557499785,8.46760844160348));
#7625=CARTESIAN_POINT('Ctrl Pts',(5.79859839064467,1.94340146823296,8.47533320370668));
#7626=CARTESIAN_POINT('Ctrl Pts',(5.74245689117747,2.10351097055519,8.48305796580988));
#7627=CARTESIAN_POINT('Ctrl Pts',(5.67975112004893,2.26102914107779,8.49078272791308));
#7628=CARTESIAN_POINT('Ctrl Pts',(5.61705758085826,2.41851658472404,8.49850598315641));
#7629=CARTESIAN_POINT('Ctrl Pts',(5.5478024421776,2.57341341092616,8.50622923839974));
#7630=CARTESIAN_POINT('Ctrl Pts',(5.472225775228,2.72517350409664,8.51395249364307));
#7631=CARTESIAN_POINT('Ctrl Pts',(5.3966461876034,2.87693946206544,8.5216760473531));
#7632=CARTESIAN_POINT('Ctrl Pts',(5.31474472058753,3.02556815898231,8.52939960106314));
#7633=CARTESIAN_POINT('Ctrl Pts',(5.2268083224284,3.17053628320087,8.53712315477317));
#7634=CARTESIAN_POINT('Ctrl Pts',(5.13887783047677,3.31549467070244,8.54484618973429));
#7635=CARTESIAN_POINT('Ctrl Pts',(5.04491338291061,3.45679270651908,8.55256922469541));
#7636=CARTESIAN_POINT('Ctrl Pts',(4.94524644182811,3.59393422200329,8.56029225965653));
#7637=CARTESIAN_POINT('Ctrl Pts',(4.84555301361461,3.73111218372783,8.5680173470639));
#7638=CARTESIAN_POINT('Ctrl Pts',(4.74015424828601,3.86413115998052,8.57574243447126));
#7639=CARTESIAN_POINT('Ctrl Pts',(4.6294238259699,3.99252559190824,8.58346752187862));
#7640=CARTESIAN_POINT('Ctrl Pts',(4.51912277907408,4.12042215331384,8.5911626539893));
#7641=CARTESIAN_POINT('Ctrl Pts',(4.40353157874229,4.24372975614234,8.59885778609998));
#7642=CARTESIAN_POINT('Ctrl Pts',(4.28305799071617,4.36202244499755,8.60655291821066));
#7643=CARTESIAN_POINT('Ctrl Pts',(4.16212052091903,4.48077061810374,8.61427768031386));
#7644=CARTESIAN_POINT('Ctrl Pts',(4.03622013617656,4.59450721651413,8.62200244241706));
#7645=CARTESIAN_POINT('Ctrl Pts',(3.90579526204611,4.70282775928251,8.62972720452026));
#7646=CARTESIAN_POINT('Ctrl Pts',(3.77539582973515,4.81112717209608,8.63745045976363));
#7647=CARTESIAN_POINT('Ctrl Pts',(3.640473912771,4.9140124350067,8.645173715007));
#7648=CARTESIAN_POINT('Ctrl Pts',(3.50150160162873,5.01111884675383,8.65289697025037));
#7649=CARTESIAN_POINT('Ctrl Pts',(3.3625239198749,5.10822901119683,8.66062052396042));
#7650=CARTESIAN_POINT('Ctrl Pts',(3.21949578823365,5.19955969282079,8.66834407767047));
#7651=CARTESIAN_POINT('Ctrl Pts',(3.07291955104879,5.28478864244182,8.67606763138052));
#7652=CARTESIAN_POINT('Ctrl Pts',(2.92635315858919,5.37001186769984,8.68379066634166));
#7653=CARTESIAN_POINT('Ctrl Pts',(2.77623941148398,5.44913402175403,8.69151370130279));
#7654=CARTESIAN_POINT('Ctrl Pts',(2.62310675684637,5.52187798712421,8.69923673626392));
#7655=CARTESIAN_POINT('Ctrl Pts',(2.46993340622074,5.59464128467113,8.70696182367127));
#7656=CARTESIAN_POINT('Ctrl Pts',(2.31373983041921,5.66102286836999,8.71468691107863));
#7657=CARTESIAN_POINT('Ctrl Pts',(2.1550769046879,5.72079269834005,8.72241199848598));
#7658=CARTESIAN_POINT('Ctrl Pts',(1.99702922054153,5.78033076096589,8.73010713059661));
#7659=CARTESIAN_POINT('Ctrl Pts',(1.83653160655494,5.83330817515008,8.73780226270723));
#7660=CARTESIAN_POINT('Ctrl Pts',(1.67414592198967,5.87954598539593,8.74549739481786));
#7661=CARTESIAN_POINT('Ctrl Pts',(1.51113497374385,5.92596183364735,8.75322215692104));
#7662=CARTESIAN_POINT('Ctrl Pts',(1.34616364423006,5.96560248367512,8.76094691902423));
#7663=CARTESIAN_POINT('Ctrl Pts',(1.17981044188946,5.99832250581015,8.76867168112741));
#7664=CARTESIAN_POINT('Ctrl Pts',(1.01348968986373,6.03103614529066,8.77639493637074));
#7665=CARTESIAN_POINT('Ctrl Pts',(0.845787913659838,6.05683178948147,8.78411819161407));
#7666=CARTESIAN_POINT('Ctrl Pts',(0.677294151997093,6.07561504657517,8.7918414468574));
#7667=CARTESIAN_POINT('Ctrl Pts',(0.508793878860008,6.0943990295515,8.79956500056744));
#7668=CARTESIAN_POINT('Ctrl Pts',(0.339501873546732,6.10617004410448,8.80728855427748));
#7669=CARTESIAN_POINT('Ctrl Pts',(0.170013431173421,6.11088545103904,8.81501210798751));
#7670=CARTESIAN_POINT('Ctrl Pts',(0.000536372413207947,6.11560054126547,
8.82273514294863));
#7671=CARTESIAN_POINT('Ctrl Pts',(-0.169136780169513,6.11326096338999,8.83045817790974));
#7672=CARTESIAN_POINT('Ctrl Pts',(-0.338409402262352,6.10387619787299,8.83818121287085));
#7673=CARTESIAN_POINT('Ctrl Pts',(-0.507727009643669,6.09448893829417,8.8459063002782));
#7674=CARTESIAN_POINT('Ctrl Pts',(-0.676643557050688,6.07805276513605,8.85363138768555));
#7675=CARTESIAN_POINT('Ctrl Pts',(-0.84456524874239,6.05462922920279,8.86135647509289));
#7676=CARTESIAN_POINT('Ctrl Pts',(-1.01183579646384,6.03129652188154,8.86905160720361));
#7677=CARTESIAN_POINT('Ctrl Pts',(-1.17811888544632,6.00103061981052,8.87674673931433));
#7678=CARTESIAN_POINT('Ctrl Pts',(-1.34283551486153,5.9639431873993,8.88444187142505));
#7679=CARTESIAN_POINT('Ctrl Pts',(-1.5081863832247,5.92671295037753,8.89216663352827));
#7680=CARTESIAN_POINT('Ctrl Pts',(-1.67201726057745,5.88259533119599,8.89989139563148));
#7681=CARTESIAN_POINT('Ctrl Pts',(-1.83375056574864,5.83173939962311,8.9076161577347));
#7682=CARTESIAN_POINT('Ctrl Pts',(-1.99545232180208,5.78089338845452,8.91533941297804));
#7683=CARTESIAN_POINT('Ctrl Pts',(-2.15505701996771,5.72331178267044,8.92306266822139));
#7684=CARTESIAN_POINT('Ctrl Pts',(-2.31200225016791,5.65919350771102,8.93078592346472));
#7685=CARTESIAN_POINT('Ctrl Pts',(-2.46895354554717,5.59507275488834,8.93850947717477));
#7686=CARTESIAN_POINT('Ctrl Pts',(-2.62324487242339,5.52441494359042,8.9462330308848));
#7687=CARTESIAN_POINT('Ctrl Pts',(-2.77433308677689,5.44746743782054,8.95395658459485));
#7688=CARTESIAN_POINT('Ctrl Pts',(-2.92541115335974,5.3705251001946,8.96167961955595));
#7689=CARTESIAN_POINT('Ctrl Pts',(-3.07328625550624,5.28729405732557,8.96940265451705));
#7690=CARTESIAN_POINT('Ctrl Pts',(-3.21743901756219,5.19806807677318,8.97712568947815));
#7691=CARTESIAN_POINT('Ctrl Pts',(-3.3616300891425,5.10881838384215,8.9848507768855));
#7692=CARTESIAN_POINT('Ctrl Pts',(-3.50209657308055,5.01357073470532,8.99257586429285));
#7693=CARTESIAN_POINT('Ctrl Pts',(-3.63834648953989,4.91266326797927,9.0003009517002));
#7694=CARTESIAN_POINT('Ctrl Pts',(-3.77406807454422,4.81214708654792,9.00799608381087));
#7695=CARTESIAN_POINT('Ctrl Pts',(-3.90560550311546,4.70601511495476,9.01569121592155));
#7696=CARTESIAN_POINT('Ctrl Pts',(-4.03250376303064,4.59464241956257,9.02338634803222));
#7697=CARTESIAN_POINT('Ctrl Pts',(-4.15989064282114,4.4828408852519,9.03111111013541));
#7698=CARTESIAN_POINT('Ctrl Pts',(-4.28264765377203,4.36571856902371,9.03883587223861));
#7699=CARTESIAN_POINT('Ctrl Pts',(-4.40033892611598,4.24368270465741,9.04656063434181));
#7700=CARTESIAN_POINT('Ctrl Pts',(-4.51800724056737,4.12167064567792,9.05428388958511));
#7701=CARTESIAN_POINT('Ctrl Pts',(-4.63061156829005,3.99474717905708,9.0620071448284));
#7702=CARTESIAN_POINT('Ctrl Pts',(-4.73775321406145,3.86335605984621,9.06973040007171));
#7703=CARTESIAN_POINT('Ctrl Pts',(-4.84489900034333,3.73195986299908,9.07745395378176));
#7704=CARTESIAN_POINT('Ctrl Pts',(-4.94658147888625,3.59609591117928,9.08517750749182));
#7705=CARTESIAN_POINT('Ctrl Pts',(-5.04244204692123,3.45624127715945,9.09290106120187));
#7706=CARTESIAN_POINT('Ctrl Pts',(-5.13829617652533,3.31639603641169,9.100624096163));
#7707=CARTESIAN_POINT('Ctrl Pts',(-5.22832899893599,3.17256091128272,9.10834713112413));
#7708=CARTESIAN_POINT('Ctrl Pts',(-5.31222498382503,3.02524235123819,9.11607016608525));
#7709=CARTESIAN_POINT('Ctrl Pts',(-5.39614326461181,2.87788464033853,9.12379525349261));
#7710=CARTESIAN_POINT('Ctrl Pts',(-5.47392129009374,2.72704191917447,9.13152034089997));
#7711=CARTESIAN_POINT('Ctrl Pts',(-5.5452888153366,2.5732464936346,9.13924542830732));
#7712=CARTESIAN_POINT('Ctrl Pts',(-5.61637960126538,2.42004743514583,9.14694056041802));
#7713=CARTESIAN_POINT('Ctrl Pts',(-5.68110941194921,2.26391882752246,9.15463569252872));
#7714=CARTESIAN_POINT('Ctrl Pts',(-5.73925813199411,2.10540771748361,9.16233082463941));
#7715=CARTESIAN_POINT('Ctrl Pts',(-5.79753362347359,1.9465510335301,9.17004273309422));
#7716=CARTESIAN_POINT('Ctrl Pts',(-5.84922072930545,1.78524288839063,9.17775464154903));
#7717=CARTESIAN_POINT('Ctrl Pts',(-5.89413163322722,1.62204742615319,9.18546655000383));
#7718=CARTESIAN_POINT('Ctrl Pts',(-5.93903523272857,1.4588785064291,9.19317720417479));
#7719=CARTESIAN_POINT('Ctrl Pts',(-5.97716474304143,1.2938231890582,9.20088785834574));
#7720=CARTESIAN_POINT('Ctrl Pts',(-6.00838243299909,1.12746002205309,9.20859851251669));
#7721=CARTESIAN_POINT('Ctrl Pts',(-6.03959582536704,0.961119757467542,9.21630810519886));
#7722=CARTESIAN_POINT('Ctrl Pts',(-6.06389923863602,0.793472316223263,9.22401769788102));
#7723=CARTESIAN_POINT('Ctrl Pts',(-6.0812061301577,0.625106043029861,9.23172729056319));
#7724=CARTESIAN_POINT('Ctrl Pts',(-6.09851354978445,0.456734632282888,9.23943711849701));
#7725=CARTESIAN_POINT('Ctrl Pts',(-6.10882398799324,0.287644663002158,9.24714694643083));
#7726=CARTESIAN_POINT('Ctrl Pts',(-6.11210274251537,0.118429841830782,9.25485677436465));
#7727=CARTESIAN_POINT('Ctrl Pts',(-6.11286853846333,0.0789075099477037,
9.25665750538959));
#7728=CARTESIAN_POINT('Ctrl Pts',(-6.1132509679055,0.0393783782833313,9.25845823641453));
#7729=CARTESIAN_POINT('Ctrl Pts',(-6.11324999816033,-0.000149975753035227,
9.26025896743946));
#7730=CARTESIAN_POINT('Ctrl Pts',(-6.11324999816031,-0.000149976428034141,
9.26025896747021));
#7731=CARTESIAN_POINT('Ctrl Pts',(-6.11324566360336,-0.176832609976691,
9.26830782018757));
#7732=CARTESIAN_POINT('Ctrl Pts',(-6.10557737691335,-0.35347768337121,9.27635667290493));
#7733=CARTESIAN_POINT('Ctrl Pts',(-6.0902808612631,-0.529437997722481,9.28440552562229));
#7734=CARTESIAN_POINT('Ctrl Pts',(-6.07959408821543,-0.652371088359816,
9.29002878416372));
#7735=CARTESIAN_POINT('Ctrl Pts',(-6.06518507130406,-0.774969979963666,
9.29565204270516));
#7736=CARTESIAN_POINT('Ctrl Pts',(-6.04708101675142,-0.897015462154686,
9.30127530124659));
#7737=CARTESIAN_POINT('Ctrl Pts',(-6.02221118131847,-1.06467133441257,9.30900006334979));
#7738=CARTESIAN_POINT('Ctrl Pts',(-5.99036023379552,-1.23132198049045,9.316724825453));
#7739=CARTESIAN_POINT('Ctrl Pts',(-5.95163401593469,-1.39638035752052,9.3244495875562));
#7740=CARTESIAN_POINT('Ctrl Pts',(-5.91291535234972,-1.56140653681524,9.33217284279952));
#7741=CARTESIAN_POINT('Ctrl Pts',(-5.86732416685052,-1.72484075846385,9.33989609804284));
#7742=CARTESIAN_POINT('Ctrl Pts',(-5.81501714435499,-1.88610741299576,9.34761935328616));
#7743=CARTESIAN_POINT('Ctrl Pts',(-5.76270810044427,-2.04738029970932,9.35534290699621));
#7744=CARTESIAN_POINT('Ctrl Pts',(-5.70368279420213,-2.20648514900584,9.36306646070626));
#7745=CARTESIAN_POINT('Ctrl Pts',(-5.63814764407514,-2.36286197356298,9.3707900144163));
#7746=CARTESIAN_POINT('Ctrl Pts',(-5.57261689558631,-2.51922829514276,9.37851304937742));
#7747=CARTESIAN_POINT('Ctrl Pts',(-5.50057730069756,-2.67286666632751,9.38623608433854));
#7748=CARTESIAN_POINT('Ctrl Pts',(-5.42228331574657,-2.82323736272322,9.39395911929966));
#7749=CARTESIAN_POINT('Ctrl Pts',(-5.34396852366531,-2.97364802109903,9.40168420670701));
#7750=CARTESIAN_POINT('Ctrl Pts',(-5.25939616468751,-3.12078898709069,9.40940929411436));
#7751=CARTESIAN_POINT('Ctrl Pts',(-5.16886697504909,-3.26414456737855,9.41713438152172));
#7752=CARTESIAN_POINT('Ctrl Pts',(-5.07868882722921,-3.40694426283186,9.42482951363241));
#7753=CARTESIAN_POINT('Ctrl Pts',(-4.98260015775692,-3.54598763055786,9.4325246457431));
#7754=CARTESIAN_POINT('Ctrl Pts',(-4.880941269523,-3.68079310556396,9.44021977785379));
#7755=CARTESIAN_POINT('Ctrl Pts',(-4.77889094524181,-3.81611764706001,9.44794453995699));
#7756=CARTESIAN_POINT('Ctrl Pts',(-4.6711912537948,-3.94721950501217,9.4556693020602));
#7757=CARTESIAN_POINT('Ctrl Pts',(-4.55821599606418,-4.07363381954301,9.4633940641634));
#7758=CARTESIAN_POINT('Ctrl Pts',(-4.44526277627839,-4.20002347458872,9.47111731940674));
#7759=CARTESIAN_POINT('Ctrl Pts',(-4.32703625468782,-4.3217271745893,9.47884057465008));
#7760=CARTESIAN_POINT('Ctrl Pts',(-4.20394940881419,-4.43831442448941,9.48656382989342));
#7761=CARTESIAN_POINT('Ctrl Pts',(-4.08085780622533,-4.55490617992661,9.49428738360347));
#7762=CARTESIAN_POINT('Ctrl Pts',(-3.95290573086101,-4.6663808687876,9.50201093731352));
#7763=CARTESIAN_POINT('Ctrl Pts',(-3.82054235846018,-4.77234550820784,9.50973449102357));
#7764=CARTESIAN_POINT('Ctrl Pts',(-3.68818787618433,-4.87830303056184,9.51745752598469));
#7765=CARTESIAN_POINT('Ctrl Pts',(-3.55142293722101,-4.97875104598478,9.52518056094581));
#7766=CARTESIAN_POINT('Ctrl Pts',(-3.41072920625785,-5.07333734775047,9.53290359590693));
#7767=CARTESIAN_POINT('Ctrl Pts',(-3.2699980850303,-5.16794878643452,9.54062868331429));
#7768=CARTESIAN_POINT('Ctrl Pts',(-3.12533634741829,-5.25669521986794,9.54835377072166));
#7769=CARTESIAN_POINT('Ctrl Pts',(-2.97725480052742,-5.33926768529509,9.55607885812901));
#7770=CARTESIAN_POINT('Ctrl Pts',(-2.82974746418462,-5.42151996240964,9.56377399023967));
#7771=CARTESIAN_POINT('Ctrl Pts',(-2.67884708152624,-5.49764594366959,9.57146912235032));
#7772=CARTESIAN_POINT('Ctrl Pts',(-2.52508287618065,-5.5673855651391,9.57916425446097));
#7773=CARTESIAN_POINT('Ctrl Pts',(-2.37072660403329,-5.63739371799112,9.58688901656417));
#7774=CARTESIAN_POINT('Ctrl Pts',(-2.21342973040418,-5.70099099971579,9.59461377866736));
#7775=CARTESIAN_POINT('Ctrl Pts',(-2.05374290216678,-5.75794804199374,9.60233854077056));
#7776=CARTESIAN_POINT('Ctrl Pts',(-1.89408722384319,-5.81489397373129,9.61006179601388));
#7777=CARTESIAN_POINT('Ctrl Pts',(-1.73204281948366,-5.86520214420964,9.61778505125721));
#7778=CARTESIAN_POINT('Ctrl Pts',(-1.56817829685562,-5.90869210500691,9.62550830650053));
#7779=CARTESIAN_POINT('Ctrl Pts',(-1.40430744165072,-5.95218374648231,9.63323186021058));
#7780=CARTESIAN_POINT('Ctrl Pts',(-1.23861663272228,-5.98885656589006,9.64095541392063));
#7781=CARTESIAN_POINT('Ctrl Pts',(-1.07168831750803,-6.01858037352803,9.64867896763067));
#7782=CARTESIAN_POINT('Ctrl Pts',(-0.904771213957228,-6.04830218478014,
9.65640200259179));
#7783=CARTESIAN_POINT('Ctrl Pts',(-0.736617082500552,-6.07107586270196,
9.66412503755291));
#7784=CARTESIAN_POINT('Ctrl Pts',(-0.567817391472592,-6.08682256784615,
9.67184807251403));
#7785=CARTESIAN_POINT('Ctrl Pts',(-0.39897284084057,-6.10257345777856,9.67957315992139));
#7786=CARTESIAN_POINT('Ctrl Pts',(-0.22948270339204,-6.11129361166031,9.68729824732874));
#7787=CARTESIAN_POINT('Ctrl Pts',(-0.0599433489993579,-6.11295610628857,
9.69502333473609));
#7788=CARTESIAN_POINT('Ctrl Pts',(0.108938588669152,-6.11461215432054,9.70271846684678));
#7789=CARTESIAN_POINT('Ctrl Pts',(0.277869049776686,-6.10926520944416,9.71041359895747));
#7790=CARTESIAN_POINT('Ctrl Pts',(0.446258887046951,-6.09694009878985,9.71810873106816));
#7791=CARTESIAN_POINT('Ctrl Pts',(0.615297106898085,-6.08456753047905,9.72583349317136));
#7792=CARTESIAN_POINT('Ctrl Pts',(0.783850397435319,-6.06515853912477,9.73355825527457));
#7793=CARTESIAN_POINT('Ctrl Pts',(0.951325484752262,-6.03877515598659,9.74128301737777));
#7794=CARTESIAN_POINT('Ctrl Pts',(1.1187679029092,-6.01239691942262,9.7490062726211));
#7795=CARTESIAN_POINT('Ctrl Pts',(1.28513222464177,-5.97904705502086,9.75672952786443));
#7796=CARTESIAN_POINT('Ctrl Pts',(1.44983280882339,-5.93883914489686,9.76445278310776));
#7797=CARTESIAN_POINT('Ctrl Pts',(1.6145397578916,-5.89862968093024,9.77217633681781));
#7798=CARTESIAN_POINT('Ctrl Pts',(1.77758253193398,-5.85156171221188,9.77989989052787));
#7799=CARTESIAN_POINT('Ctrl Pts',(1.93838738208954,-5.7977995756542,9.78762344423792));
#7800=CARTESIAN_POINT('Ctrl Pts',(2.09918143186151,-5.74404105000564,9.79534647919905));
#7801=CARTESIAN_POINT('Ctrl Pts',(2.25773755793989,-5.68358935676934,9.80306951416018));
#7802=CARTESIAN_POINT('Ctrl Pts',(2.41349865744236,-5.61665824071787,9.81079254912131));
#7803=CARTESIAN_POINT('Ctrl Pts',(2.56930115145921,-5.54970933729166,9.81851763652867));
#7804=CARTESIAN_POINT('Ctrl Pts',(2.72230684236503,-5.47627769338708,9.82624272393604));
#7805=CARTESIAN_POINT('Ctrl Pts',(2.87197916135893,-5.39662498782527,9.8339678113434));
#7806=CARTESIAN_POINT('Ctrl Pts',(3.02107110132431,-5.3172811487271,9.84166294345405));
#7807=CARTESIAN_POINT('Ctrl Pts',(3.16685521437114,-5.23176458370965,9.8493580755647));
#7808=CARTESIAN_POINT('Ctrl Pts',(3.30882603292164,-5.14037895941146,9.85705320767535));
#7809=CARTESIAN_POINT('Ctrl Pts',(3.45078320703718,-5.04900211794075,9.86474760022748));
#7810=CARTESIAN_POINT('Ctrl Pts',(3.58897790024294,-4.95172510966648,9.8724419927796));
#7811=CARTESIAN_POINT('Ctrl Pts',(3.72292453512037,-4.84888218750454,9.88013638533173));
#7812=CARTESIAN_POINT('',(-6.113249999346,-8.94212127014783E-5,9.1147410326001));
#7813=CARTESIAN_POINT('Ctrl Pts',(-6.113249999346,-8.94212126777935E-5,
9.1147410326001));
#7814=CARTESIAN_POINT('Ctrl Pts',(-6.11324745823273,-0.173811743037197,
9.12265381564133));
#7815=CARTESIAN_POINT('Ctrl Pts',(-6.10583548873119,-0.347505304511466,
9.13056659868255));
#7816=CARTESIAN_POINT('Ctrl Pts',(-6.09104741134544,-0.520544902234175,
9.13847938172378));
#7817=CARTESIAN_POINT('Ctrl Pts',(-6.07625447837759,-0.69364131653641,9.14639476288285));
#7818=CARTESIAN_POINT('Ctrl Pts',(-6.0540806237368,-0.866083056933325,9.15431014404192));
#7819=CARTESIAN_POINT('Ctrl Pts',(-6.02461106481588,-1.03724976750927,9.16222552520099));
#7820=CARTESIAN_POINT('Ctrl Pts',(-6.01454643743982,-1.09570768897857,9.16492883549211));
#7821=CARTESIAN_POINT('Ctrl Pts',(-6.00363128079267,-1.15401695675892,9.16763214578322));
#7822=CARTESIAN_POINT('Ctrl Pts',(-5.99187036227722,-1.2121530943589,9.17033545607434));
#7823=CARTESIAN_POINT('Ctrl Pts',(-5.95826330727307,-1.3782782461899,9.17806021817753));
#7824=CARTESIAN_POINT('Ctrl Pts',(-5.91773729124733,-1.54303431655236,9.18578498028072));
#7825=CARTESIAN_POINT('Ctrl Pts',(-5.87042872341687,-1.70584060386138,9.19350974238391));
#7826=CARTESIAN_POINT('Ctrl Pts',(-5.82312938401064,-1.86861513274787,9.20123299762724));
#7827=CARTESIAN_POINT('Ctrl Pts',(-5.76905022116773,-2.02944033334585,9.20895625287057));
#7828=CARTESIAN_POINT('Ctrl Pts',(-5.70837781947927,-2.18774958177967,9.2166795081139));
#7829=CARTESIAN_POINT('Ctrl Pts',(-5.64770307309394,-2.34606494810545,9.22440306182395));
#7830=CARTESIAN_POINT('Ctrl Pts',(-5.58043468771526,-2.50186387035847,9.23212661553399));
#7831=CARTESIAN_POINT('Ctrl Pts',(-5.50680809604756,-2.65459792733382,9.23985016924404));
#7832=CARTESIAN_POINT('Ctrl Pts',(-5.43318644947603,-2.80732172599649,9.24757320420515));
#7833=CARTESIAN_POINT('Ctrl Pts',(-5.35320758884491,-2.95698078580961,9.25529623916626));
#7834=CARTESIAN_POINT('Ctrl Pts',(-5.26715385886396,-3.10304943395275,9.26301927412738));
#7835=CARTESIAN_POINT('Ctrl Pts',(-5.18107725955049,-3.24915690077911,9.27074436153473));
#7836=CARTESIAN_POINT('Ctrl Pts',(-5.08892272395834,-3.3916717749005,9.27846944894209));
#7837=CARTESIAN_POINT('Ctrl Pts',(-4.99101755607863,-3.53009480289339,9.28619453634944));
#7838=CARTESIAN_POINT('Ctrl Pts',(-4.89349203158589,-3.66798107283438,9.29388966846014));
#7839=CARTESIAN_POINT('Ctrl Pts',(-4.79026060016387,-3.80180693758459,9.30158480057083));
#7840=CARTESIAN_POINT('Ctrl Pts',(-4.68168829277586,-3.93110929532434,9.30927993268153));
#7841=CARTESIAN_POINT('Ctrl Pts',(-4.57269792932238,-4.06090952988217,9.31700469478473));
#7842=CARTESIAN_POINT('Ctrl Pts',(-4.45828685419007,-4.18619730495752,9.32472945688792));
#7843=CARTESIAN_POINT('Ctrl Pts',(-4.33885267649468,-4.30652795348816,9.33245421899112));
#7844=CARTESIAN_POINT('Ctrl Pts',(-4.21944179667792,-4.42683512926671,9.34017747423445));
#7845=CARTESIAN_POINT('Ctrl Pts',(-4.09500999257646,-4.5421868831726,9.34790072947777));
#7846=CARTESIAN_POINT('Ctrl Pts',(-3.96599219842421,-4.65217491551407,9.35562398472109));
#7847=CARTESIAN_POINT('Ctrl Pts',(-3.83696941835378,-4.7621671983648,9.36334753843114));
#7848=CARTESIAN_POINT('Ctrl Pts',(-3.70336053219576,-4.86679513625091,9.3710710921412));
#7849=CARTESIAN_POINT('Ctrl Pts',(-3.56563466029741,-4.96568978408698,9.37879464585125));
#7850=CARTESIAN_POINT('Ctrl Pts',(-3.42791803869402,-5.06457778970942,9.38651768081236));
#7851=CARTESIAN_POINT('Ctrl Pts',(-3.28608524216595,-5.15773309101325,9.39424071577347));
#7852=CARTESIAN_POINT('Ctrl Pts',(-3.14063570222464,-5.24482916293867,9.40196375073458));
#7853=CARTESIAN_POINT('Ctrl Pts',(-2.99514750813191,-5.33194838120579,9.40968883814194));
#7854=CARTESIAN_POINT('Ctrl Pts',(-2.84604092094657,-5.41300498756226,9.4174139255493));
#7855=CARTESIAN_POINT('Ctrl Pts',(-2.69384221228653,-5.48771716634551,9.42513901295666));
#7856=CARTESIAN_POINT('Ctrl Pts',(-2.5422336791458,-5.56213963637039,9.43283414506734));
#7857=CARTESIAN_POINT('Ctrl Pts',(-2.38755725677093,-5.6302666858497,9.44052927717802));
#7858=CARTESIAN_POINT('Ctrl Pts',(-2.23035504983439,-5.69186629447479,9.4482244092887));
#7859=CARTESIAN_POINT('Ctrl Pts',(-2.07254753812235,-5.75370309148291,9.4559491713919));
#7860=CARTESIAN_POINT('Ctrl Pts',(-1.91213885056458,-5.80898395301959,9.4636739334951));
#7861=CARTESIAN_POINT('Ctrl Pts',(-1.7496908798326,-5.85750863315886,9.47139869559829));
#7862=CARTESIAN_POINT('Ctrl Pts',(-1.58727459762713,-5.90602384764827,9.47912195084161));
#7863=CARTESIAN_POINT('Ctrl Pts',(-1.42282012948558,-5.94778541980937,9.48684520608493));
#7864=CARTESIAN_POINT('Ctrl Pts',(-1.25690474502644,-5.98264289628171,9.49456846132825));
#7865=CARTESIAN_POINT('Ctrl Pts',(-1.09098294873446,-6.01750171982813,9.5022920150383));
#7866=CARTESIAN_POINT('Ctrl Pts',(-0.923600432482852,-6.04545584474639,
9.51001556874834));
#7867=CARTESIAN_POINT('Ctrl Pts',(-0.755345657214048,-6.06640573161966,
9.51773912245839));
#7868=CARTESIAN_POINT('Ctrl Pts',(-0.587102182699702,-6.08735421140344,
9.52546215741951));
#7869=CARTESIAN_POINT('Ctrl Pts',(-0.417986880935509,-6.10129935540618,
9.53318519238063));
#7870=CARTESIAN_POINT('Ctrl Pts',(-0.248594534907554,-6.10819337609036,
9.54090822734175));
#7871=CARTESIAN_POINT('Ctrl Pts',(-0.0791571717736587,-6.11508922890489,
9.54863331474911));
#7872=CARTESIAN_POINT('Ctrl Pts',(0.0905570659481728,-6.11493019885617,
9.55635840215646));
#7873=CARTESIAN_POINT('Ctrl Pts',(0.259951216556874,-6.10772059998741,9.56408348956382));
#7874=CARTESIAN_POINT('Ctrl Pts',(0.428688513492966,-6.10053895752375,9.57177862167451));
#7875=CARTESIAN_POINT('Ctrl Pts',(0.597107890748209,-6.08636137400293,9.5794737537852));
#7876=CARTESIAN_POINT('Ctrl Pts',(0.764622306756637,-6.06524346506471,9.58716888589589));
#7877=CARTESIAN_POINT('Ctrl Pts',(0.932781734549123,-6.04404424193011,9.59489364799909));
#7878=CARTESIAN_POINT('Ctrl Pts',(1.10008877149121,-6.01584360211571,9.60261841010229));
#7879=CARTESIAN_POINT('Ctrl Pts',(1.26595420145235,-5.98073453033364,9.61034317220549));
#7880=CARTESIAN_POINT('Ctrl Pts',(1.43178727624756,-5.94563230723513,9.61806642744883));
#7881=CARTESIAN_POINT('Ctrl Pts',(1.5961789953133,-5.9036244067426,9.62578968269216));
#7882=CARTESIAN_POINT('Ctrl Pts',(1.75855046184005,-5.85485489450099,9.6335129379355));
#7883=CARTESIAN_POINT('Ctrl Pts',(1.92092820324404,-5.80608349755198,9.64123649164555));
#7884=CARTESIAN_POINT('Ctrl Pts',(2.08128523121816,-5.75055005334046,9.64896004535559));
#7885=CARTESIAN_POINT('Ctrl Pts',(2.23905718027886,-5.68844869063101,9.65668359906564));
#7886=CARTESIAN_POINT('Ctrl Pts',(2.39681853265922,-5.62635149893101,9.66440663402676));
#7887=CARTESIAN_POINT('Ctrl Pts',(2.55199485864944,-5.55768738760475,9.67212966898789));
#7888=CARTESIAN_POINT('Ctrl Pts',(2.70404100082699,-5.4826989547436,9.67985270394901));
#7889=CARTESIAN_POINT('Ctrl Pts',(2.85612755024525,-5.40769059322387,9.68757779135637));
#7890=CARTESIAN_POINT('Ctrl Pts',(3.00508196817793,-5.32635468999279,9.69530287876373));
#7891=CARTESIAN_POINT('Ctrl Pts',(3.150382110936,-5.23898063726088,9.70302796617109));
#7892=CARTESIAN_POINT('Ctrl Pts',(3.29511882849818,-5.15194539178574,9.71072309828175));
#7893=CARTESIAN_POINT('Ctrl Pts',(3.43622930968405,-5.05891892991148,9.71841823039243));
#7894=CARTESIAN_POINT('Ctrl Pts',(3.57322466611832,-4.96023094703701,9.72611336250309));
#7895=CARTESIAN_POINT('Ctrl Pts',(3.62368399696851,-4.92388132389347,9.72894770103262));
#7896=CARTESIAN_POINT('Ctrl Pts',(3.67359190198392,-4.88675930292695,9.73178203956215));
#7897=CARTESIAN_POINT('Ctrl Pts',(3.72292453512039,-4.84888218750452,9.73461637809168));
#7898=CARTESIAN_POINT('Ctrl Pts',(3.72292453512037,-4.84888218750454,7.98461472294509));
#7899=CARTESIAN_POINT('Ctrl Pts',(3.8574022678144,-4.74563149360974,7.99233781167824));
#7900=CARTESIAN_POINT('Ctrl Pts',(3.98758355070785,-4.63678185091767,8.00006090041139));
#7901=CARTESIAN_POINT('Ctrl Pts',(4.11301107379905,-4.52271660280703,8.00778398914454));
#7902=CARTESIAN_POINT('Ctrl Pts',(4.23843847491679,-4.40865146562047,8.01550707036727));
#7903=CARTESIAN_POINT('Ctrl Pts',(4.35911189315032,-4.28937094866781,8.02323015159001));
#7904=CARTESIAN_POINT('Ctrl Pts',(4.47460933368528,-4.16529673293471,8.03095323281275));
#7905=CARTESIAN_POINT('Ctrl Pts',(4.59013082874591,-4.04119667640035,8.03867792251317));
#7906=CARTESIAN_POINT('Ctrl Pts',(4.70047397780303,-3.91230115962854,8.04640261221359));
#7907=CARTESIAN_POINT('Ctrl Pts',(4.80525518851297,-3.77906709860637,8.05412730191402));
#7908=CARTESIAN_POINT('Ctrl Pts',(4.82629068090824,-3.75231951611106,8.0556780823483));
#7909=CARTESIAN_POINT('Ctrl Pts',(4.84710214032259,-3.7253971827812,8.05722886278257));
#7910=CARTESIAN_POINT('Ctrl Pts',(4.86768666217403,-3.69830395200192,8.05877964321685));
#7911=CARTESIAN_POINT('Ctrl Pts',(4.97022247626845,-3.56334689570254,8.06650440532005));
#7912=CARTESIAN_POINT('Ctrl Pts',(5.0671604439934,-3.42409909101741,8.07422916742325));
#7913=CARTESIAN_POINT('Ctrl Pts',(5.15815464990081,-3.28104650534044,8.08195392952645));
#7914=CARTESIAN_POINT('Ctrl Pts',(5.24913110568005,-3.13802182475594,8.08967718476978));
#7915=CARTESIAN_POINT('Ctrl Pts',(5.33416594314995,-2.99119411137184,8.09740044001311));
#7916=CARTESIAN_POINT('Ctrl Pts',(5.41295695714888,-2.84107770793999,8.10512369525643));
#7917=CARTESIAN_POINT('Ctrl Pts',(5.49175101604207,-2.69095550323017,8.11284724896648));
#7918=CARTESIAN_POINT('Ctrl Pts',(5.56430061782847,-2.53754463292657,8.12057080267653));
#7919=CARTESIAN_POINT('Ctrl Pts',(5.63034948816571,-2.38138409409573,8.12829435638658));
#7920=CARTESIAN_POINT('Ctrl Pts',(5.69639392236101,-2.22523404371551,8.1360173913477));
#7921=CARTESIAN_POINT('Ctrl Pts',(5.7559383753895,-2.06633498630608,8.14374042630882));
#7922=CARTESIAN_POINT('Ctrl Pts',(5.80877463804117,-1.90524611715905,8.15146346126995));
#7923=CARTESIAN_POINT('Ctrl Pts',(5.86162494226961,-1.74411443760854,8.1591885486773));
#7924=CARTESIAN_POINT('Ctrl Pts',(5.90776339285081,-1.58079208410473,8.16691363608466));
#7925=CARTESIAN_POINT('Ctrl Pts',(5.94703131228762,-1.41585455932823,8.17463872349201));
#7926=CARTESIAN_POINT('Ctrl Pts',(5.98614696390985,-1.25155660692535,8.18233385560268));
#7927=CARTESIAN_POINT('Ctrl Pts',(6.01844523195451,-1.08565629833407,8.19002898771335));
#7928=CARTESIAN_POINT('Ctrl Pts',(6.04381950108335,-0.918733585336168,8.19772411982402));
#7929=CARTESIAN_POINT('Ctrl Pts',(6.06929147346066,-0.751168138897491,8.20544888192722));
#7930=CARTESIAN_POINT('Ctrl Pts',(6.08779501129324,-0.582513047708593,8.21317364403042));
#7931=CARTESIAN_POINT('Ctrl Pts',(6.09925885820982,-0.413360548491332,8.22089840613361));
#7932=CARTESIAN_POINT('Ctrl Pts',(6.11072046888784,-0.244241045644635,8.22862166137694));
#7933=CARTESIAN_POINT('Ctrl Pts',(6.11514510730666,-0.0746246443857959,
8.23634491662026));
#7934=CARTESIAN_POINT('Ctrl Pts',(6.11251347583972,0.0948924137001474,8.24406817186359));
#7935=CARTESIAN_POINT('Ctrl Pts',(6.10988174267286,0.264416022806168,8.25179172557364));
#7936=CARTESIAN_POINT('Ctrl Pts',(6.10019319490759,0.433839964115716,8.25951527928369));
#7937=CARTESIAN_POINT('Ctrl Pts',(6.08348066331392,0.602568321093682,8.26723883299373));
#7938=CARTESIAN_POINT('Ctrl Pts',(6.06676925420973,0.771285345509321,8.27496186795485));
#7939=CARTESIAN_POINT('Ctrl Pts',(6.04303483659968,0.939306563671693,8.28268490291598));
#7940=CARTESIAN_POINT('Ctrl Pts',(6.01236211192288,1.10604131822201,8.2904079378771));
#7941=CARTESIAN_POINT('Ctrl Pts',(5.98168123577213,1.27282038360621,8.29813302528446));
#7942=CARTESIAN_POINT('Ctrl Pts',(5.94405842323202,1.43831198989677,8.30585811269181));
#7943=CARTESIAN_POINT('Ctrl Pts',(5.89962967276359,1.60193485721093,8.31358320009917));
#7944=CARTESIAN_POINT('Ctrl Pts',(5.85537320208061,1.76492324995224,8.32127833220985));
#7945=CARTESIAN_POINT('Ctrl Pts',(5.80436359484624,1.92605707780743,8.32897346432053));
#7946=CARTESIAN_POINT('Ctrl Pts',(5.74678469524245,2.08477606208128,8.33666859643122));
#7947=CARTESIAN_POINT('Ctrl Pts',(5.68898408893631,2.24410619145943,8.34439335853442));
#7948=CARTESIAN_POINT('Ctrl Pts',(5.62454300042812,2.40105926345284,8.35211812063762));
#7949=CARTESIAN_POINT('Ctrl Pts',(5.55368220100643,2.55508112840364,8.35984288274082));
#7950=CARTESIAN_POINT('Ctrl Pts',(5.48283522431398,2.70907294849812,8.36756613798415));
#7951=CARTESIAN_POINT('Ctrl Pts',(5.40557116784684,2.86013441472761,8.37528939322748));
#7952=CARTESIAN_POINT('Ctrl Pts',(5.32215834526735,3.00773271924238,8.38301264847081));
#7953=CARTESIAN_POINT('Ctrl Pts',(5.2387422991829,3.15533672772269,8.39073620218086));
#7954=CARTESIAN_POINT('Ctrl Pts',(5.1491771639691,3.29947702882138,8.39845975589091));
#7955=CARTESIAN_POINT('Ctrl Pts',(5.05377687308074,3.43964603987303,8.40618330960096));
#7956=CARTESIAN_POINT('Ctrl Pts',(4.95838298970897,3.57980563653764,8.41390634456209));
#7957=CARTESIAN_POINT('Ctrl Pts',(4.85715491329265,3.7159942149028,8.42162937952321));
#7958=CARTESIAN_POINT('Ctrl Pts',(4.75044961013144,3.84773362696822,8.42935241448434));
#7959=CARTESIAN_POINT('Ctrl Pts',(4.64371594934927,3.97950804963014,8.4370775018917));
#7960=CARTESIAN_POINT('Ctrl Pts',(4.53150235108678,4.10683069545986,8.44480258929906));
#7961=CARTESIAN_POINT('Ctrl Pts',(4.41420634043892,4.22925619305911,8.45252767670642));
#7962=CARTESIAN_POINT('Ctrl Pts',(4.29736516435994,4.35120696566036,8.46022280881708));
#7963=CARTESIAN_POINT('Ctrl Pts',(4.17548116086376,4.46829829839282,8.46791794092775));
#7964=CARTESIAN_POINT('Ctrl Pts',(4.04898382203956,4.58012615234143,8.47561307303841));
#7965=CARTESIAN_POINT('Ctrl Pts',(3.92199940708056,4.69238459778999,8.48333783514161));
#7966=CARTESIAN_POINT('Ctrl Pts',(3.79032106512151,4.79937868620239,8.49106259724481));
#7967=CARTESIAN_POINT('Ctrl Pts',(3.65440778259716,4.900727427739,8.49878735934801));
#7968=CARTESIAN_POINT('Ctrl Pts',(3.51852101251008,5.00205639930094,8.50651061459134));
#7969=CARTESIAN_POINT('Ctrl Pts',(3.37840120414425,5.09774203199839,8.51423386983468));
#7970=CARTESIAN_POINT('Ctrl Pts',(3.23453888158875,5.18744482245263,8.52195712507801));
#7971=CARTESIAN_POINT('Ctrl Pts',(3.09067099944551,5.27715107948885,8.52968067878806));
#7972=CARTESIAN_POINT('Ctrl Pts',(2.94306058052596,5.36087386057674,8.53740423249811));
#7973=CARTESIAN_POINT('Ctrl Pts',(2.79222614038394,5.43831763907337,8.54512778620816));
#7974=CARTESIAN_POINT('Ctrl Pts',(2.64140183096753,5.51575621609434,8.55285082116929));
#7975=CARTESIAN_POINT('Ctrl Pts',(2.48735421562718,5.58691648970304,8.56057385613042));
#7976=CARTESIAN_POINT('Ctrl Pts',(2.33062551577657,5.65154936877589,8.56829689109155));
#7977=CARTESIAN_POINT('Ctrl Pts',(2.17385516426556,5.71619942445221,8.57602197849891));
#7978=CARTESIAN_POINT('Ctrl Pts',(2.01440259683183,5.77431849632089,8.58374706590627));
#7979=CARTESIAN_POINT('Ctrl Pts',(1.85282996934096,5.82570567976206,8.59147215331363));
#7980=CARTESIAN_POINT('Ctrl Pts',(1.69188386628157,5.87689360094954,8.59916728542429));
#7981=CARTESIAN_POINT('Ctrl Pts',(1.52883442297593,5.92140168501278,8.60686241753494));
#7982=CARTESIAN_POINT('Ctrl Pts',(1.36425209167301,5.95908061640937,8.61455754964559));
#7983=CARTESIAN_POINT('Ctrl Pts',(1.19903603853412,5.99690462997482,8.62228231174879));
#7984=CARTESIAN_POINT('Ctrl Pts',(1.03221674792847,6.02786016224444,8.63000707385199));
#7985=CARTESIAN_POINT('Ctrl Pts',(0.864379544508043,6.05183224862818,8.63773183595519));
#7986=CARTESIAN_POINT('Ctrl Pts',(0.696575080885137,6.07579965880643,8.64545509119851));
#7987=CARTESIAN_POINT('Ctrl Pts',(0.527753414203596,6.09278629649545,8.65317834644184));
#7988=CARTESIAN_POINT('Ctrl Pts',(0.358507714816743,6.10272871598573,8.66090160168516));
#7989=CARTESIAN_POINT('Ctrl Pts',(0.189255474896465,6.11267151970278,8.6686251553952));
#7990=CARTESIAN_POINT('Ctrl Pts',(0.0195794856200138,6.11556953794196,8.67634870910525));
#7991=CARTESIAN_POINT('Ctrl Pts',(-0.149923542379877,6.11141133404881,8.6840722628153));
#7992=CARTESIAN_POINT('Ctrl Pts',(-0.319415185787106,6.10725340943951,8.69179529777642));
#7993=CARTESIAN_POINT('Ctrl Pts',(-0.488733574303142,6.09604021888496,8.69951833273755));
#7994=CARTESIAN_POINT('Ctrl Pts',(-0.657283396671435,6.07781244354908,8.70724136769867));
#7995=CARTESIAN_POINT('Ctrl Pts',(-0.825878012239498,6.05957982406463,8.71496645510603));
#7996=CARTESIAN_POINT('Ctrl Pts',(-0.993703337970038,6.03432892666479,8.72269154251339));
#7997=CARTESIAN_POINT('Ctrl Pts',(-1.16016961147651,6.00215228356516,8.73041662992074));
#7998=CARTESIAN_POINT('Ctrl Pts',(-1.32599038463506,5.97010041069001,8.73811176203142));
#7999=CARTESIAN_POINT('Ctrl Pts',(-1.49046232633288,5.93117649896973,8.74580689414211));
#8000=CARTESIAN_POINT('Ctrl Pts',(-1.65301307063605,5.88552235156799,8.75350202625279));
#8001=CARTESIAN_POINT('Ctrl Pts',(-1.81618971417897,5.83969241354607,8.76122678835599));
#8002=CARTESIAN_POINT('Ctrl Pts',(-1.97748812006645,5.78706404710313,8.76895155045919));
#8003=CARTESIAN_POINT('Ctrl Pts',(-2.1363392970195,5.7278163352634,8.7766763125624));
#8004=CARTESIAN_POINT('Ctrl Pts',(-2.29515948706802,5.66858018080225,8.78439956780572));
#8005=CARTESIAN_POINT('Ctrl Pts',(-2.45153310395785,5.60272736809181,8.79212282304904));
#8006=CARTESIAN_POINT('Ctrl Pts',(-2.60490891503397,5.53048597384322,8.79984607829236));
#8007=CARTESIAN_POINT('Ctrl Pts',(-2.75829065334869,5.45824178781163,8.80756963200241));
#8008=CARTESIAN_POINT('Ctrl Pts',(-2.90867406563048,5.37960865766176,8.81529318571245));
#8009=CARTESIAN_POINT('Ctrl Pts',(-3.05552969306556,5.29486202438691,8.8230167394225));
#8010=CARTESIAN_POINT('Ctrl Pts',(-3.20237545701001,5.21012108308068,8.83073977438362));
#8011=CARTESIAN_POINT('Ctrl Pts',(-3.34569363574495,5.11926761877613,8.83846280934474));
#8012=CARTESIAN_POINT('Ctrl Pts',(-3.48498093397388,5.02262216898091,8.84618584430586));
#8013=CARTESIAN_POINT('Ctrl Pts',(-3.62430524869861,4.92595103503552,8.85391093171321));
#8014=CARTESIAN_POINT('Ctrl Pts',(-3.7595962805231,4.82348501879639,8.86163601912057));
#8015=CARTESIAN_POINT('Ctrl Pts',(-3.89038041381802,4.71558753479151,8.86936110652793));
#8016=CARTESIAN_POINT('Ctrl Pts',(-4.02065741013091,4.60810844102275,8.8770562386386));
#8017=CARTESIAN_POINT('Ctrl Pts',(-4.14646217796333,4.49524015096725,8.88475137074928));
#8018=CARTESIAN_POINT('Ctrl Pts',(-4.26735995062769,4.37738102228705,8.89244650285996));
#8019=CARTESIAN_POINT('Ctrl Pts',(-4.38872323837968,4.25906807877299,8.90017126496315));
#8020=CARTESIAN_POINT('Ctrl Pts',(-4.50518462963113,4.13568386161381,8.90789602706634));
#8021=CARTESIAN_POINT('Ctrl Pts',(-4.61633015684259,4.00765785035669,8.91562078916953));
#8022=CARTESIAN_POINT('Ctrl Pts',(-4.72745400303229,3.87965681297668,8.92334404441284));
#8023=CARTESIAN_POINT('Ctrl Pts',(-4.83326384664574,3.7470160274108,8.93106729965615));
#8024=CARTESIAN_POINT('Ctrl Pts',(-4.93338475446752,3.61019949959659,8.93879055489947));
#8025=CARTESIAN_POINT('Ctrl Pts',(-5.03350953148165,3.4733776844805,8.94651410860951));
#8026=CARTESIAN_POINT('Ctrl Pts',(-5.1279447424171,3.33238005761311,8.95423766231956));
#8027=CARTESIAN_POINT('Ctrl Pts',(-5.21635723469462,3.18770179950212,8.96196121602961));
#8028=CARTESIAN_POINT('Ctrl Pts',(-5.3047637887878,3.04303325863974,8.96968425099072));
#8029=CARTESIAN_POINT('Ctrl Pts',(-5.38714826845094,2.89468485169631,8.97740728595184));
#8030=CARTESIAN_POINT('Ctrl Pts',(-5.46322207146371,2.74317884221421,8.98513032091295));
#8031=CARTESIAN_POINT('Ctrl Pts',(-5.53931609157915,2.59163256903522,8.9928554083203));
#8032=CARTESIAN_POINT('Ctrl Pts',(-5.60909593952382,2.43692729893481,9.00058049572766));
#8033=CARTESIAN_POINT('Ctrl Pts',(-5.67231958918843,2.27960874726546,9.00830558313501));
#8034=CARTESIAN_POINT('Ctrl Pts',(-5.73529807875576,2.12290022414772,9.01600071524572));
#8035=CARTESIAN_POINT('Ctrl Pts',(-5.79177103862998,1.96359895198479,9.02369584735643));
#8036=CARTESIAN_POINT('Ctrl Pts',(-5.84154727478895,1.80226274413744,9.03139097946714));
#8037=CARTESIAN_POINT('Ctrl Pts',(-5.89171153494281,1.63966886144922,9.03914609795154));
#8038=CARTESIAN_POINT('Ctrl Pts',(-5.93509151719397,1.47495225274229,9.04690121643594));
#8039=CARTESIAN_POINT('Ctrl Pts',(-5.97152821508267,1.30869260675361,9.05465633492034));
#8040=CARTESIAN_POINT('Ctrl Pts',(-6.00795675422069,1.14247018891895,9.06240971691153));
#8041=CARTESIAN_POINT('Ctrl Pts',(-6.03744504534487,0.974705727749124,9.07016309890272));
#8042=CARTESIAN_POINT('Ctrl Pts',(-6.05988488740563,0.805990517247494,9.07791648089391));
#8043=CARTESIAN_POINT('Ctrl Pts',(-6.08232272788607,0.637290355739623,9.08566917130195));
#8044=CARTESIAN_POINT('Ctrl Pts',(-6.09771333128856,0.467639922840535,9.09342186171));
#8045=CARTESIAN_POINT('Ctrl Pts',(-6.10600010853084,0.297637761585123,9.10117455211803));
#8046=CARTESIAN_POINT('Ctrl Pts',(-6.11083380261946,0.198475153747465,9.10569671226554));
#8047=CARTESIAN_POINT('Ctrl Pts',(-6.11325145157963,0.0991929884357902,
9.11021887241305));
#8048=CARTESIAN_POINT('Ctrl Pts',(-6.11324999934601,-8.94203443601632E-5,
9.11474103256055));
#8049=CARTESIAN_POINT('Origin',(0.,0.,-3.86474103256053));
#8050=CARTESIAN_POINT('',(3.72292453512036,-4.84888218750454,6.23460979329304));
#8051=CARTESIAN_POINT('',(3.72323907905152,-4.84929205898336,6.38013065756227));
#8052=CARTESIAN_POINT('',(3.72292453512038,-4.84888218750453,-3.86474103256053));
#8053=CARTESIAN_POINT('',(-6.11324999906832,0.000106729296146127,7.51025896743946));
#8054=CARTESIAN_POINT('Ctrl Pts',(3.72323907905155,-4.84929205898333,6.38013065756227));
#8055=CARTESIAN_POINT('Ctrl Pts',(3.74244957685544,-4.83454974172044,6.38123420254007));
#8056=CARTESIAN_POINT('Ctrl Pts',(4.56407058896953,-4.19609180936438,6.4286525730536));
#8057=CARTESIAN_POINT('Ctrl Pts',(5.85647901784331,-2.51246545019524,6.52238576910286));
#8058=CARTESIAN_POINT('Ctrl Pts',(6.34476406083597,0.595649340793697,6.66133024571005));
#8059=CARTESIAN_POINT('Ctrl Pts',(5.28652688781551,3.55857592152639,6.80027472231724));
#8060=CARTESIAN_POINT('Ctrl Pts',(2.93971047068678,5.65410748689819,6.93921919892443));
#8061=CARTESIAN_POINT('Ctrl Pts',(-0.123653876037357,6.37146284959777,7.07816367553161));
#8062=CARTESIAN_POINT('Ctrl Pts',(-3.15687786378923,5.53578822553583,7.2171081521388));
#8063=CARTESIAN_POINT('Ctrl Pts',(-5.42061984988151,3.35077745723799,7.35605262874599));
#8064=CARTESIAN_POINT('Ctrl Pts',(-6.0834461464926,1.23970149668133,7.45376956717954));
#8065=CARTESIAN_POINT('Ctrl Pts',(-6.11370812977969,0.111745833966236,7.50517168007736));
#8066=CARTESIAN_POINT('Ctrl Pts',(-6.11361710986571,0.000106735705416132,
7.51025896743946));
#8067=CARTESIAN_POINT('Ctrl Pts',(-6.11324999906832,0.000106729296146127,
7.51025896743946));
#8068=CARTESIAN_POINT('Ctrl Pts',(-6.11325294774147,-0.168787630489055,
7.51795578481954));
#8069=CARTESIAN_POINT('Ctrl Pts',(-6.10625233739568,-0.33771293236707,7.52565260219963));
#8070=CARTESIAN_POINT('Ctrl Pts',(-6.09226654106778,-0.506077024854876,
7.53334941957971));
#8071=CARTESIAN_POINT('Ctrl Pts',(-6.07828327346374,-0.674410676008743,
7.54104484532465));
#8072=CARTESIAN_POINT('Ctrl Pts',(-6.05731736650498,-0.842183000067764,
7.54874027106959));
#8073=CARTESIAN_POINT('Ctrl Pts',(-6.02943916153457,-1.00880570966528,7.55643569681453));
#8074=CARTESIAN_POINT('Ctrl Pts',(-6.0015598834746,-1.1754348329143,7.56413141877227));
#8075=CARTESIAN_POINT('Ctrl Pts',(-5.96676782543536,-1.34091393569506,7.57182714073001));
#8076=CARTESIAN_POINT('Ctrl Pts',(-5.92518479316057,-1.50466299529121,7.57952286268775));
#8077=CARTESIAN_POINT('Ctrl Pts',(-5.88360268844497,-1.66840840226907,7.58721841298322));
#8078=CARTESIAN_POINT('Ctrl Pts',(-5.83522999381734,-1.8304235322667,7.5949139632787));
#8079=CARTESIAN_POINT('Ctrl Pts',(-5.78023897185452,-1.9901414499362,7.60260951357417));
#8080=CARTESIAN_POINT('Ctrl Pts',(-5.72523548542042,-2.14989556986797,7.61030680817193));
#8081=CARTESIAN_POINT('Ctrl Pts',(-5.66361078029505,-2.30735113356998,7.6180041027697));
#8082=CARTESIAN_POINT('Ctrl Pts',(-5.59558629701935,-2.46195847956648,7.62570139736746));
#8083=CARTESIAN_POINT('Ctrl Pts',(-5.57131221422705,-2.51712907897855,7.6284481255651));
#8084=CARTESIAN_POINT('Ctrl Pts',(-5.5462236479206,-2.57193717972177,7.63119485376273));
#8085=CARTESIAN_POINT('Ctrl Pts',(-5.52033212740917,-2.62635846098626,7.63394158196037));
#8086=CARTESIAN_POINT('Ctrl Pts',(-5.4475160997392,-2.77941017228462,7.64166634406357));
#8087=CARTESIAN_POINT('Ctrl Pts',(-5.36831819637481,-2.92945887370836,7.64939110616676));
#8088=CARTESIAN_POINT('Ctrl Pts',(-5.28301132117769,-3.07597414534133,7.65711586826996));
#8089=CARTESIAN_POINT('Ctrl Pts',(-5.197721086688,-3.22246083642012,7.6648391235133));
#8090=CARTESIAN_POINT('Ctrl Pts',(-5.10632441754276,-3.36541519931389,7.67256237875664));
#8091=CARTESIAN_POINT('Ctrl Pts',(-5.00913949382559,-3.50433261747465,7.68028563399997));
#8092=CARTESIAN_POINT('Ctrl Pts',(-4.91195081437798,-3.64325540412627,7.68800918771002));
#8093=CARTESIAN_POINT('Ctrl Pts',(-4.80897361116746,-3.77814067191202,7.69573274142008));
#8094=CARTESIAN_POINT('Ctrl Pts',(-4.70056905431399,-3.90851328872317,7.70345629513013));
#8095=CARTESIAN_POINT('Ctrl Pts',(-4.59217177840257,-4.03887714911768,7.71117933009126));
#8096=CARTESIAN_POINT('Ctrl Pts',(-4.47834808097592,-4.1647287213615,7.71890236505238));
#8097=CARTESIAN_POINT('Ctrl Pts',(-4.35949914342364,-4.28562629973596,7.72662540001351));
#8098=CARTESIAN_POINT('Ctrl Pts',(-4.24061862100162,-4.40655600741964,7.73435048742087));
#8099=CARTESIAN_POINT('Ctrl Pts',(-4.11671041060107,-4.52252886274096,7.74207557482822));
#8100=CARTESIAN_POINT('Ctrl Pts',(-3.98821292170116,-4.63313967560615,7.74980066223558));
#8101=CARTESIAN_POINT('Ctrl Pts',(-3.86021370294402,-4.74332157685611,7.75749579434623));
#8102=CARTESIAN_POINT('Ctrl Pts',(-3.72766099141761,-4.84818276689439,7.76519092645689));
#8103=CARTESIAN_POINT('Ctrl Pts',(-3.59102105187657,-4.9473622636188,7.77288605856754));
#8104=CARTESIAN_POINT('Ctrl Pts',(-3.4538549822663,-5.0469236495306,7.78061082067074));
#8105=CARTESIAN_POINT('Ctrl Pts',(-3.31252154875908,-5.14079473810075,7.78833558277394));
#8106=CARTESIAN_POINT('Ctrl Pts',(-3.16751416376062,-5.22864031894295,7.79606034487714));
#8107=CARTESIAN_POINT('Ctrl Pts',(-3.02253506517465,-5.31646876385559,7.80378360012048));
#8108=CARTESIAN_POINT('Ctrl Pts',(-2.87388371601856,-5.39827388224882,7.81150685536382));
#8109=CARTESIAN_POINT('Ctrl Pts',(-2.72208094184447,-5.47376478381627,7.81923011060717));
#8110=CARTESIAN_POINT('Ctrl Pts',(-2.5702723012226,-5.5492586027443,7.82695366431721));
#8111=CARTESIAN_POINT('Ctrl Pts',(-2.41531227388109,-5.61843757189667,7.83467721802726));
#8112=CARTESIAN_POINT('Ctrl Pts',(-2.2577453298272,-5.6810572597135,7.84240077173731));
#8113=CARTESIAN_POINT('Ctrl Pts',(-2.10018896868471,-5.74367274170778,7.85012380669842));
#8114=CARTESIAN_POINT('Ctrl Pts',(-1.94002633576995,-5.79972970692885,7.85784684165953));
#8115=CARTESIAN_POINT('Ctrl Pts',(-1.77782104386801,-5.8490322189641,7.86556987662064));
#8116=CARTESIAN_POINT('Ctrl Pts',(-1.61557264486594,-5.89834783345918,7.87329496402799));
#8117=CARTESIAN_POINT('Ctrl Pts',(-1.45128080493979,-5.94090531352668,7.88102005143534));
#8118=CARTESIAN_POINT('Ctrl Pts',(-1.28552435768903,-5.97655859908428,7.88874513884269));
#8119=CARTESIAN_POINT('Ctrl Pts',(-1.12041065831811,-6.01207363316459,7.89644027095337));
#8120=CARTESIAN_POINT('Ctrl Pts',(-0.953844001930205,-6.04073788771953,
7.90413540306405));
#8121=CARTESIAN_POINT('Ctrl Pts',(-0.786406532173293,-6.06245744963667,
7.91183053517473));
#8122=CARTESIAN_POINT('Ctrl Pts',(-0.618324346912324,-6.08426064240615,
7.91955529727793));
#8123=CARTESIAN_POINT('Ctrl Pts',(-0.449305095290647,-6.0990732477667,7.92728005938114));
#8124=CARTESIAN_POINT('Ctrl Pts',(-0.279942430074679,-6.10683697165266,
7.93500482148434));
#8125=CARTESIAN_POINT('Ctrl Pts',(-0.110612802225837,-6.11459918107854,
7.94272807672769));
#8126=CARTESIAN_POINT('Ctrl Pts',(0.0590597891480183,-6.11531523817638,
7.95045133197104));
#8127=CARTESIAN_POINT('Ctrl Pts',(0.228478823103353,-6.10897888275064,7.95817458721439));
#8128=CARTESIAN_POINT('Ctrl Pts',(0.397904404290227,-6.10264228245522,7.96589814092444));
#8129=CARTESIAN_POINT('Ctrl Pts',(0.567076091606076,-6.08925273214945,7.97362169463449));
#8130=CARTESIAN_POINT('Ctrl Pts',(0.735398828517154,-6.06885608047477,7.98134524834454));
#8131=CARTESIAN_POINT('Ctrl Pts',(0.903710260109033,-6.04846079873182,7.98906828330565));
#8132=CARTESIAN_POINT('Ctrl Pts',(1.07117254074636,-6.0210593955603,7.99679131826677));
#8133=CARTESIAN_POINT('Ctrl Pts',(1.23719700561922,-5.98674946292116,8.00451435322789));
#8134=CARTESIAN_POINT('Ctrl Pts',(1.40326559256198,-5.95243041219664,8.01223944063524));
#8135=CARTESIAN_POINT('Ctrl Pts',(1.56789528916575,-5.91119922530853,8.0199645280426));
#8136=CARTESIAN_POINT('Ctrl Pts',(1.73050792712124,-5.86320457400819,8.02768961544995));
#8137=CARTESIAN_POINT('Ctrl Pts',(1.89249000783377,-5.81539602986029,8.03538474756061));
#8138=CARTESIAN_POINT('Ctrl Pts',(2.05247035474955,-5.76087650024044,8.04307987967126));
#8139=CARTESIAN_POINT('Ctrl Pts',(2.20989284155477,-5.69984203213957,8.05077501178192));
#8140=CARTESIAN_POINT('Ctrl Pts',(2.36792369396233,-5.63857169385457,8.05849988204356));
#8141=CARTESIAN_POINT('Ctrl Pts',(2.5234328366786,-5.5707142337554,8.0662247523052));
#8142=CARTESIAN_POINT('Ctrl Pts',(2.67587105519959,-5.49650249326288,8.07394962256685));
#8143=CARTESIAN_POINT('Ctrl Pts',(2.82827703775813,-5.42230644625525,8.08167285925766));
#8144=CARTESIAN_POINT('Ctrl Pts',(2.97761310740808,-5.34175893929577,8.08939609594846));
#8145=CARTESIAN_POINT('Ctrl Pts',(3.12335245258178,-5.25513986678294,8.09711933263927));
#8146=CARTESIAN_POINT('Ctrl Pts',(3.2690827895958,-5.16852614820137,8.10484209195625));
#8147=CARTESIAN_POINT('Ctrl Pts',(3.4112165726881,-5.07584177357938,8.11256485127323));
#8148=CARTESIAN_POINT('Ctrl Pts',(3.54925335581439,-4.97741159426667,8.12028761059021));
#8149=CARTESIAN_POINT('Ctrl Pts',(3.60789506958217,-4.93559582407384,8.12356844509756));
#8150=CARTESIAN_POINT('Ctrl Pts',(3.6657977138052,-4.89274360472679,8.1268492796049));
#8151=CARTESIAN_POINT('Ctrl Pts',(3.72292453512038,-4.84888218750453,8.13013011411225));
#8152=CARTESIAN_POINT('',(-6.11324999999769,5.31886132084791E-6,7.36474103251824));
#8153=CARTESIAN_POINT('Ctrl Pts',(-6.11324999999769,5.31793291456405E-6,
7.36474103256055));
#8154=CARTESIAN_POINT('Ctrl Pts',(-6.11325014740321,-0.169445255362402,
7.37246397694535));
#8155=CARTESIAN_POINT('Ctrl Pts',(-6.10620055882416,-0.338926118695248,
7.38018692133014));
#8156=CARTESIAN_POINT('Ctrl Pts',(-6.09211972579428,-0.507841322745799,
7.38790986571494));
#8157=CARTESIAN_POINT('Ctrl Pts',(-6.07804165032709,-0.676723446774617,
7.39563129765348));
#8158=CARTESIAN_POINT('Ctrl Pts',(-6.05693510430396,-0.845039816620301,
7.40335272959201));
#8159=CARTESIAN_POINT('Ctrl Pts',(-6.0288705499934,-1.01219832736588,7.41107416153055));
#8160=CARTESIAN_POINT('Ctrl Pts',(-6.00080494970368,-1.17936306818789,7.4187958812505));
#8161=CARTESIAN_POINT('Ctrl Pts',(-5.96578087081875,-1.3453695500608,7.42651760097044));
#8162=CARTESIAN_POINT('Ctrl Pts',(-5.92392026267643,-1.5096338244593,7.43423932069038));
#8163=CARTESIAN_POINT('Ctrl Pts',(-5.88206240640404,-1.67388730030668,7.44196053279304));
#8164=CARTESIAN_POINT('Ctrl Pts',(-5.83336899865677,-1.83639849045815,7.44968174489571));
#8165=CARTESIAN_POINT('Ctrl Pts',(-5.77801247941001,-1.99659644151795,7.45740295699837));
#8166=CARTESIAN_POINT('Ctrl Pts',(-5.72264136364105,-2.15683663390691,7.4651262050463));
#8167=CARTESIAN_POINT('Ctrl Pts',(-5.66060372734563,-2.3147620676604,7.47284945309423));
#8168=CARTESIAN_POINT('Ctrl Pts',(-5.5921213109299,-2.46981878006134,7.48057270114217));
#8169=CARTESIAN_POINT('Ctrl Pts',(-5.52582819395051,-2.61991851823695,7.48804904635748));
#8170=CARTESIAN_POINT('Ctrl Pts',(-5.45349612724275,-2.76732987301179,7.49552539157279));
#8171=CARTESIAN_POINT('Ctrl Pts',(-5.37536853871852,-2.91156978886907,7.5030017367881));
#8172=CARTESIAN_POINT('Ctrl Pts',(-5.29464500099184,-3.06060237146041,7.51072649889129));
#8173=CARTESIAN_POINT('Ctrl Pts',(-5.20770543635674,-3.20630217515723,7.51845126099449));
#8174=CARTESIAN_POINT('Ctrl Pts',(-5.11485012499966,-3.34815378399662,7.52617602309768));
#8175=CARTESIAN_POINT('Ctrl Pts',(-5.02201292681427,-3.4899777220167,7.533899278341));
#8176=CARTESIAN_POINT('Ctrl Pts',(-4.92326245797659,-3.62795469801437,7.54162253358432));
#8177=CARTESIAN_POINT('Ctrl Pts',(-4.8189428629313,-3.76159743278086,7.54934578882765));
#8178=CARTESIAN_POINT('Ctrl Pts',(-4.71461923643464,-3.89524533219723,7.5570693425377));
#8179=CARTESIAN_POINT('Ctrl Pts',(-4.60472624494501,-4.02455840295248,7.56479289624775));
#8180=CARTESIAN_POINT('Ctrl Pts',(-4.48964942152743,-4.14908105901516,7.5725164499578));
#8181=CARTESIAN_POINT('Ctrl Pts',(-4.37458032719155,-4.27359535157116,7.58023948491894));
#8182=CARTESIAN_POINT('Ctrl Pts',(-4.254328312797,-4.39331964052788,7.58796251988007));
#8183=CARTESIAN_POINT('Ctrl Pts',(-4.12931711911013,-4.50783381374291,7.59568555484121));
#8184=CARTESIAN_POINT('Ctrl Pts',(-4.00427270289438,-4.62237841983613,7.60341064224856));
#8185=CARTESIAN_POINT('Ctrl Pts',(-3.87446681243393,-4.73170992754462,7.61113572965592));
#8186=CARTESIAN_POINT('Ctrl Pts',(-3.74035845520799,-4.83544663801123,7.61886081706327));
#8187=CARTESIAN_POINT('Ctrl Pts',(-3.60677012518912,-4.93878109232519,7.62655594917394));
#8188=CARTESIAN_POINT('Ctrl Pts',(-3.46891290279384,-5.03656389624701,7.63425108128461));
#8189=CARTESIAN_POINT('Ctrl Pts',(-3.3272712997932,-5.12845895567786,7.64194621339527));
#8190=CARTESIAN_POINT('Ctrl Pts',(-3.18508430789232,-5.22070785567773,7.64967097549847));
#8191=CARTESIAN_POINT('Ctrl Pts',(-3.03903335938653,-5.30705622646052,7.65739573760167));
#8192=CARTESIAN_POINT('Ctrl Pts',(-2.88962872821693,-5.38719513063741,7.66512049970487));
#8193=CARTESIAN_POINT('Ctrl Pts',(-2.74025324122563,-5.46731840221647,7.6728437549482));
#8194=CARTESIAN_POINT('Ctrl Pts',(-2.58752565604764,-5.54123447439842,7.68056701019152));
#8195=CARTESIAN_POINT('Ctrl Pts',(-2.43198130352822,-5.60868010335669,7.68829026543485));
#8196=CARTESIAN_POINT('Ctrl Pts',(-2.27643093996662,-5.67612833876459,7.69601381914489));
#8197=CARTESIAN_POINT('Ctrl Pts',(-2.11806388042359,-5.73710550086938,7.70373737285494));
#8198=CARTESIAN_POINT('Ctrl Pts',(-1.95743663722948,-5.79139597797731,7.71146092656498));
#8199=CARTESIAN_POINT('Ctrl Pts',(-1.79682018249013,-5.84568280869036,7.7191839615261));
#8200=CARTESIAN_POINT('Ctrl Pts',(-1.63394414815684,-5.89328375166325,7.72690699648723));
#8201=CARTESIAN_POINT('Ctrl Pts',(-1.46938162599392,-5.93403262543201,7.73463003144835));
#8202=CARTESIAN_POINT('Ctrl Pts',(-1.30477537028179,-5.97479232847618,7.74235511885571));
#8203=CARTESIAN_POINT('Ctrl Pts',(-1.13848203846609,-6.00869624520714,7.75008020626306));
#8204=CARTESIAN_POINT('Ctrl Pts',(-0.971087312893186,-6.0356287984963,7.75780529367042));
#8205=CARTESIAN_POINT('Ctrl Pts',(-0.804341687893734,-6.06245691638151,
7.76550042578111));
#8206=CARTESIAN_POINT('Ctrl Pts',(-0.636503508969812,-6.08236762216965,
7.77319555789179));
#8207=CARTESIAN_POINT('Ctrl Pts',(-0.46815903580214,-6.09529758746009,7.78089069000247));
#8208=CARTESIAN_POINT('Ctrl Pts',(-0.29916635472732,-6.10827733939089,7.78861545210568));
#8209=CARTESIAN_POINT('Ctrl Pts',(-0.129603618233078,-6.1142270527368,7.79634021420888));
#8210=CARTESIAN_POINT('Ctrl Pts',(0.0399332841301361,-6.11311957148873,
7.80406497631209));
#8211=CARTESIAN_POINT('Ctrl Pts',(0.209437115137693,-6.11201230627567,7.81178823155542));
#8212=CARTESIAN_POINT('Ctrl Pts',(0.378914805342489,-6.10385059542405,7.81951148679875));
#8213=CARTESIAN_POINT('Ctrl Pts',(0.54777032320894,-6.08865939559043,7.82723474204209));
#8214=CARTESIAN_POINT('Ctrl Pts',(0.716632366530116,-6.07346760868989,7.83495829575214));
#8215=CARTESIAN_POINT('Ctrl Pts',(0.884871873401426,-6.05124581365886,7.84268184946219));
#8216=CARTESIAN_POINT('Ctrl Pts',(1.05189700087771,-6.02207092801509,7.85040540317224));
#8217=CARTESIAN_POINT('Ctrl Pts',(1.21891091018829,-5.99289800188906,7.85812843813337));
#8218=CARTESIAN_POINT('Ctrl Pts',(1.3847102910964,-5.95677297424082,7.86585147309449));
#8219=CARTESIAN_POINT('Ctrl Pts',(1.54871239069064,-5.91382410064937,7.87357450805561));
#8220=CARTESIAN_POINT('Ctrl Pts',(1.71275807489821,-5.87086381311838,7.88129959546298));
#8221=CARTESIAN_POINT('Ctrl Pts',(1.87500521599692,-5.82107613410619,7.88902468287035));
#8222=CARTESIAN_POINT('Ctrl Pts',(2.03488421555061,-5.76463977988243,7.89674977027771));
#8223=CARTESIAN_POINT('Ctrl Pts',(2.19414325799339,-5.70842226690244,7.90444490238836));
#8224=CARTESIAN_POINT('Ctrl Pts',(2.35105220830446,-5.64560768402968,7.91214003449901));
#8225=CARTESIAN_POINT('Ctrl Pts',(2.50506595839486,-5.57642090471937,7.91983516660965));
#8226=CARTESIAN_POINT('Ctrl Pts',(2.65967203777948,-5.50696803646484,7.92755989381924));
#8227=CARTESIAN_POINT('Ctrl Pts',(2.8114153475298,-5.43106923489391,7.93528462102883));
#8228=CARTESIAN_POINT('Ctrl Pts',(2.9597596364623,-5.34898574094833,7.94300934823842));
#8229=CARTESIAN_POINT('Ctrl Pts',(3.10808411080891,-5.2669132110274,7.95073304364374));
#8230=CARTESIAN_POINT('Ctrl Pts',(3.25301019191251,-5.17865778836112,7.95845673904906));
#8231=CARTESIAN_POINT('Ctrl Pts',(3.39402634211527,-5.084526600533,7.96618043445437));
#8232=CARTESIAN_POINT('Ctrl Pts',(3.50621497110141,-5.00963837750259,7.97232519728461));
#8233=CARTESIAN_POINT('Ctrl Pts',(3.61592928983639,-4.93103209513385,7.97846996011485));
#8234=CARTESIAN_POINT('Ctrl Pts',(3.72292453512037,-4.84888218750454,7.98461472294509));
#8235=CARTESIAN_POINT('Ctrl Pts',(3.72292453512037,-4.84888218750454,6.23460979329304));
#8236=CARTESIAN_POINT('Ctrl Pts',(3.82674007619718,-4.76917362580806,6.24057367796984));
#8237=CARTESIAN_POINT('Ctrl Pts',(3.92798420304844,-4.68613792056754,6.24653756264663));
#8238=CARTESIAN_POINT('Ctrl Pts',(4.02644658881525,-4.59995145951759,6.25250144732343));
#8239=CARTESIAN_POINT('Ctrl Pts',(4.15398066222203,-4.4883178609143,6.26022620942661));
#8240=CARTESIAN_POINT('Ctrl Pts',(4.27689188120749,-4.37135738492506,6.26795097152978));
#8241=CARTESIAN_POINT('Ctrl Pts',(4.3947438398315,-4.24947669069534,6.27567573363296));
#8242=CARTESIAN_POINT('Ctrl Pts',(4.51257280921926,-4.12761977158237,6.28339898887632));
#8243=CARTESIAN_POINT('Ctrl Pts',(4.62534426730198,-4.00084477703188,6.29112224411968));
#8244=CARTESIAN_POINT('Ctrl Pts',(4.73265893453336,-3.86959493640893,6.29884549936304));
#8245=CARTESIAN_POINT('Ctrl Pts',(4.83997774896067,-3.73834002361067,6.30656905307308));
#8246=CARTESIAN_POINT('Ctrl Pts',(4.94183914688451,-3.60261016153296,6.31429260678313));
#8247=CARTESIAN_POINT('Ctrl Pts',(5.03788389727962,-3.46288195005702,6.32201616049317));
#8248=CARTESIAN_POINT('Ctrl Pts',(5.13392219687341,-3.3231631233619,6.32973919545429));
#8249=CARTESIAN_POINT('Ctrl Pts',(5.22414445120127,-3.17944674588159,6.33746223041541));
#8250=CARTESIAN_POINT('Ctrl Pts',(5.30823446293605,-3.03223885091495,6.34518526537653));
#8251=CARTESIAN_POINT('Ctrl Pts',(5.39234682213254,-2.88499183450299,6.35291035278389));
#8252=CARTESIAN_POINT('Ctrl Pts',(5.47032352303129,-2.73425172075412,6.36063544019125));
#8253=CARTESIAN_POINT('Ctrl Pts',(5.54189361959266,-2.58055045903353,6.36836052759861));
#8254=CARTESIAN_POINT('Ctrl Pts',(5.61318619133598,-2.42744519922915,6.37605565970927));
#8255=CARTESIAN_POINT('Ctrl Pts',(5.67812165318492,-2.27140201192588,6.38375079181993));
#8256=CARTESIAN_POINT('Ctrl Pts',(5.73647916917479,-2.11296765335481,6.39144592393059));
#8257=CARTESIAN_POINT('Ctrl Pts',(5.79506138991806,-1.95392324562609,6.39917068603379));
#8258=CARTESIAN_POINT('Ctrl Pts',(5.84703562758219,-1.79241287656113,6.40689544813698));
#8259=CARTESIAN_POINT('Ctrl Pts',(5.89221322034706,-1.62900243353636,6.41462021024018));
#8260=CARTESIAN_POINT('Ctrl Pts',(5.93738200037424,-1.46562386678653,6.4223434654835));
#8261=CARTESIAN_POINT('Ctrl Pts',(5.97575669657398,-1.30034627092843,6.43006672072682));
#8262=CARTESIAN_POINT('Ctrl Pts',(6.00719874504435,-1.13374988425033,6.43778997597013));
#8263=CARTESIAN_POINT('Ctrl Pts',(6.03864200859886,-0.967147059422086,6.44551352968017));
#8264=CARTESIAN_POINT('Ctrl Pts',(6.06315202564524,-0.799225652475361,6.4532370833902));
#8265=CARTESIAN_POINT('Ctrl Pts',(6.08064136536425,-0.630576044836139,6.46096063710024));
#8266=CARTESIAN_POINT('Ctrl Pts',(6.09812953041987,-0.461937764469577,6.46868367206137));
#8267=CARTESIAN_POINT('Ctrl Pts',(6.10859792909061,-0.292571696553318,6.47640670702251));
#8268=CARTESIAN_POINT('Ctrl Pts',(6.11201100137875,-0.123073480186015,6.48412974198364));
#8269=CARTESIAN_POINT('Ctrl Pts',(6.11542498071282,0.0464697814227938,6.491854829391));
#8270=CARTESIAN_POINT('Ctrl Pts',(6.11177987839815,0.216144944617681,6.49957991679836));
#8271=CARTESIAN_POINT('Ctrl Pts',(6.10109226977798,0.385355262265019,6.50730500420572));
#8272=CARTESIAN_POINT('Ctrl Pts',(6.09044610411762,0.553909439082053,6.51500013631641));
#8273=CARTESIAN_POINT('Ctrl Pts',(6.07281200386748,0.722002059437204,6.52269526842709));
#8274=CARTESIAN_POINT('Ctrl Pts',(6.04825763137341,0.889047348026707,6.53039040053778));
#8275=CARTESIAN_POINT('Ctrl Pts',(6.02360871263081,1.05673584203206,6.53811516264098));
#8276=CARTESIAN_POINT('Ctrl Pts',(5.99197736342121,1.22342830869872,6.54583992474417));
#8277=CARTESIAN_POINT('Ctrl Pts',(5.95346865194615,1.38853756621652,6.55356468684737));
#8278=CARTESIAN_POINT('Ctrl Pts',(5.91496745231817,1.55361461607414,6.5612879420907));
#8279=CARTESIAN_POINT('Ctrl Pts',(5.86959163925624,1.71710876456313,6.56901119733403));
#8280=CARTESIAN_POINT('Ctrl Pts',(5.81749713914765,1.87844419627224,6.57673445257736));
#8281=CARTESIAN_POINT('Ctrl Pts',(5.76540062583691,2.03978586282069,6.58445800628741));
#8282=CARTESIAN_POINT('Ctrl Pts',(5.70658499952515,2.19896834284973,6.59218155999745));
#8283=CARTESIAN_POINT('Ctrl Pts',(5.64125594066812,2.35543137755629,6.59990511370749));
#8284=CARTESIAN_POINT('Ctrl Pts',(5.57593126960733,2.51188390349494,6.6076281486686));
#8285=CARTESIAN_POINT('Ctrl Pts',(5.50409416358331,2.66561705714119,6.6153511836297));
#8286=CARTESIAN_POINT('Ctrl Pts',(5.42599836759865,2.81609077931035,6.6230742185908));
#8287=CARTESIAN_POINT('Ctrl Pts',(5.34788181715341,2.96660449083996,6.63079930599817));
#8288=CARTESIAN_POINT('Ctrl Pts',(5.26350339725766,3.11385675748476,6.63852439340554));
#8289=CARTESIAN_POINT('Ctrl Pts',(5.17316316443419,3.25733149013748,6.64624948081291));
#8290=CARTESIAN_POINT('Ctrl Pts',(5.08317324071836,3.40024987592243,6.6539446129236));
#8291=CARTESIAN_POINT('Ctrl Pts',(4.98726785132823,3.53941972465211,6.66163974503429));
#8292=CARTESIAN_POINT('Ctrl Pts',(4.88578666437294,3.67435902338564,6.66933487714498));
#8293=CARTESIAN_POINT('Ctrl Pts',(4.7839147256064,3.80981790389558,6.67705963924818));
#8294=CARTESIAN_POINT('Ctrl Pts',(4.67638786097806,3.94106154785416,6.68478440135139));
#8295=CARTESIAN_POINT('Ctrl Pts',(4.56357925856923,4.06762460328589,6.6925091634546));
#8296=CARTESIAN_POINT('Ctrl Pts',(4.450792661597,4.19416297021663,6.70023241869788));
#8297=CARTESIAN_POINT('Ctrl Pts',(4.332726593414,4.31602233401184,6.70795567394115));
#8298=CARTESIAN_POINT('Ctrl Pts',(4.20979346398447,4.43277165587104,6.71567892918443));
#8299=CARTESIAN_POINT('Ctrl Pts',(4.08685558377908,4.54952548953158,6.72340248289448));
#8300=CARTESIAN_POINT('Ctrl Pts',(3.95905049302257,4.66116866497647,6.73112603660453));
#8301=CARTESIAN_POINT('Ctrl Pts',(3.82682684928917,4.76730760787045,6.73884959031458));
#8302=CARTESIAN_POINT('Ctrl Pts',(3.69461208629594,4.87343942199119,6.7465726252757));
#8303=CARTESIAN_POINT('Ctrl Pts',(3.55797961138892,4.97406754496306,6.75429566023682));
#8304=CARTESIAN_POINT('Ctrl Pts',(3.41741062478746,5.06883913574793,6.76201869519794));
#8305=CARTESIAN_POINT('Ctrl Pts',(3.27680428107322,5.16363591269292,6.76974378260531));
#8306=CARTESIAN_POINT('Ctrl Pts',(3.13225959694467,5.25257286826412,6.77746887001267));
#8307=CARTESIAN_POINT('Ctrl Pts',(2.98428697198997,5.33534036695982,6.78519395742003));
#8308=CARTESIAN_POINT('Ctrl Pts',(2.83688813521952,5.41778692106995,6.79288908953074));
#8309=CARTESIAN_POINT('Ctrl Pts',(2.6860881833734,5.49411165515322,6.80058422164145));
#8310=CARTESIAN_POINT('Ctrl Pts',(2.53241599697323,5.56405380822059,6.80827935375216));
#8311=CARTESIAN_POINT('Ctrl Pts',(2.37815209809004,5.63426527251486,6.81600411585536));
#8312=CARTESIAN_POINT('Ctrl Pts',(2.22093915363002,5.69806974563762,6.82372887795856));
#8313=CARTESIAN_POINT('Ctrl Pts',(2.0613275077843,5.75523713396344,6.83145364006176));
#8314=CARTESIAN_POINT('Ctrl Pts',(1.90174699718607,5.81239337071713,6.83917689530511));
#8315=CARTESIAN_POINT('Ctrl Pts',(1.73976901703855,5.8629149992405,6.84690015054846));
#8316=CARTESIAN_POINT('Ctrl Pts',(1.57596193686568,5.90662082209875,6.85462340579181));
#8317=CARTESIAN_POINT('Ctrl Pts',(1.41214852633633,5.95032833397704,6.86234695950187));
#8318=CARTESIAN_POINT('Ctrl Pts',(1.24650617951962,5.98721942758742,6.87007051321192));
#8319=CARTESIAN_POINT('Ctrl Pts',(1.07961717181621,6.01716314593676,6.87779406692198));
#8320=CARTESIAN_POINT('Ctrl Pts',(0.912739373136056,6.04710485313007,6.88551710188311));
#8321=CARTESIAN_POINT('Ctrl Pts',(0.744615393106126,6.07010006287075,6.89324013684424));
#8322=CARTESIAN_POINT('Ctrl Pts',(0.575836595672656,6.08606915649043,6.90096317180537));
#8323=CARTESIAN_POINT('Ctrl Pts',(0.407012944188079,6.10204249399946,6.90868825921272));
#8324=CARTESIAN_POINT('Ctrl Pts',(0.237534443096473,6.11098595215364,6.91641334662007));
#8325=CARTESIAN_POINT('Ctrl Pts',(0.0679974262798713,6.11287182202599,6.92413843402742));
#8326=CARTESIAN_POINT('Ctrl Pts',(-0.100882182876039,6.1147503791278,6.93183356613806));
#8327=CARTESIAN_POINT('Ctrl Pts',(-0.26981954222674,6.10962601333181,6.93952869824871));
#8328=CARTESIAN_POINT('Ctrl Pts',(-0.438225472296301,6.09752277551554,6.94722383035936));
#8329=CARTESIAN_POINT('Ctrl Pts',(-0.607279846912093,6.08537293436082,6.95494859246253));
#8330=CARTESIAN_POINT('Ctrl Pts',(-0.775858563478678,6.06618603735116,6.96267335456571));
#8331=CARTESIAN_POINT('Ctrl Pts',(-0.94336826687528,6.04002333402386,6.97039811666888));
#8332=CARTESIAN_POINT('Ctrl Pts',(-1.11084529436024,6.01386573422289,6.97812137191222));
#8333=CARTESIAN_POINT('Ctrl Pts',(-1.27725341182941,5.98073509218863,6.98584462715556));
#8334=CARTESIAN_POINT('Ctrl Pts',(-1.44200682901433,5.94074421832619,6.9935678823989));
#8335=CARTESIAN_POINT('Ctrl Pts',(-1.60676661312709,5.90075179900865,7.00129143610895));
#8336=CARTESIAN_POINT('Ctrl Pts',(-1.7698712600859,5.85389868825748,7.00901498981898));
#8337=CARTESIAN_POINT('Ctrl Pts',(-1.93074680500557,5.80034846689927,7.01673854352903));
#8338=CARTESIAN_POINT('Ctrl Pts',(-2.09161154479325,5.74680184221706,7.02446157849013));
#8339=CARTESIAN_POINT('Ctrl Pts',(-2.25024718141715,5.6865591071788,7.03218461345124));
#8340=CARTESIAN_POINT('Ctrl Pts',(-2.40609633085892,5.61983327236024,7.03990764841235));
#8341=CARTESIAN_POINT('Ctrl Pts',(-2.56198689821528,5.5530897047216,7.04763273581971));
#8342=CARTESIAN_POINT('Ctrl Pts',(-2.71508920622712,5.47985971730165,7.05535782322707));
#8343=CARTESIAN_POINT('Ctrl Pts',(-2.86486634178415,5.40040428173783,7.06308291063443));
#8344=CARTESIAN_POINT('Ctrl Pts',(-3.01406269187019,5.32125694769028,7.07077804274513));
#8345=CARTESIAN_POINT('Ctrl Pts',(-3.15995935078779,5.2359325348516,7.07847317485582));
#8346=CARTESIAN_POINT('Ctrl Pts',(-3.30205045130174,5.14473404361761,7.08616830696652));
#8347=CARTESIAN_POINT('Ctrl Pts',(-3.44468867149895,5.0531843939405,7.09389306906973));
#8348=CARTESIAN_POINT('Ctrl Pts',(-3.58354247061905,4.95568289053558,7.10161783117293));
#8349=CARTESIAN_POINT('Ctrl Pts',(-3.71812011161081,4.85256719666356,7.10934259327613));
#8350=CARTESIAN_POINT('Ctrl Pts',(-3.85267150070687,4.74947161744372,7.11706584851944));
#8351=CARTESIAN_POINT('Ctrl Pts',(-3.98294814467582,4.64076422561949,7.12478910376276));
#8352=CARTESIAN_POINT('Ctrl Pts',(-4.10848961758786,4.526824342149,7.13251235900607));
#8353=CARTESIAN_POINT('Ctrl Pts',(-4.23403594207518,4.41288005544898,7.14023591271613));
#8354=CARTESIAN_POINT('Ctrl Pts',(-4.35484649199016,4.29370308252234,7.14795946642618));
#8355=CARTESIAN_POINT('Ctrl Pts',(-4.47049551563522,4.16971166955048,7.15568302013624));
#8356=CARTESIAN_POINT('Ctrl Pts',(-4.58613677176657,4.04572858440508,7.16340605509734));
#8357=CARTESIAN_POINT('Ctrl Pts',(-4.69661697918975,3.91693193809907,7.17112909005845));
#8358=CARTESIAN_POINT('Ctrl Pts',(-4.80154859493683,3.78377544959531,7.17885212501956));
#8359=CARTESIAN_POINT('Ctrl Pts',(-4.90650809693604,3.65058357389785,7.1865772124269));
#8360=CARTESIAN_POINT('Ctrl Pts',(-5.0059158626915,3.51302978847744,7.19430229983425));
#8361=CARTESIAN_POINT('Ctrl Pts',(-5.09942527124864,3.37160013427611,7.20202738724159));
#8362=CARTESIAN_POINT('Ctrl Pts',(-5.19257208169858,3.23071889681388,7.2097225193523));
#8363=CARTESIAN_POINT('Ctrl Pts',(-5.27986605204589,3.08599207396941,7.21741765146301));
#8364=CARTESIAN_POINT('Ctrl Pts',(-5.36100793131647,2.93792775998013,7.22511278357372));
#8365=CARTESIAN_POINT('Ctrl Pts',(-5.44246224619427,2.78929332653756,7.23283754567692));
#8366=CARTESIAN_POINT('Ctrl Pts',(-5.51774582123992,2.63724299268517,7.24056230778012));
#8367=CARTESIAN_POINT('Ctrl Pts',(-5.58658839729109,2.48230853073357,7.24828706988332));
#8368=CARTESIAN_POINT('Ctrl Pts',(-5.65541754430528,2.32740429165766,7.25601032512664));
#8369=CARTESIAN_POINT('Ctrl Pts',(-5.71780807075731,2.16961733652475,7.26373358036996));
#8370=CARTESIAN_POINT('Ctrl Pts',(-5.77353714285875,2.00950103820087,7.27145683561328));
#8371=CARTESIAN_POINT('Ctrl Pts',(-5.82926836862119,1.84937855215102,7.27918038932332));
#8372=CARTESIAN_POINT('Ctrl Pts',(-5.87833751697747,1.68692684078353,7.28690394303336));
#8373=CARTESIAN_POINT('Ctrl Pts',(-5.92057082545285,1.52271686905236,7.29462749674341));
#8374=CARTESIAN_POINT('Ctrl Pts',(-5.96280129734756,1.3585179264081,7.30235053170453));
#8375=CARTESIAN_POINT('Ctrl Pts',(-5.99819676920487,1.19256126669211,7.31007356666565));
#8376=CARTESIAN_POINT('Ctrl Pts',(-6.02663400184908,1.02543072426009,7.31779660162678));
#8377=CARTESIAN_POINT('Ctrl Pts',(-6.05507879187085,0.85825576581093,7.32552168903414));
#8378=CARTESIAN_POINT('Ctrl Pts',(-6.07656159218805,0.689906613550995,7.33324677644151));
#8379=CARTESIAN_POINT('Ctrl Pts',(-6.09101056209332,0.520975906321606,7.34097186384887));
#8380=CARTESIAN_POINT('Ctrl Pts',(-6.10540350374189,0.352700255687394,7.34866699595955));
#8381=CARTESIAN_POINT('Ctrl Pts',(-6.11281707319215,0.183847866016913,7.35636212807023));
#8382=CARTESIAN_POINT('Ctrl Pts',(-6.11323157749471,0.0150080785417984,
7.3640572601809));
#8383=CARTESIAN_POINT('Ctrl Pts',(-6.11324385480432,0.0100071694253899,
7.36428518427924));
#8384=CARTESIAN_POINT('Ctrl Pts',(-6.11324999564585,0.0050062452407887,
7.36451310837758));
#8385=CARTESIAN_POINT('Ctrl Pts',(-6.11324999999769,5.31978972713177E-6,
7.36474103247592));
#8386=CARTESIAN_POINT('Origin',(0.,0.,-3.86474103256053));
#8387=CARTESIAN_POINT('',(3.72292453512037,-4.84888218750453,4.4846183003358));
#8388=CARTESIAN_POINT('',(3.72292453512038,-4.84888218750453,4.63013458917765));
#8389=CARTESIAN_POINT('',(3.72292453512038,-4.84888218750453,-3.86474103256053));
#8390=CARTESIAN_POINT('',(-6.11319920576163,-1.41071580853158E-5,5.76025896758647));
#8391=CARTESIAN_POINT('Ctrl Pts',(3.72292453512038,-4.84888218750453,4.63013458917765));
#8392=CARTESIAN_POINT('Ctrl Pts',(3.85740293170725,-4.74563098387927,4.63785792890056));
#8393=CARTESIAN_POINT('Ctrl Pts',(3.98758890164652,-4.6367776533406,4.64558126862347));
#8394=CARTESIAN_POINT('Ctrl Pts',(4.11302426972855,-4.52270460224011,4.65330460834637));
#8395=CARTESIAN_POINT('Ctrl Pts',(4.23845419774736,-4.40863649842539,4.66102761311227));
#8396=CARTESIAN_POINT('Ctrl Pts',(4.35913370250064,-4.28934934113618,4.66875061787816));
#8397=CARTESIAN_POINT('Ctrl Pts',(4.47463982938566,-4.16526397240024,4.67647362264406));
#8398=CARTESIAN_POINT('Ctrl Pts',(4.59017383948617,-4.04114864941713,4.68419849174574));
#8399=CARTESIAN_POINT('Ctrl Pts',(4.70053175983779,-3.91223303220383,4.69192336084742));
#8400=CARTESIAN_POINT('Ctrl Pts',(4.80532886836392,-3.77897340945505,4.6996482299491));
#8401=CARTESIAN_POINT('Ctrl Pts',(4.87975910829058,-3.68432818657416,4.70513467770254));
#8402=CARTESIAN_POINT('Ctrl Pts',(4.95138511255325,-3.5874924626389,4.71062112545598));
#8403=CARTESIAN_POINT('Ctrl Pts',(5.02008170643796,-3.48863945158953,4.71610757320942));
#8404=CARTESIAN_POINT('Ctrl Pts',(5.11680455315176,-3.34945722880027,4.72383233531262));
#8405=CARTESIAN_POINT('Ctrl Pts',(5.20775270115482,-3.20622540597074,4.73155709741581));
#8406=CARTESIAN_POINT('Ctrl Pts',(5.29260114598734,-3.05944417696965,4.73928185951901));
#8407=CARTESIAN_POINT('Ctrl Pts',(5.3774330395378,-2.91269158040286,4.74700511476234));
#8408=CARTESIAN_POINT('Ctrl Pts',(5.45616744560474,-2.76239123342247,4.75472837000567));
#8409=CARTESIAN_POINT('Ctrl Pts',(5.52852423355157,-2.60906982687951,4.76245162524899));
#8410=CARTESIAN_POINT('Ctrl Pts',(5.60088381774069,-2.45574249520064,4.77017517895904));
#8411=CARTESIAN_POINT('Ctrl Pts',(5.66686515178002,-2.29939415525088,4.77789873266908));
#8412=CARTESIAN_POINT('Ctrl Pts',(5.72623503965873,-2.14057418303701,4.78562228637913));
#8413=CARTESIAN_POINT('Ctrl Pts',(5.78560093998629,-1.98176487789336,4.79334532134025));
#8414=CARTESIAN_POINT('Ctrl Pts',(5.83835617180195,-1.82048456958474,4.80106835630137));
#8415=CARTESIAN_POINT('Ctrl Pts',(5.8843164172226,-1.65730077671634,4.80879139126249));
#8416=CARTESIAN_POINT('Ctrl Pts',(5.93028887687421,-1.49407361670494,4.81651647866985));
#8417=CARTESIAN_POINT('Ctrl Pts',(5.96946265360397,-1.32894226597837,4.82424156607721));
#8418=CARTESIAN_POINT('Ctrl Pts',(6.00170360798695,-1.16248843623341,4.83196665348456));
#8419=CARTESIAN_POINT('Ctrl Pts',(6.03381954276788,-0.996680058583567,4.83966178559525));
#8420=CARTESIAN_POINT('Ctrl Pts',(6.05905629822593,-0.82955975256591,4.84735691770593));
#8421=CARTESIAN_POINT('Ctrl Pts',(6.07733193889542,-0.661711468074713,4.85505204981662));
#8422=CARTESIAN_POINT('Ctrl Pts',(6.09567794964934,-0.493216886243646,4.86277681191982));
#8423=CARTESIAN_POINT('Ctrl Pts',(6.10701559962199,-0.32392902965204,4.87050157402302));
#8424=CARTESIAN_POINT('Ctrl Pts',(6.11129880128841,-0.154442623232287,4.87822633612622));
#8425=CARTESIAN_POINT('Ctrl Pts',(6.11558116743593,0.0150107216820271,4.88594959136955));
#8426=CARTESIAN_POINT('Ctrl Pts',(6.11281182309288,0.18466222250966,4.89367284661288));
#8427=CARTESIAN_POINT('Ctrl Pts',(6.10299676254115,0.353915355575724,4.90139610185621));
#8428=CARTESIAN_POINT('Ctrl Pts',(6.09318132268446,0.52317502946243,4.90911965556626));
#8429=CARTESIAN_POINT('Ctrl Pts',(6.07631963615679,0.692035988165516,4.91684320927631));
#8430=CARTESIAN_POINT('Ctrl Pts',(6.05246976500209,0.85990424248026,4.92456676298636));
#8431=CARTESIAN_POINT('Ctrl Pts',(6.02862149571299,1.0277612220011,4.93228979794748));
#8432=CARTESIAN_POINT('Ctrl Pts',(5.99778602564995,1.19462531675511,4.94001283290861));
#8433=CARTESIAN_POINT('Ctrl Pts',(5.96007301796655,1.35990999077407,4.94773586786973));
#8434=CARTESIAN_POINT('Ctrl Pts',(5.92234998780869,1.52523859025868,4.95546095527709));
#8435=CARTESIAN_POINT('Ctrl Pts',(5.87774583616835,1.68898662057517,4.96318604268445));
#8436=CARTESIAN_POINT('Ctrl Pts',(5.82642107960329,1.85057908927299,4.97091113009181));
#8437=CARTESIAN_POINT('Ctrl Pts',(5.77529534322139,2.011544956602,4.97860626220248));
#8438=CARTESIAN_POINT('Ctrl Pts',(5.71750115499425,2.17037166190213,4.98630139431314));
#8439=CARTESIAN_POINT('Ctrl Pts',(5.65324594395815,2.32650722320407,4.99399652642381));
#8440=CARTESIAN_POINT('Ctrl Pts',(5.588743319181,2.48324398217871,5.00172128852701));
#8441=CARTESIAN_POINT('Ctrl Pts',(5.51770694400194,2.63732433166466,5.00944605063021));
#8442=CARTESIAN_POINT('Ctrl Pts',(5.44038088156317,2.78820397855356,5.01717081273341));
#8443=CARTESIAN_POINT('Ctrl Pts',(5.36306990302458,2.93905419353479,5.02489406797675));
#8444=CARTESIAN_POINT('Ctrl Pts',(5.27947182983405,3.08670466986316,5.03261732322008));
#8445=CARTESIAN_POINT('Ctrl Pts',(5.18987732009901,3.2306344523672,5.04034057846341));
#8446=CARTESIAN_POINT('Ctrl Pts',(5.10027934796653,3.37456979706599,5.04806413217346));
#8447=CARTESIAN_POINT('Ctrl Pts',(5.0046846396936,3.51478388907138,5.05578768588351));
#8448=CARTESIAN_POINT('Ctrl Pts',(4.90342836288413,3.65078290953645,5.06351123959356));
#8449=CARTESIAN_POINT('Ctrl Pts',(4.80217888690586,3.78677279568995,5.07123427455468));
#8450=CARTESIAN_POINT('Ctrl Pts',(4.69526879263646,3.91854792261217,5.0789573095158));
#8451=CARTESIAN_POINT('Ctrl Pts',(4.58307499411493,4.04564570381768,5.08668034447692));
#8452=CARTESIAN_POINT('Ctrl Pts',(4.47085137936944,4.17277726207644,5.09440543188428));
#8453=CARTESIAN_POINT('Ctrl Pts',(4.3533414627329,4.29522875152499,5.10213051929164));
#8454=CARTESIAN_POINT('Ctrl Pts',(4.23096129118955,4.41257205209792,5.10985560669901));
#8455=CARTESIAN_POINT('Ctrl Pts',(4.10905566888494,4.52946033472753,5.11755073880967));
#8456=CARTESIAN_POINT('Ctrl Pts',(3.98231774261072,4.64127978094795,5.12524587092034));
#8457=CARTESIAN_POINT('Ctrl Pts',(3.851193745536,4.74764492109977,5.132941003031));
#8458=CARTESIAN_POINT('Ctrl Pts',(3.7195648574473,4.85441961865268,5.1406657651342));
#8459=CARTESIAN_POINT('Ctrl Pts',(3.58346941655499,4.95573571640908,5.14839052723739));
#8460=CARTESIAN_POINT('Ctrl Pts',(3.44338214681699,5.05123202332679,5.15611528934059));
#8461=CARTESIAN_POINT('Ctrl Pts',(3.30332220373084,5.14670970189706,5.16383854458392));
#8462=CARTESIAN_POINT('Ctrl Pts',(3.15927224725646,5.23636967647257,5.17156179982725));
#8463=CARTESIAN_POINT('Ctrl Pts',(3.01173675205558,5.31989354205681,5.17928505507058));
#8464=CARTESIAN_POINT('Ctrl Pts',(2.86419555531649,5.40342063543725,5.18700860878062));
#8465=CARTESIAN_POINT('Ctrl Pts',(2.71316882414718,5.48081098573346,5.19473216249067));
#8466=CARTESIAN_POINT('Ctrl Pts',(2.55918713534885,5.55179131170877,5.20245571620071));
#8467=CARTESIAN_POINT('Ctrl Pts',(2.4052157886596,5.62276687032323,5.21017875116184));
#8468=CARTESIAN_POINT('Ctrl Pts',(2.24829016935885,5.6873331334887,5.21790178612296));
#8469=CARTESIAN_POINT('Ctrl Pts',(2.08896257040708,5.74526421863592,5.22562482108408));
#8470=CARTESIAN_POINT('Ctrl Pts',(1.92959262912074,5.80321069934176,5.23334990849144));
#8471=CARTESIAN_POINT('Ctrl Pts',(1.7678197299364,5.85451836802344,5.2410749958988));
#8472=CARTESIAN_POINT('Ctrl Pts',(1.60421403973201,5.89901033032039,5.24880008330615));
#8473=CARTESIAN_POINT('Ctrl Pts',(1.44124275749345,5.94332976771762,5.25649521541683));
#8474=CARTESIAN_POINT('Ctrl Pts',(1.27645318257264,5.9808862119964,5.26419034752751));
#8475=CARTESIAN_POINT('Ctrl Pts',(1.1104215839229,6.01155466318474,5.27188547963819));
#8476=CARTESIAN_POINT('Ctrl Pts',(0.943750683055199,6.04234120279134,5.27961024174139));
#8477=CARTESIAN_POINT('Ctrl Pts',(0.775769139355649,6.06619747392887,5.28733500384459));
#8478=CARTESIAN_POINT('Ctrl Pts',(0.607066624682404,6.08303342713952,5.29505976594779));
#8479=CARTESIAN_POINT('Ctrl Pts',(0.438397018601847,6.09986609618141,5.30278302119112));
#8480=CARTESIAN_POINT('Ctrl Pts',(0.269007037341032,6.10968114837651,5.31050627643444));
#8481=CARTESIAN_POINT('Ctrl Pts',(0.0994920075322081,6.11244033941741,5.31822953167777));
#8482=CARTESIAN_POINT('Ctrl Pts',(-0.0700295732183527,6.11519963708779,
5.32595308538781));
#8483=CARTESIAN_POINT('Ctrl Pts',(-0.239675895375619,6.11090251884586,5.33367663909786));
#8484=CARTESIAN_POINT('Ctrl Pts',(-0.408850299863663,6.0995628527626,5.34140019280791));
#8485=CARTESIAN_POINT('Ctrl Pts',(-0.578013341830746,6.08822394830279,5.34912322776903));
#8486=CARTESIAN_POINT('Ctrl Pts',(-0.746704213310474,6.06984346377552,5.35684626273015));
#8487=CARTESIAN_POINT('Ctrl Pts',(-0.914329862609266,6.04448727890471,5.36456929769127));
#8488=CARTESIAN_POINT('Ctrl Pts',(-1.08200005950303,6.01912435546461,5.37229438509863));
#8489=CARTESIAN_POINT('Ctrl Pts',(-1.24860415462535,5.98678207254353,5.38001947250599));
#8490=CARTESIAN_POINT('Ctrl Pts',(-1.41355683812085,5.94757787909513,5.38774455991335));
#8491=CARTESIAN_POINT('Ctrl Pts',(-1.57786989046229,5.90852570635333,5.39543969202402));
#8492=CARTESIAN_POINT('Ctrl Pts',(-1.74054401937625,5.86266484840827,5.40313482413469));
#8493=CARTESIAN_POINT('Ctrl Pts',(-1.90101338440889,5.81016124344224,5.41082995624536));
#8494=CARTESIAN_POINT('Ctrl Pts',(-2.06210063436128,5.75745547412082,5.41855471834856));
#8495=CARTESIAN_POINT('Ctrl Pts',(-2.2210231508804,5.69803700527917,5.42627948045175));
#8496=CARTESIAN_POINT('Ctrl Pts',(-2.37722004541994,5.63210887840014,5.43400424255495));
#8497=CARTESIAN_POINT('Ctrl Pts',(-2.5333864708227,5.56619361204,5.44172749779827));
#8498=CARTESIAN_POINT('Ctrl Pts',(-2.68682804333982,5.49377134457642,5.44945075304159));
#8499=CARTESIAN_POINT('Ctrl Pts',(-2.83700369391927,5.4150933143565,5.45717400828491));
#8500=CARTESIAN_POINT('Ctrl Pts',(-2.98718514806639,5.33641224360856,5.46489756199496));
#8501=CARTESIAN_POINT('Ctrl Pts',(-3.13410014515453,5.25147506990209,5.47262111570501));
#8502=CARTESIAN_POINT('Ctrl Pts',(-3.27723137816399,5.16057943030406,5.48034466941505));
#8503=CARTESIAN_POINT('Ctrl Pts',(-3.42035299783036,5.06968989566964,5.48806770437618));
#8504=CARTESIAN_POINT('Ctrl Pts',(-3.55969109442315,4.97284286592676,5.49579073933731));
#8505=CARTESIAN_POINT('Ctrl Pts',(-3.69475641255519,4.87037992505537,5.50351377429844));
#8506=CARTESIAN_POINT('Ctrl Pts',(-3.82985762516441,4.76788975399828,5.5112388617058));
#8507=CARTESIAN_POINT('Ctrl Pts',(-3.96068353628313,4.65978087945045,5.51896394911315));
#8508=CARTESIAN_POINT('Ctrl Pts',(-4.0867763610621,4.54643646575689,5.52668903652051));
#8509=CARTESIAN_POINT('Ctrl Pts',(-4.21238024017934,4.43353156366484,5.53438416863119));
#8510=CARTESIAN_POINT('Ctrl Pts',(-4.3332874637223,4.31543188625376,5.54207930074187));
#8511=CARTESIAN_POINT('Ctrl Pts',(-4.44908054209656,4.19255386279506,5.54977443285255));
#8512=CARTESIAN_POINT('Ctrl Pts',(-4.56531948000866,4.06920269932213,5.55749919495576));
#8513=CARTESIAN_POINT('Ctrl Pts',(-4.67644595721203,3.94099261094878,5.56522395705897));
#8514=CARTESIAN_POINT('Ctrl Pts',(-4.7820645838156,3.80837023918585,5.57294871916217));
#8515=CARTESIAN_POINT('Ctrl Pts',(-4.887662607523,3.6757737379066,5.5806719744055));
#8516=CARTESIAN_POINT('Ctrl Pts',(-4.98775472714699,3.5387669184038,5.58839522964882));
#8517=CARTESIAN_POINT('Ctrl Pts',(-5.08198601560127,3.39782926288728,5.59611848489214));
#8518=CARTESIAN_POINT('Ctrl Pts',(-5.17622094564231,3.25688616080722,5.60384203860218));
#8519=CARTESIAN_POINT('Ctrl Pts',(-5.26459441184698,3.11201217999068,5.61156559231223));
#8520=CARTESIAN_POINT('Ctrl Pts',(-5.34679455169444,2.96371617812345,5.61928914602228));
#8521=CARTESIAN_POINT('Ctrl Pts',(-5.42898917060749,2.81543013648866,5.62701218098341));
#8522=CARTESIAN_POINT('Ctrl Pts',(-5.50501113924724,2.66372281096924,5.63473521594454));
#8523=CARTESIAN_POINT('Ctrl Pts',(-5.5745942534521,2.50912822946114,5.64245825090566));
#8524=CARTESIAN_POINT('Ctrl Pts',(-5.6441958598173,2.35449256344825,5.65018333831303));
#8525=CARTESIAN_POINT('Ctrl Pts',(-5.70735506026154,2.1969683964917,5.65790842572039));
#8526=CARTESIAN_POINT('Ctrl Pts',(-5.76385317898686,2.03711121286567,5.66563351312776));
#8527=CARTESIAN_POINT('Ctrl Pts',(-5.82013221696651,1.87787390175539,5.67332864523842));
#8528=CARTESIAN_POINT('Ctrl Pts',(-5.86980166664037,1.71632194021236,5.68102377734908));
#8529=CARTESIAN_POINT('Ctrl Pts',(-5.91269415143927,1.55302074488264,5.68871890945974));
#8530=CARTESIAN_POINT('Ctrl Pts',(-5.95622561344383,1.38728682172284,5.69652867736351));
#8531=CARTESIAN_POINT('Ctrl Pts',(-5.99279060141521,1.21969844586006,5.70433844526727));
#8532=CARTESIAN_POINT('Ctrl Pts',(-6.02225374567939,1.05084983948734,5.71214821317104));
#8533=CARTESIAN_POINT('Ctrl Pts',(-6.05250419851263,0.877489292587187,5.72016667221578));
#8534=CARTESIAN_POINT('Ctrl Pts',(-6.07526787912564,0.702800542431067,5.72818513126051));
#8535=CARTESIAN_POINT('Ctrl Pts',(-6.09045444039747,0.527437457849552,5.73620359030525));
#8536=CARTESIAN_POINT('Ctrl Pts',(-6.10564100166929,0.352074373268037,5.74422204934998));
#8537=CARTESIAN_POINT('Ctrl Pts',(-6.11325040615677,0.176037297326452,5.75224050839472));
#8538=CARTESIAN_POINT('Ctrl Pts',(-6.11324999998373,-1.4104047642468E-5,
5.76025896743945));
#8539=CARTESIAN_POINT('Ctrl Pts',(-6.11272873999193,-1.41359676000207E-5,
5.76025896894818));
#8540=CARTESIAN_POINT('Ctrl Pts',(-6.11276834790607,-0.493277251017307,
5.78272710798777));
#8541=CARTESIAN_POINT('Ctrl Pts',(-5.9321396680783,-2.00330256368141,5.85151007256308));
#8542=CARTESIAN_POINT('Ctrl Pts',(-4.70225644657925,-4.30111769607244,5.96660786267411));
#8543=CARTESIAN_POINT('Ctrl Pts',(-2.071393642429,-6.02662073661255,6.1055523392813));
#8544=CARTESIAN_POINT('Ctrl Pts',(1.03946149232852,-6.28111086285485,6.24339327091069));
#8545=CARTESIAN_POINT('Ctrl Pts',(2.93620164665179,-5.45327201018824,6.33491937700434));
#8546=CARTESIAN_POINT('Ctrl Pts',(3.72323907905155,-4.84929205898333,6.38013065756227));
#8547=CARTESIAN_POINT('',(-6.11324999945666,8.15052733732165E-5,5.61474103252431));
#8548=CARTESIAN_POINT('Ctrl Pts',(-6.11324999945667,8.15044776936738E-5,
5.61474103256055));
#8549=CARTESIAN_POINT('Ctrl Pts',(-6.11325227041943,-0.170252242020816,
5.62249939646803));
#8550=CARTESIAN_POINT('Ctrl Pts',(-6.10613117300444,-0.340583666322338,
5.63025776037552));
#8551=CARTESIAN_POINT('Ctrl Pts',(-6.09191333408529,-0.510311172221234,
5.638016124283));
#8552=CARTESIAN_POINT('Ctrl Pts',(-6.07769535203109,-0.680040386815467,
5.64577456629615));
#8553=CARTESIAN_POINT('Ctrl Pts',(-6.0563805151783,-0.849165361413687,5.6535330083093));
#8554=CARTESIAN_POINT('Ctrl Pts',(-6.02804736704293,-1.01708923069061,5.66129145032245));
#8555=CARTESIAN_POINT('Ctrl Pts',(-5.999707103126,-1.1850552735222,5.66905184084405));
#8556=CARTESIAN_POINT('Ctrl Pts',(-5.96434505832789,-1.35181930182925,5.67681223136565));
#8557=CARTESIAN_POINT('Ctrl Pts',(-5.9220911369778,-1.5167933701823,5.68457262188726));
#8558=CARTESIAN_POINT('Ctrl Pts',(-5.90003795229844,-1.60289670640407,5.68862292822306));
#8559=CARTESIAN_POINT('Ctrl Pts',(-5.87610825654539,-1.68851263893871,5.69267323455887));
#8560=CARTESIAN_POINT('Ctrl Pts',(-5.85032597278372,-1.77355901358603,5.69672354089467));
#8561=CARTESIAN_POINT('Ctrl Pts',(-5.80115388750823,-1.93575983431962,5.70444830299787));
#8562=CARTESIAN_POINT('Ctrl Pts',(-5.74522338914962,-2.09594316694078,5.71217306510106));
#8563=CARTESIAN_POINT('Ctrl Pts',(-5.68272521061636,-2.25354381877194,5.71989782720426));
#8564=CARTESIAN_POINT('Ctrl Pts',(-5.62023922352594,-2.41111372763774,5.72762108244762));
#8565=CARTESIAN_POINT('Ctrl Pts',(-5.55118822937105,-2.56610166654768,5.73534433769097));
#8566=CARTESIAN_POINT('Ctrl Pts',(-5.47581157962943,-2.71796120408226,5.74306759293432));
#8567=CARTESIAN_POINT('Ctrl Pts',(-5.40043201694254,-2.86982661025815,5.75079114664437));
#8568=CARTESIAN_POINT('Ctrl Pts',(-5.3187264468512,-3.01856308750147,5.75851470035443));
#8569=CARTESIAN_POINT('Ctrl Pts',(-5.23098112786476,-3.1636469465512,5.76623825406448));
#8570=CARTESIAN_POINT('Ctrl Pts',(-5.14324170225228,-3.30872106111031,5.7739612890256));
#8571=CARTESIAN_POINT('Ctrl Pts',(-5.04946350356382,-3.45014277720372,5.78168432398672));
#8572=CARTESIAN_POINT('Ctrl Pts',(-4.94997733988254,-3.5874154898965,5.78940735894785));
#8573=CARTESIAN_POINT('Ctrl Pts',(-4.85046473711304,-3.72472468369606,5.79713244635521));
#8574=CARTESIAN_POINT('Ctrl Pts',(-4.74524132250649,-3.8578824127043,5.80485753376257));
#8575=CARTESIAN_POINT('Ctrl Pts',(-4.63468016246876,-3.98642262612967,5.81258262116993));
#8576=CARTESIAN_POINT('Ctrl Pts',(-4.52454772150958,-4.11446440374052,5.82027775328057));
#8577=CARTESIAN_POINT('Ctrl Pts',(-4.40911908552082,-4.23792419680251,5.82797288539121));
#8578=CARTESIAN_POINT('Ctrl Pts',(-4.28880145867236,-4.35637551303717,5.83566801750185));
#8579=CARTESIAN_POINT('Ctrl Pts',(-4.16802055057835,-4.47528292431591,5.84339277960505));
#8580=CARTESIAN_POINT('Ctrl Pts',(-4.04227012884317,-4.58918530414057,5.85111754170825));
#8581=CARTESIAN_POINT('Ctrl Pts',(-3.91198808571947,-4.69767759426814,5.85884230381145));
#8582=CARTESIAN_POINT('Ctrl Pts',(-3.78173145655423,-4.80614872093766,5.86656555905478));
#8583=CARTESIAN_POINT('Ctrl Pts',(-3.64694521324448,-4.90921166100622,5.87428881429811));
#8584=CARTESIAN_POINT('Ctrl Pts',(-3.50810096534317,-5.00650109152673,5.88201206954143));
#8585=CARTESIAN_POINT('Ctrl Pts',(-3.3692513517786,-5.1037942818164,5.88973562325148));
#8586=CARTESIAN_POINT('Ctrl Pts',(-3.22634367708091,-5.19531333097637,5.89745917696152));
#8587=CARTESIAN_POINT('Ctrl Pts',(-3.07987986057829,-5.28073532823832,5.90518273067156));
#8588=CARTESIAN_POINT('Ctrl Pts',(-2.93342588125007,-5.36615158817138,5.9129057656327));
#8589=CARTESIAN_POINT('Ctrl Pts',(-2.7834165118849,-5.4454714560156,5.92062880059383));
#8590=CARTESIAN_POINT('Ctrl Pts',(-2.63037983402097,-5.51841711827548,5.92835183555497));
#8591=CARTESIAN_POINT('Ctrl Pts',(-2.47730248567556,-5.59138216631429,5.93607692296232));
#8592=CARTESIAN_POINT('Ctrl Pts',(-2.32119650654447,-5.65796948534384,5.94380201036967));
#8593=CARTESIAN_POINT('Ctrl Pts',(-2.16261246830647,-5.71794830987701,5.95152709777702));
#8594=CARTESIAN_POINT('Ctrl Pts',(-2.00464336575315,-5.77769455665558,5.95922222988769));
#8595=CARTESIAN_POINT('Ctrl Pts',(-1.8442156914994,-5.83088338859352,5.96691736199837));
#8596=CARTESIAN_POINT('Ctrl Pts',(-1.68189106853615,-5.87733511007143,5.97461249410904));
#8597=CARTESIAN_POINT('Ctrl Pts',(-1.51894141700973,-5.92396569321679,5.98233725621225));
#8598=CARTESIAN_POINT('Ctrl Pts',(-1.35402245925002,-5.96382366692076,5.99006201831545));
#8599=CARTESIAN_POINT('Ctrl Pts',(-1.18771251158513,-5.9967628394263,5.99778678041866));
#8600=CARTESIAN_POINT('Ctrl Pts',(-1.02143500579854,-6.0296955865277,6.00551003566196));
#8601=CARTESIAN_POINT('Ctrl Pts',(-0.853767362223276,-6.05571216391337,
6.01323329090526));
#8602=CARTESIAN_POINT('Ctrl Pts',(-0.685298494701385,-6.0747174037695,6.02095654614857));
#8603=CARTESIAN_POINT('Ctrl Pts',(-0.516823116666214,-6.09372337808694,
6.02868009985862));
#8604=CARTESIAN_POINT('Ctrl Pts',(-0.347546767200922,-6.10571743321528,
6.03640365356867));
#8605=CARTESIAN_POINT('Ctrl Pts',(-0.178064684725665,-6.11065614566501,
6.04412720727873));
#8606=CARTESIAN_POINT('Ctrl Pts',(-0.00859398543617382,-6.1155945264084,
6.05185024223987));
#8607=CARTESIAN_POINT('Ctrl Pts',(0.161082102388196,-6.11347850353662,6.059573277201));
#8608=CARTESIAN_POINT('Ctrl Pts',(0.330366942461903,-6.10431677141909,6.06729631216214));
#8609=CARTESIAN_POINT('Ctrl Pts',(0.499696771071035,-6.0951526045123,6.07502139956951));
#8610=CARTESIAN_POINT('Ctrl Pts',(0.66863482735465,-6.07893900172759,6.08274648697688));
#8611=CARTESIAN_POINT('Ctrl Pts',(0.836587234990848,-6.05573673145971,6.09047157438425));
#8612=CARTESIAN_POINT('Ctrl Pts',(1.00388837954898,-6.0326244318101,6.09816670649491));
#8613=CARTESIAN_POINT('Ctrl Pts',(1.17021120106051,-6.00257764240171,6.10586183860557));
#8614=CARTESIAN_POINT('Ctrl Pts',(1.33497655207619,-5.96570726468428,6.11355697071623));
#8615=CARTESIAN_POINT('Ctrl Pts',(1.50037510143476,-5.92869519296426,6.12128167545773));
#8616=CARTESIAN_POINT('Ctrl Pts',(1.66426275803222,-5.88479384477632,6.12900638019924));
#8617=CARTESIAN_POINT('Ctrl Pts',(1.82606175761478,-5.8341515252757,6.13673108494074));
#8618=CARTESIAN_POINT('Ctrl Pts',(1.98782868547295,-5.78351924407271,6.14445425849477));
#8619=CARTESIAN_POINT('Ctrl Pts',(2.14750748019648,-5.72614875246145,6.15217743204879));
#8620=CARTESIAN_POINT('Ctrl Pts',(2.30453548773657,-5.66223822779144,6.15990060560282));
#8621=CARTESIAN_POINT('Ctrl Pts',(2.46155959184305,-5.59832929182204,6.16762358717266));
#8622=CARTESIAN_POINT('Ctrl Pts',(2.61593274570186,-5.52788076395922,6.1753465687425));
#8623=CARTESIAN_POINT('Ctrl Pts',(2.76711159942012,-5.45113923495397,6.18306955031233));
#8624=CARTESIAN_POINT('Ctrl Pts',(2.91828130145515,-5.37440235153339,6.19079206436783));
#8625=CARTESIAN_POINT('Ctrl Pts',(3.06625680778526,-5.29137337273966,6.19851457842334));
#8626=CARTESIAN_POINT('Ctrl Pts',(3.21051845807112,-5.2023453165745,6.20623709247884));
#8627=CARTESIAN_POINT('Ctrl Pts',(3.35479862779034,-5.1133058315289,6.21396059790373));
#8628=CARTESIAN_POINT('Ctrl Pts',(3.49536371969221,-5.01826589756368,6.22168410332863));
#8629=CARTESIAN_POINT('Ctrl Pts',(3.63172160349,-4.91756278630421,6.22940760875352));
#8630=CARTESIAN_POINT('Ctrl Pts',(3.66233632378909,-4.89495318355452,6.2311416702667));
#8631=CARTESIAN_POINT('Ctrl Pts',(3.69273908654001,-4.8720582810407,6.23287573177987));
#8632=CARTESIAN_POINT('Ctrl Pts',(3.72292453512037,-4.84888218750454,6.23460979329304));
#8633=CARTESIAN_POINT('Ctrl Pts',(3.72292453512037,-4.84888218750453,4.4846183003358));
#8634=CARTESIAN_POINT('Ctrl Pts',(3.85738003164868,-4.74564856632129,4.49234091472402));
#8635=CARTESIAN_POINT('Ctrl Pts',(3.98754958283495,-4.63681087233664,4.50006352911223));
#8636=CARTESIAN_POINT('Ctrl Pts',(4.11297418411632,-4.52275015043863,4.50778614350044));
#8637=CARTESIAN_POINT('Ctrl Pts',(4.23840733119494,-4.40868165702058,4.5155092840685));
#8638=CARTESIAN_POINT('Ctrl Pts',(4.35909464600389,-4.28938963570915,4.52323242463655));
#8639=CARTESIAN_POINT('Ctrl Pts',(4.47461199751822,-4.1652938712852,4.53095556520461));
#8640=CARTESIAN_POINT('Ctrl Pts',(4.59012790250441,-4.04119966080974,4.53867860906217));
#8641=CARTESIAN_POINT('Ctrl Pts',(4.70047375972252,-3.91230206130686,4.54640165291973));
#8642=CARTESIAN_POINT('Ctrl Pts',(4.80526379357084,-3.77905615685943,4.55412469677729));
#8643=CARTESIAN_POINT('Ctrl Pts',(4.91007646117892,-3.6457814724252,4.56184940874691));
#8644=CARTESIAN_POINT('Ctrl Pts',(5.00933071284341,-3.50815685642527,4.56957412071653));
#8645=CARTESIAN_POINT('Ctrl Pts',(5.10268193066479,-3.36666937446596,4.57729883268615));
#8646=CARTESIAN_POINT('Ctrl Pts',(5.13437981000813,-3.31862658256237,4.57992179780316));
#8647=CARTESIAN_POINT('Ctrl Pts',(5.16539744813244,-3.27013866339535,4.58254476292016));
#8648=CARTESIAN_POINT('Ctrl Pts',(5.19572249657802,-3.22122543468368,4.58516772803716));
#8649=CARTESIAN_POINT('Ctrl Pts',(5.28503126530388,-3.0771735549815,4.59289249014036));
#8650=CARTESIAN_POINT('Ctrl Pts',(5.36836138009955,-2.92937973689538,4.60061725224357));
#8651=CARTESIAN_POINT('Ctrl Pts',(5.44541445031272,-2.77836049259728,4.60834201434678));
#8652=CARTESIAN_POINT('Ctrl Pts',(5.52245248987796,-2.627370707438,4.61606526959011));
#8653=CARTESIAN_POINT('Ctrl Pts',(5.59321578413792,-2.47315703363873,4.62378852483345));
#8654=CARTESIAN_POINT('Ctrl Pts',(5.65745214105643,-2.31626009639591,4.63151178007678));
#8655=CARTESIAN_POINT('Ctrl Pts',(5.72169098040162,-2.15935709584001,4.63923533378684));
#8656=CARTESIAN_POINT('Ctrl Pts',(5.77940225392466,-1.99977091612798,4.64695888749689));
#8657=CARTESIAN_POINT('Ctrl Pts',(5.83038182676192,-1.838062381059,4.65468244120695));
#8658=CARTESIAN_POINT('Ctrl Pts',(5.88135797557967,-1.67636470706926,4.66240547616808));
#8659=CARTESIAN_POINT('Ctrl Pts',(5.92560323320806,-1.51254526527581,4.67012851112921));
#8660=CARTESIAN_POINT('Ctrl Pts',(5.96296322514271,-1.34718044006572,4.67785154609034));
#8661=CARTESIAN_POINT('Ctrl Pts',(6.00033314573561,-1.18177166808926,4.68557663349771));
#8662=CARTESIAN_POINT('Ctrl Pts',(6.0308140722262,-1.0148170008996,4.69330172090507));
#8663=CARTESIAN_POINT('Ctrl Pts',(6.05430248239203,-0.846904371344088,4.70102680831244));
#8664=CARTESIAN_POINT('Ctrl Pts',(6.07769981238503,-0.679642850621103,4.70872194042308));
#8665=CARTESIAN_POINT('Ctrl Pts',(6.09415874759425,-0.511431097283521,4.71641707253371));
#8666=CARTESIAN_POINT('Ctrl Pts',(6.10362801536036,-0.342856548148325,4.72411220464435));
#8667=CARTESIAN_POINT('Ctrl Pts',(6.11313374440217,-0.173632905200967,4.73183696674755));
#8668=CARTESIAN_POINT('Ctrl Pts',(6.11559920859452,-0.00398373136690208,
4.73956172885075));
#8669=CARTESIAN_POINT('Ctrl Pts',(6.1110094978451,0.165494651717244,4.74728649095394));
#8670=CARTESIAN_POINT('Ctrl Pts',(6.10642068240492,0.334939974861039,4.75500974619727));
#8671=CARTESIAN_POINT('Ctrl Pts',(6.09477944669772,0.504214257114271,4.7627330014406));
#8672=CARTESIAN_POINT('Ctrl Pts',(6.07612298521814,0.672722105333136,4.77045625668393));
#8673=CARTESIAN_POINT('Ctrl Pts',(6.05746580275592,0.841236465570973,4.77817981039397));
#8674=CARTESIAN_POINT('Ctrl Pts',(6.03179288296159,1.0089840170759,4.78590336410402));
#8675=CARTESIAN_POINT('Ctrl Pts',(5.99919328418982,1.17537462174058,4.79362691781407));
#8676=CARTESIAN_POINT('Ctrl Pts',(5.96659587495507,1.34175405085698,4.80134995277519));
#8677=CARTESIAN_POINT('Ctrl Pts',(5.92707277868547,1.50677640447407,4.80907298773631));
#8678=CARTESIAN_POINT('Ctrl Pts',(5.88076419424647,1.6698616871372,4.81679602269744));
#8679=CARTESIAN_POINT('Ctrl Pts',(5.83444330300318,1.83299031076359,4.82452111010479));
#8680=CARTESIAN_POINT('Ctrl Pts',(5.78133340471915,1.99418052907824,4.83224619751215));
#8681=CARTESIAN_POINT('Ctrl Pts',(5.72162487809727,2.15286653484102,4.83997128491951));
#8682=CARTESIAN_POINT('Ctrl Pts',(5.6621478811054,2.31093720952329,4.84766641703019));
#8683=CARTESIAN_POINT('Ctrl Pts',(5.59612347945264,2.46652277728533,4.85536154914087));
#8684=CARTESIAN_POINT('Ctrl Pts',(5.52378769623179,2.61908286418325,4.86305668125155));
#8685=CARTESIAN_POINT('Ctrl Pts',(5.45117338514619,2.77223038144213,4.87078144335474));
#8686=CARTESIAN_POINT('Ctrl Pts',(5.37217324728784,2.92238329987741,4.87850620545794));
#8687=CARTESIAN_POINT('Ctrl Pts',(5.28705948742644,3.06901084046866,4.88623096756114));
#8688=CARTESIAN_POINT('Ctrl Pts',(5.20196233060183,3.2156097786053,4.89395422280446));
#8689=CARTESIAN_POINT('Ctrl Pts',(5.11075409040059,3.35868443715986,4.90167747804779));
#8690=CARTESIAN_POINT('Ctrl Pts',(5.01375228177231,3.49772978080397,4.90940073329111));
#8691=CARTESIAN_POINT('Ctrl Pts',(4.91674672448998,3.63678049788283,4.91712428700116));
#8692=CARTESIAN_POINT('Ctrl Pts',(4.81394732883338,3.77180132627353,4.92484784071121));
#8693=CARTESIAN_POINT('Ctrl Pts',(4.70571463859838,3.90231665841983,4.93257139442125));
#8694=CARTESIAN_POINT('Ctrl Pts',(4.59748921776214,4.032823224564,4.94029442938237));
#8695=CARTESIAN_POINT('Ctrl Pts',(4.48383143495245,4.15882465605924,4.9480174643435));
#8696=CARTESIAN_POINT('Ctrl Pts',(4.36514188924104,4.27987871899346,4.95574049930462));
#8697=CARTESIAN_POINT('Ctrl Pts',(4.24642080101916,4.40096495282382,4.96346558671198));
#8698=CARTESIAN_POINT('Ctrl Pts',(4.12266549827857,4.5171009628278,4.97119067411934));
#8699=CARTESIAN_POINT('Ctrl Pts',(3.99431385625943,4.62788098163662,4.97891576152669));
#8700=CARTESIAN_POINT('Ctrl Pts',(3.86645991883735,4.73823143270672,4.98661089363738));
#8701=CARTESIAN_POINT('Ctrl Pts',(3.73404548229173,4.8432671766407,4.99430602574806));
#8702=CARTESIAN_POINT('Ctrl Pts',(3.5975363353603,4.94262661732225,5.00200115785874));
#8703=CARTESIAN_POINT('Ctrl Pts',(3.46050156197515,5.04236864006238,5.00972591996194));
#8704=CARTESIAN_POINT('Ctrl Pts',(3.31929193105522,5.13642586111289,5.01745068206514));
#8705=CARTESIAN_POINT('Ctrl Pts',(3.17440041292128,5.22446242028261,5.02517544416834));
#8706=CARTESIAN_POINT('Ctrl Pts',(3.02953715859822,5.31248180626861,5.03289869941166));
#8707=CARTESIAN_POINT('Ctrl Pts',(2.88099372085466,5.39448270933945,5.04062195465499));
#8708=CARTESIAN_POINT('Ctrl Pts',(2.72929054152797,5.47017355322717,5.04834520989831));
#8709=CARTESIAN_POINT('Ctrl Pts',(2.57758149960195,5.5458673222025,5.05606876360836));
#8710=CARTESIAN_POINT('Ctrl Pts',(2.42271275355714,5.6152503989949,5.06379231731841));
#8711=CARTESIAN_POINT('Ctrl Pts',(2.26522845087726,5.67807763488984,5.07151587102845));
#8712=CARTESIAN_POINT('Ctrl Pts',(2.10775472555801,5.74090065102243,5.07923890598958));
#8713=CARTESIAN_POINT('Ctrl Pts',(1.9476660895506,5.79716858996948,5.0869619409507));
#8714=CARTESIAN_POINT('Ctrl Pts',(1.78552589699476,5.84668477290003,5.09468497591182));
#8715=CARTESIAN_POINT('Ctrl Pts',(1.62334261463946,5.8962141150748,5.10241006331918));
#8716=CARTESIAN_POINT('Ctrl Pts',(1.4591069889493,5.93898802102476,5.11013515072653));
#8717=CARTESIAN_POINT('Ctrl Pts',(1.29339766057976,5.97485966815178,5.11786023813389));
#8718=CARTESIAN_POINT('Ctrl Pts',(1.1283308973791,6.01059221706857,5.12555537024456));
#8719=CARTESIAN_POINT('Ctrl Pts',(0.961802152173548,6.03947590675075,5.13325050235524));
#8720=CARTESIAN_POINT('Ctrl Pts',(0.794393444370498,6.06141605716364,5.14094563446591));
#8721=CARTESIAN_POINT('Ctrl Pts',(0.62634013181097,6.0834406878016,5.1486703965691));
#8722=CARTESIAN_POINT('Ctrl Pts',(0.457340543251073,6.09847597173067,5.1563951586723));
#8723=CARTESIAN_POINT('Ctrl Pts',(0.287988254136562,6.1064628327682,5.16411992077549));
#8724=CARTESIAN_POINT('Ctrl Pts',(0.118669000365456,6.11444813581853,5.17184317601882));
#8725=CARTESIAN_POINT('Ctrl Pts',(-0.0510025002955841,6.11538774452854,
5.17956643126214));
#8726=CARTESIAN_POINT('Ctrl Pts',(-0.220429735668919,6.10927461276156,5.18728968650546));
#8727=CARTESIAN_POINT('Ctrl Pts',(-0.389863518591201,6.1031612447514,5.19501324021551));
#8728=CARTESIAN_POINT('Ctrl Pts',(-0.559052700481732,6.08999459833462,5.20273679392555));
#8729=CARTESIAN_POINT('Ctrl Pts',(-0.727402164915347,6.06981973809573,5.2104603476356));
#8730=CARTESIAN_POINT('Ctrl Pts',(-0.895740322234849,6.04964623289201,5.21818338259672));
#8731=CARTESIAN_POINT('Ctrl Pts',(-1.0632385602567,6.02246549354144,5.22590641755784));
#8732=CARTESIAN_POINT('Ctrl Pts',(-1.22930808609958,5.98837433632452,5.23362945251897));
#8733=CARTESIAN_POINT('Ctrl Pts',(-1.39542174598742,5.95427411916324,5.24135453992632));
#8734=CARTESIAN_POINT('Ctrl Pts',(-1.5601056238747,5.913259876027,5.24907962733367));
#8735=CARTESIAN_POINT('Ctrl Pts',(-1.7227813560714,5.86547951677208,5.25680471474103));
#8736=CARTESIAN_POINT('Ctrl Pts',(-1.88482628636772,5.8178844337167,5.26449984685172));
#8737=CARTESIAN_POINT('Ctrl Pts',(-2.04487832666801,5.76357573362856,5.27219497896241));
#8738=CARTESIAN_POINT('Ctrl Pts',(-2.20238109283932,5.70274873060386,5.27989011107311));
#8739=CARTESIAN_POINT('Ctrl Pts',(-2.36049032108483,5.64168751410266,5.28761487317631));
#8740=CARTESIAN_POINT('Ctrl Pts',(-2.51608659111276,5.57403604368506,5.2953396352795));
#8741=CARTESIAN_POINT('Ctrl Pts',(-2.6686204050553,5.50002642686583,5.3030643973827));
#8742=CARTESIAN_POINT('Ctrl Pts',(-2.82112446441408,5.42603124701166,5.31078765262604));
#8743=CARTESIAN_POINT('Ctrl Pts',(-2.97056697473137,5.34568053381436,5.31851090786939));
#8744=CARTESIAN_POINT('Ctrl Pts',(-3.11642075201407,5.25925348874877,5.32623416311273));
#8745=CARTESIAN_POINT('Ctrl Pts',(-3.26228016584448,5.17282310369314,5.33395771682278));
#8746=CARTESIAN_POINT('Ctrl Pts',(-3.40455029445344,5.08031607502897,5.34168127053282));
#8747=CARTESIAN_POINT('Ctrl Pts',(-3.5427301107876,4.98205669624693,5.34940482424287));
#8748=CARTESIAN_POINT('Ctrl Pts',(-3.6809006463382,4.88380391701069,5.357127859204));
#8749=CARTESIAN_POINT('Ctrl Pts',(-3.81498116107768,4.77979974450149,5.36485089416514));
#8750=CARTESIAN_POINT('Ctrl Pts',(-3.9445009403465,4.67041089135695,5.37257392912627));
#8751=CARTESIAN_POINT('Ctrl Pts',(-4.07405514033001,4.56099296742085,5.38029901653363));
#8752=CARTESIAN_POINT('Ctrl Pts',(-4.19904593917991,4.44618770630897,5.38802410394099));
#8753=CARTESIAN_POINT('Ctrl Pts',(-4.31903622504276,4.32640169763146,5.39574919134835));
#8754=CARTESIAN_POINT('Ctrl Pts',(-4.43856122884126,4.20708017889992,5.403444323459));
#8755=CARTESIAN_POINT('Ctrl Pts',(-4.55312423317451,4.08281671465023,5.41113945556965));
#8756=CARTESIAN_POINT('Ctrl Pts',(-4.66233010658665,3.95404900573017,5.41883458768029));
#8757=CARTESIAN_POINT('Ctrl Pts',(-4.77195647560163,3.82478547864853,5.42655934978349));
#8758=CARTESIAN_POINT('Ctrl Pts',(-4.87622318019224,3.69093715026868,5.43428411188669));
#8759=CARTESIAN_POINT('Ctrl Pts',(-4.97475873895932,3.55297073610914,5.44200887398989));
#8760=CARTESIAN_POINT('Ctrl Pts',(-5.07327507651592,3.41503123488863,5.44973212923323));
#8761=CARTESIAN_POINT('Ctrl Pts',(-5.16606231491152,3.27297550852698,5.45745538447657));
#8762=CARTESIAN_POINT('Ctrl Pts',(-5.25279109827068,3.12730095136819,5.46517863971991));
#8763=CARTESIAN_POINT('Ctrl Pts',(-5.33952323328064,2.98162076458762,5.47290219342995));
#8764=CARTESIAN_POINT('Ctrl Pts',(-5.42019627921881,2.83232173744498,5.48062574714));
#8765=CARTESIAN_POINT('Ctrl Pts',(-5.49452542264047,2.67992834651555,5.48834930085005));
#8766=CARTESIAN_POINT('Ctrl Pts',(-5.56884957377953,2.52754519101786,5.49607233581118));
#8767=CARTESIAN_POINT('Ctrl Pts',(-5.63683053612654,2.37206837251912,5.50379537077231));
#8768=CARTESIAN_POINT('Ctrl Pts',(-5.69823040890161,2.21404511461916,5.51151840573344));
#8769=CARTESIAN_POINT('Ctrl Pts',(-5.75964659908791,2.05597986102173,5.5192434931408));
#8770=CARTESIAN_POINT('Ctrl Pts',(-5.8144780879474,1.89536711057669,5.52696858054816));
#8771=CARTESIAN_POINT('Ctrl Pts',(-5.86253556051135,1.73277302732927,5.53469366795552));
#8772=CARTESIAN_POINT('Ctrl Pts',(-5.91040668232307,1.57080942937591,5.54238880006617));
#8773=CARTESIAN_POINT('Ctrl Pts',(-5.95155617160243,1.40688014571579,5.55008393217683));
#8774=CARTESIAN_POINT('Ctrl Pts',(-5.98584646198968,1.24155857533411,5.55777906428748));
#8775=CARTESIAN_POINT('Ctrl Pts',(-6.02107100601623,1.07173274800266,5.56568385356634));
#8776=CARTESIAN_POINT('Ctrl Pts',(-6.04906762166612,0.900389754905527,5.5735886428452));
#8777=CARTESIAN_POINT('Ctrl Pts',(-6.06973067897709,0.728144935561822,5.58149343212406));
#8778=CARTESIAN_POINT('Ctrl Pts',(-6.0903879230381,0.555948574787141,5.58939599750569));
#8779=CARTESIAN_POINT('Ctrl Pts',(-6.10371569436386,0.382851176372991,5.59729856288731));
#8780=CARTESIAN_POINT('Ctrl Pts',(-6.1096600488996,0.20947469866338,5.60520112826894));
#8781=CARTESIAN_POINT('Ctrl Pts',(-6.11205203894302,0.139708535499509,5.60838109635406));
#8782=CARTESIAN_POINT('Ctrl Pts',(-6.11324906863418,0.0698972401555901,
5.61156106443918));
#8783=CARTESIAN_POINT('Ctrl Pts',(-6.11324999945666,8.15052733772887E-5,
5.61474103252431));
#8784=CARTESIAN_POINT('Origin',(0.,0.,-3.86474103256053));
#8785=CARTESIAN_POINT('',(3.72292453512037,-4.84888218750454,2.73461001778677));
#8786=CARTESIAN_POINT('',(3.72292453512038,-4.84888218750453,2.88012709193022));
#8787=CARTESIAN_POINT('',(3.72292453512038,-4.84888218750453,-3.86474103256053));
#8788=CARTESIAN_POINT('',(-6.11324999945432,-8.16805581249634E-5,4.01025896739721));
#8789=CARTESIAN_POINT('Ctrl Pts',(3.72292453512039,-4.84888218750453,2.88012709193022));
#8790=CARTESIAN_POINT('Ctrl Pts',(3.85740722513931,-4.74562768742394,2.88785179219662));
#8791=CARTESIAN_POINT('Ctrl Pts',(3.98757783499191,-4.63678558761364,2.89557649246302));
#8792=CARTESIAN_POINT('Ctrl Pts',(4.1129822323414,-4.52274283139601,2.90330119272942));
#8793=CARTESIAN_POINT('Ctrl Pts',(4.1483088696491,-4.49061678819799,2.90547725425828));
#8794=CARTESIAN_POINT('Ctrl Pts',(4.18325748915386,-4.45807828123202,2.90765331578713));
#8795=CARTESIAN_POINT('Ctrl Pts',(4.21781844241679,-4.42513651194049,2.90982937731599));
#8796=CARTESIAN_POINT('Ctrl Pts',(4.34050575545397,-4.30819711127285,2.91755413941812));
#8797=CARTESIAN_POINT('Ctrl Pts',(4.45834856405392,-4.18613158317652,2.92527890152026));
#8798=CARTESIAN_POINT('Ctrl Pts',(4.57092809274141,-4.05936472043192,2.93300366362239));
#8799=CARTESIAN_POINT('Ctrl Pts',(4.68348566067742,-3.93262258594478,2.94072691886459));
#8800=CARTESIAN_POINT('Ctrl Pts',(4.79078178701837,-3.80118118354429,2.9484501741068));
#8801=CARTESIAN_POINT('Ctrl Pts',(4.89243633951613,-3.66550026957877,2.956173429349));
#8802=CARTESIAN_POINT('Ctrl Pts',(4.9940948204743,-3.52981411219733,2.96389698305794));
#8803=CARTESIAN_POINT('Ctrl Pts',(5.09011109812451,-3.38988836665788,2.97162053676688));
#8804=CARTESIAN_POINT('Ctrl Pts',(5.18014646731156,-3.24621443218091,2.97934409047582));
#8805=CARTESIAN_POINT('Ctrl Pts',(5.27017578931429,-3.1025501474979,2.98706712543581));
#8806=CARTESIAN_POINT('Ctrl Pts',(5.3542248384284,-2.9551384462428,2.9947901603958));
#8807=CARTESIAN_POINT('Ctrl Pts',(5.4319991521926,-2.80449831040757,3.0025131953558));
#8808=CARTESIAN_POINT('Ctrl Pts',(5.50979413498119,-2.6538181409868,3.01023828276203));
#8809=CARTESIAN_POINT('Ctrl Pts',(5.58131090281586,-2.4999081033464,3.01796337016827));
#8810=CARTESIAN_POINT('Ctrl Pts',(5.64630130242559,-2.34331115405682,3.0256884575745));
#8811=CARTESIAN_POINT('Ctrl Pts',(5.71103969113038,-2.18732143505259,3.03338358969073));
#8812=CARTESIAN_POINT('Ctrl Pts',(5.76930214586503,-2.02866590593596,3.04107872180696));
#8813=CARTESIAN_POINT('Ctrl Pts',(5.82089120605154,-1.86790019267943,3.04877385392319));
#8814=CARTESIAN_POINT('Ctrl Pts',(5.87267890912134,-1.7065154535151,3.05649861602735));
#8815=CARTESIAN_POINT('Ctrl Pts',(5.91776003709367,-1.54294708064208,3.06422337813152));
#8816=CARTESIAN_POINT('Ctrl Pts',(5.95597008558128,-1.37776845012541,3.07194814023568));
#8817=CARTESIAN_POINT('Ctrl Pts',(5.9941726804816,-1.21262204080153,3.07967139547997));
#8818=CARTESIAN_POINT('Ctrl Pts',(6.02550679895802,-1.04586630918302,3.08739465072427));
#8819=CARTESIAN_POINT('Ctrl Pts',(6.04985859784319,-0.878086845706551,3.09511790596856));
#8820=CARTESIAN_POINT('Ctrl Pts',(6.07421133780852,-0.710300898359008,3.10284145967961));
#8821=CARTESIAN_POINT('Ctrl Pts',(6.0915811687888,-0.541491453049558,3.11056501339066));
#8822=CARTESIAN_POINT('Ctrl Pts',(6.10190576470393,-0.372252066714117,3.1182885671017));
#8823=CARTESIAN_POINT('Ctrl Pts',(6.1122296671723,-0.203024047264704,3.1260116020638));
#8824=CARTESIAN_POINT('Ctrl Pts',(6.11550926221234,-0.0333664609460739,
3.13373463702589));
#8825=CARTESIAN_POINT('Ctrl Pts',(6.11173427081301,0.136124081152851,3.14145767198798));
#8826=CARTESIAN_POINT('Ctrl Pts',(6.10795827618541,0.30565966645452,3.14918275939633));
#8827=CARTESIAN_POINT('Ctrl Pts',(6.09712395369223,0.475027801708435,3.15690784680469));
#8828=CARTESIAN_POINT('Ctrl Pts',(6.07927315977078,0.643632978793483,3.16463293421304));
#8829=CARTESIAN_POINT('Ctrl Pts',(6.06149158525163,0.811584361451595,3.17232806631882));
#8830=CARTESIAN_POINT('Ctrl Pts',(6.03674792255507,0.978778385355505,3.1800231984246));
#8831=CARTESIAN_POINT('Ctrl Pts',(6.00513460410749,1.14463266992115,3.18771833053038));
#8832=CARTESIAN_POINT('Ctrl Pts',(5.9733995590264,1.31112557405299,3.195443092633));
#8833=CARTESIAN_POINT('Ctrl Pts',(5.93473058105001,1.4763273622822,3.20316785473561));
#8834=CARTESIAN_POINT('Ctrl Pts',(5.88925753445974,1.63965583440829,3.21089261683823));
#8835=CARTESIAN_POINT('Ctrl Pts',(5.84379335824084,1.80295244624988,3.21861587208099));
#8836=CARTESIAN_POINT('Ctrl Pts',(5.79152784672204,1.96437616601436,3.22633912732375));
#8837=CARTESIAN_POINT('Ctrl Pts',(5.73264119483716,2.12335830555183,3.2340623825665));
#8838=CARTESIAN_POINT('Ctrl Pts',(5.67375226726619,2.28234658898495,3.24178593627596));
#8839=CARTESIAN_POINT('Ctrl Pts',(5.60824179366985,2.43889280481764,3.24950948998542));
#8840=CARTESIAN_POINT('Ctrl Pts',(5.53633901888734,2.59244591659026,3.25723304369488));
#8841=CARTESIAN_POINT('Ctrl Pts',(5.46444107342178,2.74598871503844,3.26495607865539));
#8842=CARTESIAN_POINT('Ctrl Pts',(5.38615182035971,2.89653852467828,3.27267911361589));
#8843=CARTESIAN_POINT('Ctrl Pts',(5.30174766962646,3.04356652795867,3.2804021485764));
#8844=CARTESIAN_POINT('Ctrl Pts',(5.21732108794688,3.1906336048773,3.28812723598316));
#8845=CARTESIAN_POINT('Ctrl Pts',(5.12677651731211,3.33417672906057,3.29585232338992));
#8846=CARTESIAN_POINT('Ctrl Pts',(5.03043562145371,3.47369299462541,3.30357741079668));
#8847=CARTESIAN_POINT('Ctrl Pts',(4.9344683032164,3.61266826299348,3.31127254291031));
#8848=CARTESIAN_POINT('Ctrl Pts',(4.83274973616982,3.74764760826321,3.31896767502394));
#8849=CARTESIAN_POINT('Ctrl Pts',(4.72563971554549,3.87816384921513,3.32666280713756));
#8850=CARTESIAN_POINT('Ctrl Pts',(4.61811726940627,4.00918264097942,3.33438756924104));
#8851=CARTESIAN_POINT('Ctrl Pts',(4.50512366338708,4.13575027387649,3.34211233134452));
#8852=CARTESIAN_POINT('Ctrl Pts',(4.38705147630667,4.25741763358206,3.349837093448));
#8853=CARTESIAN_POINT('Ctrl Pts',(4.2690023214234,4.37906125978456,3.35756034869158));
#8854=CARTESIAN_POINT('Ctrl Pts',(4.14587678280687,4.49580629284127,3.36528360393516));
#8855=CARTESIAN_POINT('Ctrl Pts',(4.01810517137538,4.60723956336834,3.37300685917875));
#8856=CARTESIAN_POINT('Ctrl Pts',(3.89032862218446,4.71867714025639,3.38073041288907));
#8857=CARTESIAN_POINT('Ctrl Pts',(3.75790587713221,4.82480233256016,3.38845396659939));
#8858=CARTESIAN_POINT('Ctrl Pts',(3.62130187405447,4.92524093821506,3.39617752030971));
#8859=CARTESIAN_POINT('Ctrl Pts',(3.48470704592134,5.02567279795752,3.40390055527113));
#8860=CARTESIAN_POINT('Ctrl Pts',(3.34393177711988,5.12041864761897,3.41162359023254));
#8861=CARTESIAN_POINT('Ctrl Pts',(3.19947179220364,5.20914636129503,3.41934662519396));
#8862=CARTESIAN_POINT('Ctrl Pts',(3.05497341611712,5.29789765493177,3.42707171260159));
#8863=CARTESIAN_POINT('Ctrl Pts',(2.90678863626768,5.38062744883377,3.43479680000923));
#8864=CARTESIAN_POINT('Ctrl Pts',(2.75544051885762,5.45704802155319,3.44252188741687));
#8865=CARTESIAN_POINT('Ctrl Pts',(2.60467927869192,5.53317226091944,3.45021701952616));
#8866=CARTESIAN_POINT('Ctrl Pts',(2.45077948328852,5.60303601027428,3.45791215163546));
#8867=CARTESIAN_POINT('Ctrl Pts',(2.2942805913903,5.66640116215484,3.46560728374476));
#8868=CARTESIAN_POINT('Ctrl Pts',(2.13717910279434,5.73001030062734,3.47333204584786));
#8869=CARTESIAN_POINT('Ctrl Pts',(1.9774028104633,5.78709319740479,3.48105680795096));
#8870=CARTESIAN_POINT('Ctrl Pts',(1.81551131753373,5.83744329466308,3.48878157005407));
#8871=CARTESIAN_POINT('Ctrl Pts',(1.6536514045795,5.88778357018954,3.49650482529729));
#8872=CARTESIAN_POINT('Ctrl Pts',(1.48967741677477,5.93139357275478,3.50422808054051));
#8873=CARTESIAN_POINT('Ctrl Pts',(1.324164893687,5.9681163608652,3.51195133578372));
#8874=CARTESIAN_POINT('Ctrl Pts',(1.15864597433448,6.00484056813516,3.51967488949369));
#8875=CARTESIAN_POINT('Ctrl Pts',(0.991588709257809,6.03467695583886,3.52739844320366));
#8876=CARTESIAN_POINT('Ctrl Pts',(0.823580401719469,6.05751936723306,3.53512199691363));
#8877=CARTESIAN_POINT('Ctrl Pts',(0.655583378381846,6.08036024442719,3.54284503187467));
#8878=CARTESIAN_POINT('Ctrl Pts',(0.486635754478305,6.09620804265871,3.5505680668357));
#8879=CARTESIAN_POINT('Ctrl Pts',(0.317331737426225,6.10500828262518,3.55829110179674));
#8880=CARTESIAN_POINT('Ctrl Pts',(0.147982726742336,6.11381086131204,3.56601618920401));
#8881=CARTESIAN_POINT('Ctrl Pts',(-0.021722549741907,6.11556212051749,3.57374127661127));
#8882=CARTESIAN_POINT('Ctrl Pts',(-0.191187119584226,6.11025965469595,3.58146636401854));
#8883=CARTESIAN_POINT('Ctrl Pts',(-0.359994562703326,6.10497775005717,3.58916149612967));
#8884=CARTESIAN_POINT('Ctrl Pts',(-0.528562851593163,6.092696769089,3.5968566282408));
#8885=CARTESIAN_POINT('Ctrl Pts',(-0.696304355874567,6.07346571625214,3.60455176035192));
#8886=CARTESIAN_POINT('Ctrl Pts',(-0.864691746330856,6.0541606145315,3.61227652245514));
#8887=CARTESIAN_POINT('Ctrl Pts',(-1.03230560687944,6.02784494527547,3.62000128455836));
#8888=CARTESIAN_POINT('Ctrl Pts',(-1.19855571209354,5.99460505517319,3.62772604666157));
#8889=CARTESIAN_POINT('Ctrl Pts',(-1.36477338710263,5.96137164913568,3.63544930190488));
#8890=CARTESIAN_POINT('Ctrl Pts',(-1.52962752700772,5.92121677947923,3.64317255714818));
#8891=CARTESIAN_POINT('Ctrl Pts',(-1.6925376500896,5.87427798674264,3.65089581239149));
#8892=CARTESIAN_POINT('Ctrl Pts',(-1.85545406886596,5.82733738004696,3.65861936610155));
#8893=CARTESIAN_POINT('Ctrl Pts',(-2.01642601485949,5.77361240959754,3.6663429198116));
#8894=CARTESIAN_POINT('Ctrl Pts',(-2.17488697325315,5.71329083944392,3.67406647352166));
#8895=CARTESIAN_POINT('Ctrl Pts',(-2.3333372886891,5.65297332076093,3.68178950848277));
#8896=CARTESIAN_POINT('Ctrl Pts',(-2.48927665780199,5.58606020177335,3.68951254344388));
#8897=CARTESIAN_POINT('Ctrl Pts',(-2.64215722705511,5.51278792899023,3.69723557840499));
#8898=CARTESIAN_POINT('Ctrl Pts',(-2.79507842530368,5.43949618362894,3.70496066581236));
#8899=CARTESIAN_POINT('Ctrl Pts',(-2.94493891238881,5.35984204257687,3.71268575321972));
#8900=CARTESIAN_POINT('Ctrl Pts',(-3.09121332034152,5.27410900253713,3.72041084062709));
#8901=CARTESIAN_POINT('Ctrl Pts',(-3.23692052522489,5.18870840645757,3.72810597273777));
#8902=CARTESIAN_POINT('Ctrl Pts',(-3.37906915972562,5.09727615711957,3.73580110484845));
#8903=CARTESIAN_POINT('Ctrl Pts',(-3.51716665543486,5.00013642617851,3.74349623695913));
#8904=CARTESIAN_POINT('Ctrl Pts',(-3.65579589351149,4.90262266013831,3.75122099906233));
#8905=CARTESIAN_POINT('Ctrl Pts',(-3.79039181424287,4.7993228110639,3.75894576116554));
#8906=CARTESIAN_POINT('Ctrl Pts',(-3.92047743605519,4.69059508334306,3.76667052326874));
#8907=CARTESIAN_POINT('Ctrl Pts',(-4.05053768222588,4.58188856500582,3.77439377851214));
#8908=CARTESIAN_POINT('Ctrl Pts',(-4.17608914200571,4.46775648385058,3.78211703375554));
#8909=CARTESIAN_POINT('Ctrl Pts',(-4.29668788265976,4.34859733724621,3.78984028899894));
#8910=CARTESIAN_POINT('Ctrl Pts',(-4.41729128387497,4.22943358571406,3.797563842709));
#8911=CARTESIAN_POINT('Ctrl Pts',(-4.53294135474333,4.10524259991034,3.80528739641906));
#8912=CARTESIAN_POINT('Ctrl Pts',(-4.64323045562768,3.97646029760535,3.81301095012911));
#8913=CARTESIAN_POINT('Ctrl Pts',(-4.75351214899525,3.84768664490451,3.82073398509024));
#8914=CARTESIAN_POINT('Ctrl Pts',(-4.85843338676705,3.71432253355324,3.82845702005136));
#8915=CARTESIAN_POINT('Ctrl Pts',(-4.95762620737575,3.5768377025581,3.83618005501249));
#8916=CARTESIAN_POINT('Ctrl Pts',(-5.0568453891149,3.43931633408433,3.84390514241986));
#8917=CARTESIAN_POINT('Ctrl Pts',(-5.15033292430782,3.29767231359746,3.85163022982722));
#8918=CARTESIAN_POINT('Ctrl Pts',(-5.23776310674007,3.15240593835448,3.85935531723459));
#8919=CARTESIAN_POINT('Ctrl Pts',(-5.32485426426226,3.00770285737021,3.86705044934517));
#8920=CARTESIAN_POINT('Ctrl Pts',(-5.40593482891385,2.85940574834771,3.87474558145574));
#8921=CARTESIAN_POINT('Ctrl Pts',(-5.48072735671713,2.70803493401257,3.88244071356631));
#8922=CARTESIAN_POINT('Ctrl Pts',(-5.55558719194807,2.55652789777887,3.89014277069417));
#8923=CARTESIAN_POINT('Ctrl Pts',(-5.62417561300256,2.40188493173974,3.89784482782203));
#8924=CARTESIAN_POINT('Ctrl Pts',(-5.68624590948509,2.24464541060813,3.90554688494989));
#8925=CARTESIAN_POINT('Ctrl Pts',(-5.74830346396685,2.08743816813815,3.91324736097337));
#8926=CARTESIAN_POINT('Ctrl Pts',(-5.80384544591209,1.92763573217092,3.92094783699684));
#8927=CARTESIAN_POINT('Ctrl Pts',(-5.85267341985573,1.76579710131551,3.92864831302032));
#8928=CARTESIAN_POINT('Ctrl Pts',(-5.9015019239919,1.60395671315531,3.93634887265846));
#8929=CARTESIAN_POINT('Ctrl Pts',(-5.94361617794235,1.44008039172325,3.94404943229661));
#8930=CARTESIAN_POINT('Ctrl Pts',(-5.97886752376897,1.27474259979051,3.95174999193475));
#8931=CARTESIAN_POINT('Ctrl Pts',(-6.01411712626691,1.1094129845134,3.95945017074754));
#8932=CARTESIAN_POINT('Ctrl Pts',(-6.04250443368888,0.9426223571398,3.96715034956032));
#8933=CARTESIAN_POINT('Ctrl Pts',(-6.06393180476829,0.774955888821809,3.9748505283731));
#8934=CARTESIAN_POINT('Ctrl Pts',(-6.08536381698891,0.607253104160884,3.98255237503479));
#8935=CARTESIAN_POINT('Ctrl Pts',(-6.0998328402343,0.438674417704038,3.99025422169647));
#8936=CARTESIAN_POINT('Ctrl Pts',(-6.10729296440831,0.26981143302088,3.99795606835815));
#8937=CARTESIAN_POINT('Ctrl Pts',(-6.1112652219098,0.179897747673746,4.0020570347045));
#8938=CARTESIAN_POINT('Ctrl Pts',(-6.11325120176772,0.0899035318141606,
4.00615800105085));
#8939=CARTESIAN_POINT('Ctrl Pts',(-6.11324999945432,-8.1680558123466E-5,
4.0102589673972));
#8940=CARTESIAN_POINT('Ctrl Pts',(-6.11324999945431,-8.16814850665972E-5,
4.01025896743945));
#8941=CARTESIAN_POINT('Ctrl Pts',(-6.11324891212047,-0.081460510364748,
4.0139677083508));
#8942=CARTESIAN_POINT('Ctrl Pts',(-6.11162270832985,-0.162834847314414,
4.01767644926215));
#8943=CARTESIAN_POINT('Ctrl Pts',(-6.10837287883718,-0.244144087756446,
4.0213851901735));
#8944=CARTESIAN_POINT('Ctrl Pts',(-6.10160396175534,-0.413499282476559,
4.02910995227672));
#8945=CARTESIAN_POINT('Ctrl Pts',(-6.08778642357728,-0.582602790231776,
4.03683471437994));
#8946=CARTESIAN_POINT('Ctrl Pts',(-6.06696261821026,-0.750859608541673,
4.04455947648316));
#8947=CARTESIAN_POINT('Ctrl Pts',(-6.04614287491734,-0.919083605200879,
4.05228273172653));
#8948=CARTESIAN_POINT('Ctrl Pts',(-6.0183196304021,-1.08646092763768,4.0600059869699));
#8949=CARTESIAN_POINT('Ctrl Pts',(-5.98358701388492,-1.25240249511397,4.06772924221327));
#8950=CARTESIAN_POINT('Ctrl Pts',(-5.94885305511907,-1.4183504754342,4.07545279592333));
#8951=CARTESIAN_POINT('Ctrl Pts',(-5.90720925108868,-1.58286227875742,4.0831763496334));
#8952=CARTESIAN_POINT('Ctrl Pts',(-5.85880085173651,-1.74535902959579,4.09089990334346));
#8953=CARTESIAN_POINT('Ctrl Pts',(-5.81039570371216,-1.90784486641479,4.09862293830459));
#8954=CARTESIAN_POINT('Ctrl Pts',(-5.75522696007558,-2.06831561782367,4.10634597326573));
#8955=CARTESIAN_POINT('Ctrl Pts',(-5.69348980268939,-2.2262074092887,4.11406900822687));
#8956=CARTESIAN_POINT('Ctrl Pts',(-5.63173623825635,-2.38414116151334,4.12179409563424));
#8957=CARTESIAN_POINT('Ctrl Pts',(-5.56341088540832,-2.53949428808111,4.12951918304162));
#8958=CARTESIAN_POINT('Ctrl Pts',(-5.48875751365973,-2.69172185018138,4.13724427044899));
#8959=CARTESIAN_POINT('Ctrl Pts',(-5.41439362263685,-2.84335912487575,4.14493940255955));
#8960=CARTESIAN_POINT('Ctrl Pts',(-5.33375086774613,-2.9918947656903,4.15263453467011));
#8961=CARTESIAN_POINT('Ctrl Pts',(-5.24711601306163,-3.13681352776544,4.16032966678067));
#8962=CARTESIAN_POINT('Ctrl Pts',(-5.16014757214769,-3.28229029739528,4.16805442888386));
#8963=CARTESIAN_POINT('Ctrl Pts',(-5.06710996744875,-3.42417378765433,4.17577919098705));
#8964=CARTESIAN_POINT('Ctrl Pts',(-4.96832505762452,-3.56196177467984,4.18350395309024));
#8965=CARTESIAN_POINT('Ctrl Pts',(-4.86955941765144,-3.69972288357177,4.19122720833357));
#8966=CARTESIAN_POINT('Ctrl Pts',(-4.76504889413752,-3.83338982591715,4.19895046357689));
#8967=CARTESIAN_POINT('Ctrl Pts',(-4.65515797786181,-3.96249034871374,4.20667371882021));
#8968=CARTESIAN_POINT('Ctrl Pts',(-4.54526281483007,-4.09159586062538,4.21439727253025));
#8969=CARTESIAN_POINT('Ctrl Pts',(-4.42998704536689,-4.21613435596427,4.22212082624029));
#8970=CARTESIAN_POINT('Ctrl Pts',(-4.30973516820192,-4.33566700087352,4.22984437995033));
#8971=CARTESIAN_POINT('Ctrl Pts',(-4.18949136769876,-4.45519161742786,4.23756741491145));
#8972=CARTESIAN_POINT('Ctrl Pts',(-4.0642723531173,-4.56971083293029,4.24529044987257));
#8973=CARTESIAN_POINT('Ctrl Pts',(-3.93451929281437,-4.67882287514408,4.25301348483369));
#8974=CARTESIAN_POINT('Ctrl Pts',(-3.80473174980083,-4.78796391458512,4.26073857224104));
#8975=CARTESIAN_POINT('Ctrl Pts',(-3.67040799460991,-4.89169470349284,4.26846365964839));
#8976=CARTESIAN_POINT('Ctrl Pts',(-3.53202280228015,-4.9896533433369,4.27618874705574));
#8977=CARTESIAN_POINT('Ctrl Pts',(-3.39417422128802,-5.08723213244784,4.28388387916645));
#8978=CARTESIAN_POINT('Ctrl Pts',(-3.25229591838128,-5.17908330377386,4.29157901127716));
#8979=CARTESIAN_POINT('Ctrl Pts',(-3.10688621678911,-5.26489160367294,4.29927414338787));
#8980=CARTESIAN_POINT('Ctrl Pts',(-2.96091661728943,-5.35103030716294,4.30699890549107));
#8981=CARTESIAN_POINT('Ctrl Pts',(-2.81133665657384,-5.43110999278065,4.31472366759427));
#8982=CARTESIAN_POINT('Ctrl Pts',(-2.6586692457176,-5.50484363123744,4.32244842969748));
#8983=CARTESIAN_POINT('Ctrl Pts',(-2.50603161550612,-5.57856288656373,4.33017168494081));
#8984=CARTESIAN_POINT('Ctrl Pts',(-2.35030802210038,-5.64593842706568,4.33789494018413));
#8985=CARTESIAN_POINT('Ctrl Pts',(-2.19204447401633,-5.70672993810242,4.34561819542746));
#8986=CARTESIAN_POINT('Ctrl Pts',(-2.03377480980615,-5.76752379843914,4.35334174913751));
#8987=CARTESIAN_POINT('Ctrl Pts',(-1.87296528892247,-5.82173300282247,4.36106530284756));
#8988=CARTESIAN_POINT('Ctrl Pts',(-1.71018106321062,-5.86916572380912,4.36878885655762));
#8989=CARTESIAN_POINT('Ctrl Pts',(-1.54740777082637,-5.91659525899888,4.37651189151874));
#8990=CARTESIAN_POINT('Ctrl Pts',(-1.3826603433326,-5.95724913293791,4.38423492647986));
#8991=CARTESIAN_POINT('Ctrl Pts',(-1.2165184017685,-5.99098560678113,4.39195796144099));
#8992=CARTESIAN_POINT('Ctrl Pts',(-1.05033230691417,-6.02473104630939,4.39968304884835));
#8993=CARTESIAN_POINT('Ctrl Pts',(-0.882751267811871,-6.05155534703707,
4.40740813625572));
#8994=CARTESIAN_POINT('Ctrl Pts',(-0.714365339658028,-6.07136786268097,
4.41513322366309));
#8995=CARTESIAN_POINT('Ctrl Pts',(-0.546632355629441,-6.09110355203755,
4.42282835577374));
#8996=CARTESIAN_POINT('Ctrl Pts',(-0.378101027449535,-6.10388173387967,
4.4305234878844));
#8997=CARTESIAN_POINT('Ctrl Pts',(-0.20935977231692,-6.10966398816133,4.43821861999506));
#8998=CARTESIAN_POINT('Ctrl Pts',(-0.0399687814736328,-6.1154685069277,
4.44594338209826));
#8999=CARTESIAN_POINT('Ctrl Pts',(0.129693750450044,-6.11422514153443,4.45366814420145));
#9000=CARTESIAN_POINT('Ctrl Pts',(0.299031318382102,-6.10593202002173,4.46139290630465));
#9001=CARTESIAN_POINT('Ctrl Pts',(0.468335853842491,-6.09764051623807,4.46911616154798));
#9002=CARTESIAN_POINT('Ctrl Pts',(0.637315235442858,-6.08230201581923,4.4768394167913));
#9003=CARTESIAN_POINT('Ctrl Pts',(0.805375025299262,-6.05996671864823,4.48456267203463));
#9004=CARTESIAN_POINT('Ctrl Pts',(0.973441309859275,-6.03763055832528,4.49228622574468));
#9005=CARTESIAN_POINT('Ctrl Pts',(1.14058761688449,-6.00829709800294,4.50000977945472));
#9006=CARTESIAN_POINT('Ctrl Pts',(1.30622589592708,-5.97206827416679,4.50773333316477));
#9007=CARTESIAN_POINT('Ctrl Pts',(1.47185304995097,-5.93584188362291,4.51545636812588));
#9008=CARTESIAN_POINT('Ctrl Pts',(1.63597206904608,-5.89272112408309,4.52317940308701));
#9009=CARTESIAN_POINT('Ctrl Pts',(1.79800616083802,-5.84285883862416,4.53090243804812));
#9010=CARTESIAN_POINT('Ctrl Pts',(1.96008331423251,-5.79298330194202,4.53862752545548));
#9011=CARTESIAN_POINT('Ctrl Pts',(2.12007412936835,-5.73636275047694,4.54635261286283));
#9012=CARTESIAN_POINT('Ctrl Pts',(2.27741709554115,-5.67319988502405,4.55407770027018));
#9013=CARTESIAN_POINT('Ctrl Pts',(2.4341499384906,-5.61028194396788,4.56177283238087));
#9014=CARTESIAN_POINT('Ctrl Pts',(2.5882551532058,-5.54087248274603,4.56946796449157));
#9015=CARTESIAN_POINT('Ctrl Pts',(2.73919765391028,-5.46521927970986,4.57716309660226));
#9016=CARTESIAN_POINT('Ctrl Pts',(2.89071986958217,-5.38927552037625,4.58488778290239));
#9017=CARTESIAN_POINT('Ctrl Pts',(3.0391086801984,-5.30701304086964,4.59261246920252));
#9018=CARTESIAN_POINT('Ctrl Pts',(3.18383939880802,-5.21871557426708,4.60033715550265));
#9019=CARTESIAN_POINT('Ctrl Pts',(3.3285436798381,-5.13043423673041,4.60806043075467));
#9020=CARTESIAN_POINT('Ctrl Pts',(3.46959093155419,-5.03612027631624,4.61578370600668));
#9021=CARTESIAN_POINT('Ctrl Pts',(3.60648317551241,-4.93610217350147,4.62350698125869));
#9022=CARTESIAN_POINT('Ctrl Pts',(3.64564048854767,-4.9074925163882,4.62571618389834));
#9023=CARTESIAN_POINT('Ctrl Pts',(3.68445801165065,-4.87841640971667,4.627925386538));
#9024=CARTESIAN_POINT('Ctrl Pts',(3.72292453512038,-4.84888218750453,4.63013458917765));
#9025=CARTESIAN_POINT('',(-6.11324999817629,-0.000149323895545952,3.86474103251618));
#9026=CARTESIAN_POINT('Ctrl Pts',(-6.11324999817626,-0.000149324869336022,
3.86474103256055));
#9027=CARTESIAN_POINT('Ctrl Pts',(-6.11324540503865,-0.188188990505417,
3.87330913670744));
#9028=CARTESIAN_POINT('Ctrl Pts',(-6.10455976566219,-0.376188117694265,
3.88187724085434));
#9029=CARTESIAN_POINT('Ctrl Pts',(-6.08723465950245,-0.563382430194741,
3.89044534500124));
#9030=CARTESIAN_POINT('Ctrl Pts',(-6.07161483028389,-0.732151565863044,
3.89817010710471));
#9031=CARTESIAN_POINT('Ctrl Pts',(-6.0489692004611,-0.900300595441643,3.90589486920817));
#9032=CARTESIAN_POINT('Ctrl Pts',(-6.01937119477572,-1.0672375471301,3.91361963131164));
#9033=CARTESIAN_POINT('Ctrl Pts',(-5.98977896273696,-1.23414193463244,3.92134288655525));
#9034=CARTESIAN_POINT('Ctrl Pts',(-5.95323711621792,-1.39983440415421,3.92906614179887));
#9035=CARTESIAN_POINT('Ctrl Pts',(-5.9098704745594,-1.56373160626468,3.93678939704248));
#9036=CARTESIAN_POINT('Ctrl Pts',(-5.86650215698853,-1.72763514221457,3.9445129507528));
#9037=CARTESIAN_POINT('Ctrl Pts',(-5.81630859374343,-1.88974296453487,3.95223650446312));
#9038=CARTESIAN_POINT('Ctrl Pts',(-5.7594651209688,-2.04948458956,3.95996005817344));
#9039=CARTESIAN_POINT('Ctrl Pts',(-5.70262546605979,-2.20921548561255,3.96768309313483));
#9040=CARTESIAN_POINT('Ctrl Pts',(-5.63913690168427,-2.3665802037917,3.97540612809623));
#9041=CARTESIAN_POINT('Ctrl Pts',(-5.56922384271879,-2.52102585313848,3.98312916305763));
#9042=CARTESIAN_POINT('Ctrl Pts',(-5.49929220390803,-2.67551254741034,3.99085425046526));
#9043=CARTESIAN_POINT('Ctrl Pts',(-5.42293278760885,-2.82707833286508,3.99857933787289));
#9044=CARTESIAN_POINT('Ctrl Pts',(-5.3404175391466,-2.97519177030244,4.00630442528053));
#9045=CARTESIAN_POINT('Ctrl Pts',(-5.25822225714617,-3.12273087349967,4.01399955738982));
#9046=CARTESIAN_POINT('Ctrl Pts',(-5.16991897872069,-3.2668440981476,4.02169468949912));
#9047=CARTESIAN_POINT('Ctrl Pts',(-5.07582103137174,-3.40703190768509,4.02938982160841));
#9048=CARTESIAN_POINT('Ctrl Pts',(-4.98136076125069,-3.54775950833596,4.03711458371152));
#9049=CARTESIAN_POINT('Ctrl Pts',(-4.88102762909894,-3.68458122915613,4.04483934581462));
#9050=CARTESIAN_POINT('Ctrl Pts',(-4.775169327721,-3.81701237279794,4.05256410791773));
#9051=CARTESIAN_POINT('Ctrl Pts',(-4.66933167599206,-3.94941768325901,4.06028736316097));
#9052=CARTESIAN_POINT('Ctrl Pts',(-4.55797120337342,-4.07743387808856,4.06801061840421));
#9053=CARTESIAN_POINT('Ctrl Pts',(-4.44147660841494,-4.20060842014617,4.07573387364745));
#9054=CARTESIAN_POINT('Ctrl Pts',(-4.32497751150002,-4.32378772230809,4.0834574273574));
#9055=CARTESIAN_POINT('Ctrl Pts',(-4.20334411010281,-4.44212476431314,4.09118098106735));
#9056=CARTESIAN_POINT('Ctrl Pts',(-4.07700330753907,-4.55520247550155,4.0989045347773));
#9057=CARTESIAN_POINT('Ctrl Pts',(-3.95067099059709,-4.66827259187763,4.10662756973833));
#9058=CARTESIAN_POINT('Ctrl Pts',(-3.81963214137809,-4.77608387295123,4.11435060469935));
#9059=CARTESIAN_POINT('Ctrl Pts',(-3.68434834364815,-4.87825817737819,4.12207363966038));
#9060=CARTESIAN_POINT('Ctrl Pts',(-3.54902859337836,-4.98045963528407,4.12979872706765));
#9061=CARTESIAN_POINT('Ctrl Pts',(-3.4094618921013,-5.07702093017004,4.13752381447492));
#9062=CARTESIAN_POINT('Ctrl Pts',(-3.26614129816218,-5.16760549799803,4.14524890188219));
#9063=CARTESIAN_POINT('Ctrl Pts',(-3.12337645338244,-5.25783880927565,4.15294403399333));
#9064=CARTESIAN_POINT('Ctrl Pts',(-2.97688705798117,-5.34214152303887,4.16063916610447));
#9065=CARTESIAN_POINT('Ctrl Pts',(-2.82718724591767,-5.420224888233,4.16833429821561));
#9066=CARTESIAN_POINT('Ctrl Pts',(-2.6769110169479,-5.49860891226682,4.17605906031882));
#9067=CARTESIAN_POINT('Ctrl Pts',(-2.52334636165946,-5.57075333230414,4.18378382242203));
#9068=CARTESIAN_POINT('Ctrl Pts',(-2.36703049156718,-5.63639886935721,4.19150858452525));
#9069=CARTESIAN_POINT('Ctrl Pts',(-2.21074511381998,-5.70203160101588,4.19923183976859));
#9070=CARTESIAN_POINT('Ctrl Pts',(-2.05170988415776,-5.76116785662558,4.20695509501193));
#9071=CARTESIAN_POINT('Ctrl Pts',(-1.89048263592708,-5.81359621626392,4.21467835025528));
#9072=CARTESIAN_POINT('Ctrl Pts',(-1.72924915703758,-5.86602660200657,4.22240190396534));
#9073=CARTESIAN_POINT('Ctrl Pts',(-1.56582379022629,-5.911748471275,4.23012545767541));
#9074=CARTESIAN_POINT('Ctrl Pts',(-1.40078094924048,-5.95059982646665,4.23784901138547));
#9075=CARTESIAN_POINT('Ctrl Pts',(-1.23574919328105,-5.98944857222493,4.24557204634661));
#9076=CARTESIAN_POINT('Ctrl Pts',(-1.06910048907319,-6.02142765473253,4.25329508130775));
#9077=CARTESIAN_POINT('Ctrl Pts',(-0.901421079249796,-6.04642585337686,
4.26101811626889));
#9078=CARTESIAN_POINT('Ctrl Pts',(-0.73369710754433,-6.07143069545334,4.26874320367626));
#9079=CARTESIAN_POINT('Ctrl Pts',(-0.564942196233197,-6.0894508975762,4.27646829108363));
#9080=CARTESIAN_POINT('Ctrl Pts',(-0.395750334799665,-6.10042680760994,
4.28419337849101));
#9081=CARTESIAN_POINT('Ctrl Pts',(-0.227214542631636,-6.11136015674758,
4.2918885106016));
#9082=CARTESIAN_POINT('Ctrl Pts',(-0.0582454966302977,-6.11530375944402,
4.2995836427122));
#9083=CARTESIAN_POINT('Ctrl Pts',(0.110567181803888,-6.11225003258276,4.3072787748228));
#9084=CARTESIAN_POINT('Ctrl Pts',(0.280029870964719,-6.10918454739129,4.31500353692601));
#9085=CARTESIAN_POINT('Ctrl Pts',(0.449395004085272,-6.09906662372046,4.32272829902921));
#9086=CARTESIAN_POINT('Ctrl Pts',(0.61806679505976,-6.08192559962259,4.33045306113242));
#9087=CARTESIAN_POINT('Ctrl Pts',(0.786705683434824,-6.06478791920327,4.33817631637576));
#9088=CARTESIAN_POINT('Ctrl Pts',(0.954651184423808,-6.04062990399549,4.3458995716191));
#9089=CARTESIAN_POINT('Ctrl Pts',(1.1213123005287,-6.00953278443366,4.35362282686244));
#9090=CARTESIAN_POINT('Ctrl Pts',(1.28797985728529,-5.97843446311752,4.3613463805725));
#9091=CARTESIAN_POINT('Ctrl Pts',(1.45336261756681,-5.94039655507275,4.36906993428256));
#9092=CARTESIAN_POINT('Ctrl Pts',(1.61687866927581,-5.8955516223116,4.37679348799262));
#9093=CARTESIAN_POINT('Ctrl Pts',(1.78038373850458,-5.85070970153968,4.38451652295376));
#9094=CARTESIAN_POINT('Ctrl Pts',(1.94202204439148,-5.79906175480238,4.39223955791489));
#9095=CARTESIAN_POINT('Ctrl Pts',(2.10122558078278,-5.74079059199724,4.39996259287603));
#9096=CARTESIAN_POINT('Ctrl Pts',(2.26047142653828,-5.68250394325564,4.4076876802834));
#9097=CARTESIAN_POINT('Ctrl Pts',(2.41728091124755,-5.61759066817747,4.41541276769077));
#9098=CARTESIAN_POINT('Ctrl Pts',(2.57110389791294,-5.54628256660593,4.42313785509814));
#9099=CARTESIAN_POINT('Ctrl Pts',(2.7243304106525,-5.47525097392432,4.43083298720876));
#9100=CARTESIAN_POINT('Ctrl Pts',(2.87459327577343,-5.39787422111947,4.43852811931937));
#9101=CARTESIAN_POINT('Ctrl Pts',(3.02137110334711,-5.31442774138091,4.44622325142999));
#9102=CARTESIAN_POINT('Ctrl Pts',(3.16871553818466,-5.23065913273266,4.45394808910188));
#9103=CARTESIAN_POINT('Ctrl Pts',(3.31260014595631,-5.14074414708694,4.46167292677376));
#9104=CARTESIAN_POINT('Ctrl Pts',(3.45251577270222,-5.04499359779003,4.46939776444565));
#9105=CARTESIAN_POINT('Ctrl Pts',(3.54440943264835,-4.98210663783149,4.47447127640903));
#9106=CARTESIAN_POINT('Ctrl Pts',(3.63459155151057,-4.91670339231516,4.47954478837242));
#9107=CARTESIAN_POINT('Ctrl Pts',(3.72292453512037,-4.84888218750453,4.4846183003358));
#9108=CARTESIAN_POINT('Ctrl Pts',(3.72292453512037,-4.84888218750454,2.73461001778677));
#9109=CARTESIAN_POINT('Ctrl Pts',(3.85742670434484,-4.74561273147958,2.74233503114518));
#9110=CARTESIAN_POINT('Ctrl Pts',(3.98762056731902,-4.63675019710229,2.75006004450358));
#9111=CARTESIAN_POINT('Ctrl Pts',(4.11305073883802,-4.52268053064154,2.75778505786199));
#9112=CARTESIAN_POINT('Ctrl Pts',(4.22727439585806,-4.41880237835639,2.76481988262257));
#9113=CARTESIAN_POINT('Ctrl Pts',(4.33754781035837,-4.31060659422731,2.77185470738315));
#9114=CARTESIAN_POINT('Ctrl Pts',(4.44355277819139,-4.19841211292169,2.77888953214373));
#9115=CARTESIAN_POINT('Ctrl Pts',(4.55995413570729,-4.07521420817501,2.78661429418798));
#9116=CARTESIAN_POINT('Ctrl Pts',(4.67124943892527,-3.94715064688156,2.79433905623222));
#9117=CARTESIAN_POINT('Ctrl Pts',(4.77704270982733,-3.81466754920865,2.80206381827647));
#9118=CARTESIAN_POINT('Ctrl Pts',(4.88281534375428,-3.68221029486554,2.80978707346002));
#9119=CARTESIAN_POINT('Ctrl Pts',(4.98308788929193,-3.54533547187285,2.81751032864357));
#9120=CARTESIAN_POINT('Ctrl Pts',(5.07750478792242,-3.40452209438049,2.82523358382712));
#9121=CARTESIAN_POINT('Ctrl Pts',(5.17192533530416,-3.26370327513993,2.8329571374767));
#9122=CARTESIAN_POINT('Ctrl Pts',(5.26048960316994,-3.11894585784414,2.84068069112628));
#9123=CARTESIAN_POINT('Ctrl Pts',(5.34288505882612,-2.97075828883344,2.84840424477586));
#9124=CARTESIAN_POINT('Ctrl Pts',(5.42527498042637,-2.82258067277815,2.85612727967622));
#9125=CARTESIAN_POINT('Ctrl Pts',(5.50149676492954,-2.67097364306444,2.86385031457659));
#9126=CARTESIAN_POINT('Ctrl Pts',(5.57128350479845,-2.5164708763784,2.87157334947695));
#9127=CARTESIAN_POINT('Ctrl Pts',(5.64108879094418,-2.3619270495843,2.87929843682372));
#9128=CARTESIAN_POINT('Ctrl Pts',(5.7044554826127,-2.20448623618459,2.88702352417049));
#9129=CARTESIAN_POINT('Ctrl Pts',(5.76116417231926,-2.04470363184618,2.89474861151725));
#9130=CARTESIAN_POINT('Ctrl Pts',(5.81765296740604,-1.88554060336482,2.90244374392848));
#9131=CARTESIAN_POINT('Ctrl Pts',(5.86753522907989,-1.72405421779254,2.9101388763397));
#9132=CARTESIAN_POINT('Ctrl Pts',(5.91064283593141,-1.56080967082881,2.91783400875093));
#9133=CARTESIAN_POINT('Ctrl Pts',(5.95391642647975,-1.39693655885368,2.92555877088689));
#9134=CARTESIAN_POINT('Ctrl Pts',(5.99037838488768,-1.23123367253846,2.93328353302285));
#9135=CARTESIAN_POINT('Ctrl Pts',(6.0198944294592,-1.06428220912787,2.94100829515882));
#9136=CARTESIAN_POINT('Ctrl Pts',(6.04940471637381,-0.897363312724832,2.94873155043535));
#9137=CARTESIAN_POINT('Ctrl Pts',(6.07197173788201,-0.729196637109618,2.95645480571189));
#9138=CARTESIAN_POINT('Ctrl Pts',(6.08751244314942,-0.560372926720169,2.96417806098842));
#9139=CARTESIAN_POINT('Ctrl Pts',(6.10305374899113,-0.391542692097803,2.97190161473202));
#9140=CARTESIAN_POINT('Ctrl Pts',(6.11156816224163,-0.22205568711227,2.97962516847561));
#9141=CARTESIAN_POINT('Ctrl Pts',(6.11302449538673,-0.0525079165631778,
2.9873487222192));
#9142=CARTESIAN_POINT('Ctrl Pts',(6.11448073071791,0.117028466390709,2.99507175721399));
#9143=CARTESIAN_POINT('Ctrl Pts',(6.1088798318847,0.286625289795099,3.00279479220878));
#9144=CARTESIAN_POINT('Ctrl Pts',(6.09624274694914,0.455686221834749,3.01051782720356));
#9145=CARTESIAN_POINT('Ctrl Pts',(6.08360230362713,0.624792082902369,3.01824291464448));
#9146=CARTESIAN_POINT('Ctrl Pts',(6.06392195913237,0.793361451592205,3.02596800208539));
#9147=CARTESIAN_POINT('Ctrl Pts',(6.03727466787266,0.960801825124741,3.03369308952631));
#9148=CARTESIAN_POINT('Ctrl Pts',(6.01073070655698,1.12759291673757,3.04138822147024));
#9149=CARTESIAN_POINT('Ctrl Pts',(5.97727381465468,1.29326345017323,3.04908335341418));
#9150=CARTESIAN_POINT('Ctrl Pts',(5.9370267664945,1.45723667824685,3.05677848535811));
#9151=CARTESIAN_POINT('Ctrl Pts',(5.89662474686772,1.62184128608116,3.0645032474473));
#9152=CARTESIAN_POINT('Ctrl Pts',(5.84936583776353,1.78479378253571,3.07222800953649));
#9153=CARTESIAN_POINT('Ctrl Pts',(5.79541018467373,1.9455195588531,3.07995277162568));
#9154=CARTESIAN_POINT('Ctrl Pts',(5.7414650566483,2.10621398258659,3.08767602685482));
#9155=CARTESIAN_POINT('Ctrl Pts',(5.6808258920245,2.26468225262756,3.09539928208395));
#9156=CARTESIAN_POINT('Ctrl Pts',(5.61370239110768,2.42036588692122,3.10312253731309));
#9157=CARTESIAN_POINT('Ctrl Pts',(5.54657629619104,2.57605553763705,3.11084609100882));
#9158=CARTESIAN_POINT('Ctrl Pts',(5.47296548537579,2.72896004467673,3.11856964470455));
#9159=CARTESIAN_POINT('Ctrl Pts',(5.39312771821359,2.87854111965354,3.12629319840029));
#9160=CARTESIAN_POINT('Ctrl Pts',(5.31329531331895,3.02811214808504,3.13401623334702));
#9161=CARTESIAN_POINT('Ctrl Pts',(5.22723693827673,3.1743599115294,3.14173926829376));
#9162=CARTESIAN_POINT('Ctrl Pts',(5.13525629070301,3.31677077762319,3.1494623032405));
#9163=CARTESIAN_POINT('Ctrl Pts',(5.04325119867929,3.45921949032262,3.15718739063356));
#9164=CARTESIAN_POINT('Ctrl Pts',(4.9453208593657,3.59782900050773,3.16491247802662));
#9165=CARTESIAN_POINT('Ctrl Pts',(4.84181280658558,3.73211391954799,3.17263756541967));
#9166=CARTESIAN_POINT('Ctrl Pts',(4.73870612215536,3.86587812821911,3.18033269760155));
#9167=CARTESIAN_POINT('Ctrl Pts',(4.63006512036532,3.9953509970781,3.18802782978343));
#9168=CARTESIAN_POINT('Ctrl Pts',(4.51627354531815,4.12008480815134,3.19572296196531));
#9169=CARTESIAN_POINT('Ctrl Pts',(4.40204381848931,4.24529890382852,3.20344772407255));
#9170=CARTESIAN_POINT('Ctrl Pts',(4.28258329639064,4.36578170088513,3.21117248617979));
#9171=CARTESIAN_POINT('Ctrl Pts',(4.15830751659645,4.48110523865681,3.21889724828703));
#9172=CARTESIAN_POINT('Ctrl Pts',(4.03405597912532,4.59640628040822,3.22662050353445));
#9173=CARTESIAN_POINT('Ctrl Pts',(3.90499129038211,4.70654985557746,3.23434375878188));
#9174=CARTESIAN_POINT('Ctrl Pts',(3.77156478783028,4.81114587325085,3.2420670140293));
#9175=CARTESIAN_POINT('Ctrl Pts',(3.63813312898482,4.91574593305808,3.24979056774346));
#9176=CARTESIAN_POINT('Ctrl Pts',(3.50033956599702,5.01479780772929,3.25751412145761));
#9177=CARTESIAN_POINT('Ctrl Pts',(3.35866797716767,5.10795213188695,3.26523767517177));
#9178=CARTESIAN_POINT('Ctrl Pts',(3.21700590364524,5.20110019937739,3.272960710137));
#9179=CARTESIAN_POINT('Ctrl Pts',(3.07146659035469,5.28835133489436,3.28068374510223));
#9180=CARTESIAN_POINT('Ctrl Pts',(2.92256245884773,5.36939980227157,3.28840678006746));
#9181=CARTESIAN_POINT('Ctrl Pts',(2.77361875511016,5.45046980880023,3.2961318674789));
#9182=CARTESIAN_POINT('Ctrl Pts',(2.62130872380104,5.52533369975343,3.30385695489035));
#9183=CARTESIAN_POINT('Ctrl Pts',(2.46616976756211,5.59373151304768,3.31158204230179));
#9184=CARTESIAN_POINT('Ctrl Pts',(2.31163238862835,5.66186410235693,3.31927717439202));
#9185=CARTESIAN_POINT('Ctrl Pts',(2.15428828368925,5.72358057502088,3.32697230648224));
#9186=CARTESIAN_POINT('Ctrl Pts',(1.99468862981037,5.77867137260852,3.33466743857247));
#9187=CARTESIAN_POINT('Ctrl Pts',(1.83447443939561,5.8339742966456,3.34239220067569));
#9188=CARTESIAN_POINT('Ctrl Pts',(1.67193054273701,5.88261997842296,3.35011696277891));
#9189=CARTESIAN_POINT('Ctrl Pts',(1.50762658312358,5.92443141983761,3.35784172488213));
#9190=CARTESIAN_POINT('Ctrl Pts',(1.34335467408245,5.96623470514556,3.36556498012546));
#9191=CARTESIAN_POINT('Ctrl Pts',(1.17732369411053,6.0012063320846,3.3732882353688));
#9192=CARTESIAN_POINT('Ctrl Pts',(1.01011660531776,6.02921968468237,3.38101149061213));
#9193=CARTESIAN_POINT('Ctrl Pts',(0.842903054773498,6.05723411986177,3.38873504432221));
#9194=CARTESIAN_POINT('Ctrl Pts',(0.674513616365418,6.07828968633435,3.39645859803229));
#9195=CARTESIAN_POINT('Ctrl Pts',(0.505540342874708,6.09231109877246,3.40418215174237));
#9196=CARTESIAN_POINT('Ctrl Pts',(0.336578418395957,6.10633156946887,3.41190518670353));
#9197=CARTESIAN_POINT('Ctrl Pts',(0.167033053178525,6.11331880536751,3.41962822166468));
#9198=CARTESIAN_POINT('Ctrl Pts',(-0.00249950891330681,6.11324948901607,
3.42735125662584));
#9199=CARTESIAN_POINT('Ctrl Pts',(-0.172077125374675,6.11318015424336,3.43507634403325));
#9200=CARTESIAN_POINT('Ctrl Pts',(-0.341641614760534,6.10605051781757,3.44280143144066));
#9201=CARTESIAN_POINT('Ctrl Pts',(-0.510596696319146,6.09188940938753,3.45052651884806));
#9202=CARTESIAN_POINT('Ctrl Pts',(-0.678896626763082,6.07778321298433,3.4582216509586));
#9203=CARTESIAN_POINT('Ctrl Pts',(-0.84659155873096,6.05670003721768,3.46591678306913));
#9204=CARTESIAN_POINT('Ctrl Pts',(-1.01309723036588,6.02871956258748,3.47361191517967));
#9205=CARTESIAN_POINT('Ctrl Pts',(-1.18024402960935,6.00063134955649,3.48133667728178));
#9206=CARTESIAN_POINT('Ctrl Pts',(-1.34625158532875,5.96558263870925,3.48906143938389));
#9207=CARTESIAN_POINT('Ctrl Pts',(-1.51053499781256,5.92369053740009,3.496786201486));
#9208=CARTESIAN_POINT('Ctrl Pts',(-1.67478636373223,5.88180660793185,3.50450945672822));
#9209=CARTESIAN_POINT('Ctrl Pts',(-1.83731395059546,5.83308202993113,3.51223271197044));
#9210=CARTESIAN_POINT('Ctrl Pts',(-1.99754526737113,5.77768452472988,3.51995596721266));
#9211=CARTESIAN_POINT('Ctrl Pts',(-2.15778277631777,5.72228487868108,3.52767952092162));
#9212=CARTESIAN_POINT('Ctrl Pts',(-2.31572353678688,5.66021188921617,3.53540307463057));
#9213=CARTESIAN_POINT('Ctrl Pts',(-2.47081163307323,5.59168270168918,3.54312662833952));
#9214=CARTESIAN_POINT('Ctrl Pts',(-2.62588931293904,5.5231581168935,3.55084966329954));
#9215=CARTESIAN_POINT('Ctrl Pts',(-2.77811442212812,5.44817832990716,3.55857269825957));
#9216=CARTESIAN_POINT('Ctrl Pts',(-2.92695222758717,5.36700812556889,3.5662957332196));
#9217=CARTESIAN_POINT('Ctrl Pts',(-3.07582958765062,5.28581634972659,3.57402082062585));
#9218=CARTESIAN_POINT('Ctrl Pts',(-3.22131756569114,5.19843101907086,3.5817459080321));
#9219=CARTESIAN_POINT('Ctrl Pts',(-3.3629063449619,5.10516272781926,3.58947099543836));
#9220=CARTESIAN_POINT('Ctrl Pts',(-3.50394609057995,5.01225609962381,3.59716612755453));
#9221=CARTESIAN_POINT('Ctrl Pts',(-3.64111658026085,4.91351225267007,3.60486125967069));
#9222=CARTESIAN_POINT('Ctrl Pts',(-3.77394287989615,4.80928068444556,3.61255639178686));
#9223=CARTESIAN_POINT('Ctrl Pts',(-3.9072806251576,4.70464777416891,3.62028115389102));
#9224=CARTESIAN_POINT('Ctrl Pts',(-4.03628786521529,4.59444771647263,3.62800591599518));
#9225=CARTESIAN_POINT('Ctrl Pts',(-4.16050701194673,4.47906317950998,3.63573067809934));
#9226=CARTESIAN_POINT('Ctrl Pts',(-4.28470192740124,4.36370115046775,3.64345393334361));
#9227=CARTESIAN_POINT('Ctrl Pts',(-4.40411038114396,4.24315687568503,3.65117718858788));
#9228=CARTESIAN_POINT('Ctrl Pts',(-4.51830989664579,4.11785153209446,3.65890044383215));
#9229=CARTESIAN_POINT('Ctrl Pts',(-4.63251382541117,3.99254134605335,3.66662399754319));
#9230=CARTESIAN_POINT('Ctrl Pts',(-4.74150819671914,3.86246995459035,3.67434755125424));
#9231=CARTESIAN_POINT('Ctrl Pts',(-4.84490873516459,3.72809400504143,3.68207110496528));
#9232=CARTESIAN_POINT('Ctrl Pts',(-4.94830232876042,3.59372708079137,3.68979413992739));
#9233=CARTESIAN_POINT('Ctrl Pts',(-5.04610264805784,3.45505642822008,3.6975171748895));
#9234=CARTESIAN_POINT('Ctrl Pts',(-5.13796681081408,3.31257039373852,3.70524020985161));
#9235=CARTESIAN_POINT('Ctrl Pts',(-5.22985538706272,3.17004649267641,3.71296529725996));
#9236=CARTESIAN_POINT('Ctrl Pts',(-5.31580448071359,3.02370544893328,3.7206903846683));
#9237=CARTESIAN_POINT('Ctrl Pts',(-5.39551500572968,2.87406391464175,3.72841547207665));
#9238=CARTESIAN_POINT('Ctrl Pts',(-5.47491644001749,2.72500264011901,3.73611060418245));
#9239=CARTESIAN_POINT('Ctrl Pts',(-5.54812748350642,2.57266671663333,3.74380573628825));
#9240=CARTESIAN_POINT('Ctrl Pts',(-5.61489829397816,2.41759026941729,3.75150086839405));
#9241=CARTESIAN_POINT('Ctrl Pts',(-5.68165926002252,2.26253668606663,3.75919486595964));
#9242=CARTESIAN_POINT('Ctrl Pts',(-5.74200723500789,2.10468435679823,3.76688886352523));
#9243=CARTESIAN_POINT('Ctrl Pts',(-5.79572429309673,1.94458362661738,3.77458286109083));
#9244=CARTESIAN_POINT('Ctrl Pts',(-5.84943543818212,1.78450051981731,3.78227601172556));
#9245=CARTESIAN_POINT('Ctrl Pts',(-5.89651701651356,1.62216980979388,3.78996916236029));
#9246=CARTESIAN_POINT('Ctrl Pts',(-5.93680028371151,1.4581590975689,3.79766231299503));
#9247=CARTESIAN_POINT('Ctrl Pts',(-5.97707810581009,1.29417055471316,3.80535442374466));
#9248=CARTESIAN_POINT('Ctrl Pts',(-6.01055937518844,1.12850277583631,3.81304653449429));
#9249=CARTESIAN_POINT('Ctrl Pts',(-6.03712593207551,0.961735952723713,3.82073864524391));
#9250=CARTESIAN_POINT('Ctrl Pts',(-6.06369690572731,0.794941404158186,3.82843203482857));
#9251=CARTESIAN_POINT('Ctrl Pts',(-6.08335081641304,0.627047763945297,3.83612542441322));
#9252=CARTESIAN_POINT('Ctrl Pts',(-6.09602096456547,0.458643611182269,3.84381881399787));
#9253=CARTESIAN_POINT('Ctrl Pts',(-6.10750647886695,0.305984914399864,3.85079288683731));
#9254=CARTESIAN_POINT('Ctrl Pts',(-6.11325373677083,0.152906976817679,3.85776695967675));
#9255=CARTESIAN_POINT('Ctrl Pts',(-6.11324999817629,-0.000149323895543098,
3.86474103251618));
#9256=CARTESIAN_POINT('Origin',(0.,0.,-3.86474103256053));
#9257=CARTESIAN_POINT('',(3.72318137141383,-4.84921626688776,0.984617815426764));
#9258=CARTESIAN_POINT('',(3.72292453512038,-4.84888218750453,1.13013653271955));
#9259=CARTESIAN_POINT('',(3.72292453512038,-4.84888218750453,-3.86474103256053));
#9260=CARTESIAN_POINT('',(-6.11286162838407,-0.000127878758945515,0.364741032560545));
#9261=CARTESIAN_POINT('Ctrl Pts',(-6.11286162838407,-0.000127878758945515,
0.364741032560545));
#9262=CARTESIAN_POINT('Ctrl Pts',(-6.11309733150939,-0.381299532825294,
0.382105164980884));
#9263=CARTESIAN_POINT('Ctrl Pts',(-5.98437783201522,-1.77899319463741,0.445784122936951));
#9264=CARTESIAN_POINT('Ctrl Pts',(-4.93150710543191,-4.0362823909247,0.555777906428748));
#9265=CARTESIAN_POINT('Ctrl Pts',(-2.39941005850561,-5.9036730620091,0.694722383035934));
#9266=CARTESIAN_POINT('Ctrl Pts',(0.717505479260219,-6.33215256902002,0.833666859643123));
#9267=CARTESIAN_POINT('Ctrl Pts',(2.76360922605899,-5.55669049096136,0.930298670440064));
#9268=CARTESIAN_POINT('Ctrl Pts',(3.65355952202664,-4.9027500092498,0.980615655701276));
#9269=CARTESIAN_POINT('Ctrl Pts',(3.72318137141383,-4.84921626688776,0.984617815426764));
#9270=CARTESIAN_POINT('',(-1.5788818818754,5.90584097022478,0.));
#9271=CARTESIAN_POINT('Ctrl Pts',(-1.5788818818754,5.90584097022478,0.));
#9272=CARTESIAN_POINT('Ctrl Pts',(-2.56095449565812,5.64329129027149,0.0463148255357291));
#9273=CARTESIAN_POINT('Ctrl Pts',(-4.39060121268314,4.61907415016922,0.138944476607187));
#9274=CARTESIAN_POINT('Ctrl Pts',(-5.8560845614411,2.28791808963582,0.260524820794035));
#9275=CARTESIAN_POINT('Ctrl Pts',(-6.11246864768786,0.635388098315462,0.335790339445155));
#9276=CARTESIAN_POINT('Ctrl Pts',(-6.11286162838407,-0.000127878758945515,
0.364741032560545));
#9277=CARTESIAN_POINT('',(1.57893355462654,5.90582715566367,0.));
#9278=CARTESIAN_POINT('Origin',(0.,0.,0.));
#9279=CARTESIAN_POINT('',(-6.11324999799714,-0.000156486230825092,0.510258967478569));
#9280=CARTESIAN_POINT('Ctrl Pts',(1.57893355462654,5.90582715566367,-4.44089209850063E-16));
#9281=CARTESIAN_POINT('Ctrl Pts',(1.41553753480309,5.94951137661894,0.00770829872622793));
#9282=CARTESIAN_POINT('Ctrl Pts',(1.25029716222687,5.98641851155851,0.0154165974524564));
#9283=CARTESIAN_POINT('Ctrl Pts',(1.08379079859978,6.01641280726069,0.0231248961786847));
#9284=CARTESIAN_POINT('Ctrl Pts',(0.917316661967493,6.04640129762312,0.0308317029781331));
#9285=CARTESIAN_POINT('Ctrl Pts',(0.749577337565903,6.06947956174143,0.0385385097775815));
#9286=CARTESIAN_POINT('Ctrl Pts',(0.581160905815119,6.08556304412765,0.0462453165770298));
#9287=CARTESIAN_POINT('Ctrl Pts',(0.412739059075133,6.10164704363611,0.053952371168663));
#9288=CARTESIAN_POINT('Ctrl Pts',(0.243640379249169,6.11073577750831,0.0616594257602958));
#9289=CARTESIAN_POINT('Ctrl Pts',(0.0744583243935386,6.11279653844527,0.0693664803519289));
#9290=CARTESIAN_POINT('Ctrl Pts',(-0.0947158388586656,6.11485720325674,
0.0770731754431501));
#9291=CARTESIAN_POINT('Ctrl Pts',(-0.263973049736742,6.10989054820349,0.0847798705343731));
#9292=CARTESIAN_POINT('Ctrl Pts',(-0.432719396652683,6.09791599534304,0.0924865656255944));
#9293=CARTESIAN_POINT('Ctrl Pts',(-0.601506554892215,6.0859385464356,0.100195124581918));
#9294=CARTESIAN_POINT('Ctrl Pts',(-0.769782283310316,6.06694983542276,0.107903683538241));
#9295=CARTESIAN_POINT('Ctrl Pts',(-0.936956493901048,6.04102127881012,0.115612242494564));
#9296=CARTESIAN_POINT('Ctrl Pts',(-1.04775886705582,6.02383593906779,0.12072144338713));
#9297=CARTESIAN_POINT('Ctrl Pts',(-1.15807744082288,6.00360300632556,0.125830644279697));
#9298=CARTESIAN_POINT('Ctrl Pts',(-1.2677424668155,5.98035572523345,0.130939845172263));
#9299=CARTESIAN_POINT('Ctrl Pts',(-1.433546794107,5.94520778478531,0.138664528673874));
#9300=CARTESIAN_POINT('Ctrl Pts',(-1.59791786096845,5.9031540298198,0.146389212175485));
#9301=CARTESIAN_POINT('Ctrl Pts',(-1.76027626943888,5.85433625765982,0.154113895677096));
#9302=CARTESIAN_POINT('Ctrl Pts',(-1.92260304000586,5.80552799835462,0.161837073911484));
#9303=CARTESIAN_POINT('Ctrl Pts',(-2.08291763142132,5.74995844307731,0.16956025214587));
#9304=CARTESIAN_POINT('Ctrl Pts',(-2.24065518922987,5.68781943151128,0.177283430380257));
#9305=CARTESIAN_POINT('Ctrl Pts',(-2.39839890908997,5.62567799247142,0.18500691032226));
#9306=CARTESIAN_POINT('Ctrl Pts',(-2.55356509756797,5.55696669608266,0.192730390264264));
#9307=CARTESIAN_POINT('Ctrl Pts',(-2.7056075559911,5.48192605891979,0.200453870206266));
#9308=CARTESIAN_POINT('Ctrl Pts',(-2.85763984024223,5.40689044322499,0.208176833318864));
#9309=CARTESIAN_POINT('Ctrl Pts',(-3.00654852851301,5.32552647462806,0.215899796431462));
#9310=CARTESIAN_POINT('Ctrl Pts',(-3.15181060588922,5.23812136811512,0.22362275954406));
#9311=CARTESIAN_POINT('Ctrl Pts',(-3.29711136203908,5.15069298834055,0.231347779041556));
#9312=CARTESIAN_POINT('Ctrl Pts',(-3.43876329415943,5.05722041799664,0.239072798539052));
#9313=CARTESIAN_POINT('Ctrl Pts',(-3.57627022355895,4.95803558383616,0.246797818036548));
#9314=CARTESIAN_POINT('Ctrl Pts',(-3.71325172206461,4.85922974712911,0.254493319284182));
#9315=CARTESIAN_POINT('Ctrl Pts',(-3.84611960496846,4.75475543331657,0.262188820531816));
#9316=CARTESIAN_POINT('Ctrl Pts',(-3.97441411774349,4.64498202183617,0.269884321779451));
#9317=CARTESIAN_POINT('Ctrl Pts',(-4.10319053334657,4.53479627691848,0.277608729047571));
#9318=CARTESIAN_POINT('Ctrl Pts',(-4.22740488074,4.419232384039,0.285333136315691));
#9319=CARTESIAN_POINT('Ctrl Pts',(-4.34661622458183,4.29869200556425,0.293057543583811));
#9320=CARTESIAN_POINT('Ctrl Pts',(-4.46580422246066,4.17817523332633,0.300780438129061));
#9321=CARTESIAN_POINT('Ctrl Pts',(-4.57999094901574,4.05268414536578,0.308503332674311));
#9322=CARTESIAN_POINT('Ctrl Pts',(-4.68877217920449,3.92265739187326,0.31622622721956));
#9323=CARTESIAN_POINT('Ctrl Pts',(-4.79755753321199,3.7926257091594,0.323949414534226));
#9324=CARTESIAN_POINT('Ctrl Pts',(-4.90093677434673,3.65805825740187,0.331672601848891));
#9325=CARTESIAN_POINT('Ctrl Pts',(-4.99854534658632,3.51942750751032,0.339395789163556));
#9326=CARTESIAN_POINT('Ctrl Pts',(-5.09614733242753,3.38080611209782,0.347118455335588));
#9327=CARTESIAN_POINT('Ctrl Pts',(-5.18797924609181,3.23812222643966,0.354841121507622));
#9328=CARTESIAN_POINT('Ctrl Pts',(-5.27371923011663,3.09187823893472,0.362563787679654));
#9329=CARTESIAN_POINT('Ctrl Pts',(-5.35948199583808,2.9455953934081,0.370288505816589));
#9330=CARTESIAN_POINT('Ctrl Pts',(-5.43914943511072,2.79575082835339,0.378013223953523));
#9331=CARTESIAN_POINT('Ctrl Pts',(-5.51244464647516,2.64287335717159,0.385737942090457));
#9332=CARTESIAN_POINT('Ctrl Pts',(-5.5854764025778,2.49054539493372,0.393434894189186));
#9333=CARTESIAN_POINT('Ctrl Pts',(-5.65218155735735,2.33520658914986,0.401131846287916));
#9334=CARTESIAN_POINT('Ctrl Pts',(-5.71233296231532,2.17740159138041,0.408828798386645));
#9335=CARTESIAN_POINT('Ctrl Pts',(-5.77255257252794,2.01941765963484,0.416534478005176));
#9336=CARTESIAN_POINT('Ctrl Pts',(-5.82622593648816,1.85890309650743,0.424240157623708));
#9337=CARTESIAN_POINT('Ctrl Pts',(-5.87315835556509,1.69641872571483,0.431945837242239));
#9338=CARTESIAN_POINT('Ctrl Pts',(-5.92008371072521,1.53395881085486,0.439650357059488));
#9339=CARTESIAN_POINT('Ctrl Pts',(-5.96027005446787,1.36952998661637,0.447354876876737));
#9340=CARTESIAN_POINT('Ctrl Pts',(-5.99357258088567,1.20370813744675,0.455059396693986));
#9341=CARTESIAN_POINT('Ctrl Pts',(-6.02687058901322,1.03790878600701,0.462762871207455));
#9342=CARTESIAN_POINT('Ctrl Pts',(-6.05328658190003,0.870717100760946,0.470466345720923));
#9343=CARTESIAN_POINT('Ctrl Pts',(-6.0727268179118,0.7027194016923,0.478169820234392));
#9344=CARTESIAN_POINT('Ctrl Pts',(-6.09216822287533,0.534711600832463,0.48587375796189));
#9345=CARTESIAN_POINT('Ctrl Pts',(-6.1046329952404,0.36589800713182,0.493577695689388));
#9346=CARTESIAN_POINT('Ctrl Pts',(-6.11007916304154,0.196870982792384,0.501281633416886));
#9347=CARTESIAN_POINT('Ctrl Pts',(-6.11219462092914,0.131215724836038,0.504274078091075));
#9348=CARTESIAN_POINT('Ctrl Pts',(-6.11325167937916,0.0655283026476351,
0.507266522765266));
#9349=CARTESIAN_POINT('Ctrl Pts',(-6.11324999799716,-0.000156485372245552,
0.510258967439455));
#9350=CARTESIAN_POINT('Ctrl Pts',(-6.11324999799714,-0.000156486230820938,
0.510258967478568));
#9351=CARTESIAN_POINT('Ctrl Pts',(-6.11324545367516,-0.177683775470678,
0.518346693833848));
#9352=CARTESIAN_POINT('Ctrl Pts',(-6.10550354738073,-0.355172525646239,
0.526434420189127));
#9353=CARTESIAN_POINT('Ctrl Pts',(-6.09006029727742,-0.531969113788794,
0.534522146544405));
#9354=CARTESIAN_POINT('Ctrl Pts',(-6.0816260978578,-0.628525063548642,0.538939189360876));
#9355=CARTESIAN_POINT('Ctrl Pts',(-6.07089572361351,-0.724874613800565,
0.543356232177347));
#9356=CARTESIAN_POINT('Ctrl Pts',(-6.05788157683862,-0.820911909707277,
0.547773274993818));
#9357=CARTESIAN_POINT('Ctrl Pts',(-6.03512235647263,-0.988862526732028,
0.555497826788483));
#9358=CARTESIAN_POINT('Ctrl Pts',(-6.00537031896867,-1.15589589163436,0.563222378583147));
#9359=CARTESIAN_POINT('Ctrl Pts',(-5.96872389633741,-1.32142370638293,0.570946930377813));
#9360=CARTESIAN_POINT('Ctrl Pts',(-5.93208463577432,-1.4869191708662,0.57866997250898));
#9361=CARTESIAN_POINT('Ctrl Pts',(-5.88855374713308,-1.65090936302899,0.586393014640148));
#9362=CARTESIAN_POINT('Ctrl Pts',(-5.83828064561057,-1.81281677661836,0.594116056771316));
#9363=CARTESIAN_POINT('Ctrl Pts',(-5.78800561639362,-1.97473039845849,0.601839395038287));
#9364=CARTESIAN_POINT('Ctrl Pts',(-5.73098794716263,-2.13456077803919,0.60956273330526));
#9365=CARTESIAN_POINT('Ctrl Pts',(-5.66742697942247,-2.29174540370746,0.617286071572231));
#9366=CARTESIAN_POINT('Ctrl Pts',(-5.60387028783684,-2.44891945455645,0.625008890240635));
#9367=CARTESIAN_POINT('Ctrl Pts',(-5.53377129750875,-2.60344781381839,0.632731708909037));
#9368=CARTESIAN_POINT('Ctrl Pts',(-5.45737763912667,-2.7547876263807,0.64045452757744));
#9369=CARTESIAN_POINT('Ctrl Pts',(-5.38096367159313,-2.90616767242888,0.648179399346812));
#9370=CARTESIAN_POINT('Ctrl Pts',(-5.29825183307229,-3.05435719378608,0.655904271116186));
#9371=CARTESIAN_POINT('Ctrl Pts',(-5.20953633294877,-3.19883678204854,0.663629142885557));
#9372=CARTESIAN_POINT('Ctrl Pts',(-5.12115007746558,-3.34278017167597,0.671325345790709));
#9373=CARTESIAN_POINT('Ctrl Pts',(-5.02680483702586,-3.48304086855312,0.679021548695858));
#9374=CARTESIAN_POINT('Ctrl Pts',(-4.92683498489223,-3.61913285113189,0.686717751601009));
#9375=CARTESIAN_POINT('Ctrl Pts',(-4.82649285791936,-3.75573162270607,0.69444261417343));
#9376=CARTESIAN_POINT('Ctrl Pts',(-4.72044858365999,-3.88817893987517,0.702167476745851));
#9377=CARTESIAN_POINT('Ctrl Pts',(-4.60907010354336,-4.01600527179967,0.709892339318273));
#9378=CARTESIAN_POINT('Ctrl Pts',(-4.49771333152076,-4.1438066898806,0.717615696285277));
#9379=CARTESIAN_POINT('Ctrl Pts',(-4.3810246361935,-4.26698868104521,0.72533905325228));
#9380=CARTESIAN_POINT('Ctrl Pts',(-4.25941156418452,-4.38511558449617,0.733062410219284));
#9381=CARTESIAN_POINT('Ctrl Pts',(-4.13779377703128,-4.50324706792674,0.740786066633885));
#9382=CARTESIAN_POINT('Ctrl Pts',(-4.01125145570191,-4.61632284780844,0.748509723048488));
#9383=CARTESIAN_POINT('Ctrl Pts',(-3.8802288134936,-4.72394431777451,0.756233379463089));
#9384=CARTESIAN_POINT('Ctrl Pts',(-3.74921496558499,-4.83155856413826,0.763956517462337));
#9385=CARTESIAN_POINT('Ctrl Pts',(-3.61372164350764,-4.93371903204126,0.771679655461583));
#9386=CARTESIAN_POINT('Ctrl Pts',(-3.47422605934365,-5.03006747977376,0.77940279346083));
#9387=CARTESIAN_POINT('Ctrl Pts',(-3.33469341163632,-5.12644152698949,0.78712798347385));
#9388=CARTESIAN_POINT('Ctrl Pts',(-3.19115663663698,-5.21700028625419,0.794853173486872));
#9389=CARTESIAN_POINT('Ctrl Pts',(-3.04412263002233,-5.30142839014976,0.802578363499892));
#9390=CARTESIAN_POINT('Ctrl Pts',(-2.8976704344348,-5.38552241349502,0.810272985069329));
#9391=CARTESIAN_POINT('Ctrl Pts',(-2.74774892083377,-5.46353408407591,0.817967606638764));
#9392=CARTESIAN_POINT('Ctrl Pts',(-2.59488388816268,-5.53519675977772,0.825662228208201));
#9393=CARTESIAN_POINT('Ctrl Pts',(-2.44142077045098,-5.60713981597963,0.833386955014744));
#9394=CARTESIAN_POINT('Ctrl Pts',(-2.28493669669956,-5.67270954479624,0.841111681821286));
#9395=CARTESIAN_POINT('Ctrl Pts',(-2.12597938050378,-5.73166967263229,0.848836408627829));
#9396=CARTESIAN_POINT('Ctrl Pts',(-1.96705308016936,-5.79061829612747,0.856559628180341));
#9397=CARTESIAN_POINT('Ctrl Pts',(-1.80565479728124,-5.84295978184344,0.864282847732854));
#9398=CARTESIAN_POINT('Ctrl Pts',(-1.64235082019659,-5.88850654630693,0.872006067285365));
#9399=CARTESIAN_POINT('Ctrl Pts',(-1.47904053792382,-5.93405506933701,0.879729585032403));
#9400=CARTESIAN_POINT('Ctrl Pts',(-1.31382471842629,-5.97280825718594,0.88745310277944));
#9401=CARTESIAN_POINT('Ctrl Pts',(-1.14728412070452,-6.00462860707299,0.895176620526479));
#9402=CARTESIAN_POINT('Ctrl Pts',(-0.980754710335357,-6.03644681943033,
0.902899619446772));
#9403=CARTESIAN_POINT('Ctrl Pts',(-0.812901011161869,-6.0613330663143,0.910622618367064));
#9404=CARTESIAN_POINT('Ctrl Pts',(-0.644313448120322,-6.07920107769691,
0.918345617287356));
#9405=CARTESIAN_POINT('Ctrl Pts',(-0.475681076905236,-6.09707383814251,
0.926070668870785));
#9406=CARTESIAN_POINT('Ctrl Pts',(-0.306314767223509,-6.1079246000756,0.933795720454216));
#9407=CARTESIAN_POINT('Ctrl Pts',(-0.13681049800793,-6.11171894397434,0.941520772037645));
#9408=CARTESIAN_POINT('Ctrl Pts',(0.032041197129254,-6.11549868003762,0.949216082963561));
#9409=CARTESIAN_POINT('Ctrl Pts',(0.201029478545488,-6.11227626028111,0.956911393889477));
#9410=CARTESIAN_POINT('Ctrl Pts',(0.369564889392573,-6.10206910441272,0.964606704815394));
#9411=CARTESIAN_POINT('Ctrl Pts',(0.538745432485311,-6.0918228768421,0.972331472418656));
#9412=CARTESIAN_POINT('Ctrl Pts',(0.707529554106069,-6.07453467526001,0.980056240021918));
#9413=CARTESIAN_POINT('Ctrl Pts',(0.875323246504274,-6.05025906690195,0.98778100762518));
#9414=CARTESIAN_POINT('Ctrl Pts',(1.04308420820422,-6.02598819386856,0.995504268395653));
#9415=CARTESIAN_POINT('Ctrl Pts',(1.2098548127118,-5.99473267908254,1.00322752916613));
#9416=CARTESIAN_POINT('Ctrl Pts',(1.37504803630819,-5.95659873252723,1.0109507899366));
#9417=CARTESIAN_POINT('Ctrl Pts',(1.54024764358799,-5.91846331233373,1.01867434916273));
#9418=CARTESIAN_POINT('Ctrl Pts',(1.7038694382931,-5.87344899589648,1.02639790838885));
#9419=CARTESIAN_POINT('Ctrl Pts',(1.86533764988907,-5.82171289350534,1.03412146761498));
#9420=CARTESIAN_POINT('Ctrl Pts',(2.02679501619993,-5.76998026605689,1.04184450807521));
#9421=CARTESIAN_POINT('Ctrl Pts',(2.18609878702905,-5.71152685285931,1.04956754853543));
#9422=CARTESIAN_POINT('Ctrl Pts',(2.34268921528692,-5.64655937745087,1.05729058899566));
#9423=CARTESIAN_POINT('Ctrl Pts',(2.49932125676971,-5.58157463721853,1.06501568182029));
#9424=CARTESIAN_POINT('Ctrl Pts',(2.65323822105741,-5.51007249517287,1.07274077464491));
#9425=CARTESIAN_POINT('Ctrl Pts',(2.80390029083196,-5.43230786329093,1.08046586746954));
#9426=CARTESIAN_POINT('Ctrl Pts',(2.95397750286972,-5.35484510730033,1.08816097212055));
#9427=CARTESIAN_POINT('Ctrl Pts',(3.10082478327173,-5.27116856773365,1.09585607677155));
#9428=CARTESIAN_POINT('Ctrl Pts',(3.24393289200808,-5.18157552821997,1.10355118142256));
#9429=CARTESIAN_POINT('Ctrl Pts',(3.38759122044311,-5.09163802286407,1.11127587208515));
#9430=CARTESIAN_POINT('Ctrl Pts',(3.52753242794613,-4.99570655549234,1.11900056274774));
#9431=CARTESIAN_POINT('Ctrl Pts',(3.66326102202065,-4.89411322376631,1.12672525341033));
#9432=CARTESIAN_POINT('Ctrl Pts',(3.68324059854396,-4.87915844021963,1.1278623465134));
#9433=CARTESIAN_POINT('Ctrl Pts',(3.70312894502161,-4.86408104885361,1.12899943961647));
#9434=CARTESIAN_POINT('Ctrl Pts',(3.72292453512039,-4.84888218750453,1.13013653271955));
#9435=CARTESIAN_POINT('Origin',(0.,0.,0.));
#9436=CARTESIAN_POINT('',(-4.29183622825304,2.82247096572396,18.4117650535551));
#9437=CARTESIAN_POINT('',(-4.29183622819587,2.82247096581089,18.8886809208774));
#9438=CARTESIAN_POINT('',(-4.29183622825304,2.82247096572397,0.));
#9439=CARTESIAN_POINT('',(4.95630975100502,1.34951628911715,20.));
#9440=CARTESIAN_POINT('Ctrl Pts',(4.95630975100503,1.34951628911712,20.));
#9441=CARTESIAN_POINT('Ctrl Pts',(5.02530589382568,1.09611715773841,19.985760168123));
#9442=CARTESIAN_POINT('Ctrl Pts',(5.07476845806476,0.83779585568772,19.9717441009936));
#9443=CARTESIAN_POINT('Ctrl Pts',(5.1218150352685,0.421484983818935,19.9491973439681));
#9444=CARTESIAN_POINT('Ctrl Pts',(5.13226903371038,0.265428195636579,19.940758950191));
#9445=CARTESIAN_POINT('Ctrl Pts',(5.14045498932613,-0.119762154763499,19.9198304701504));
#9446=CARTESIAN_POINT('Ctrl Pts',(5.1300101780035,-0.348729313788184,19.9072951957962));
#9447=CARTESIAN_POINT('Ctrl Pts',(5.0889160140276,-0.712747505217411,19.8871692238277));
#9448=CARTESIAN_POINT('Ctrl Pts',(5.06803371909913,-0.84859285855697,19.8796172623197));
#9449=CARTESIAN_POINT('Ctrl Pts',(5.02581032745821,-1.06505691087385,19.8675528749467));
#9450=CARTESIAN_POINT('Ctrl Pts',(5.00790987497494,-1.14627872475244,19.8630201081034));
#9451=CARTESIAN_POINT('Ctrl Pts',(4.94234733308433,-1.41279905148079,19.8481473500308));
#9452=CARTESIAN_POINT('Ctrl Pts',(4.88630680506449,-1.59587177542111,19.837910809985));
#9453=CARTESIAN_POINT('Ctrl Pts',(4.74025411427273,-1.99240401217042,19.8152538320208));
#9454=CARTESIAN_POINT('Ctrl Pts',(4.64576155677645,-2.20376481251868,19.8028440551837));
#9455=CARTESIAN_POINT('Ctrl Pts',(4.41903586086519,-2.63097371493999,19.7766204234566));
#9456=CARTESIAN_POINT('Ctrl Pts',(4.2844518484464,-2.84488454292749,19.7628135131264));
#9457=CARTESIAN_POINT('Ctrl Pts',(4.03429872523108,-3.18422073988682,19.7397008754151));
#9458=CARTESIAN_POINT('Ctrl Pts',(3.9272322427042,-3.3153697839732,19.7304310371072));
#9459=CARTESIAN_POINT('Ctrl Pts',(3.66663412093714,-3.60420810666249,19.7093400446914));
#9460=CARTESIAN_POINT('Ctrl Pts',(3.50905321579256,-3.75780135782271,19.6975958355295));
#9461=CARTESIAN_POINT('Ctrl Pts',(3.17877746362949,-4.04077194245563,19.6742682237264));
#9462=CARTESIAN_POINT('Ctrl Pts',(3.00681386490056,-4.17031553658563,19.6627090710648));
#9463=CARTESIAN_POINT('Ctrl Pts',(2.61835356823536,-4.42640047801557,19.6374696580365));
#9464=CARTESIAN_POINT('Ctrl Pts',(2.3996891680016,-4.54865736647821,19.6237791038255));
#9465=CARTESIAN_POINT('Ctrl Pts',(2.02558012934287,-4.72331379219015,19.60114309389));
#9466=CARTESIAN_POINT('Ctrl Pts',(1.87497726074543,-4.78509454034322,19.5922303821311));
#9467=CARTESIAN_POINT('Ctrl Pts',(1.54278421990625,-4.90327212686748,19.5731008180843));
#9468=CARTESIAN_POINT('Ctrl Pts',(1.36047834009044,-4.95695086501791,19.5629341636872));
#9469=CARTESIAN_POINT('Ctrl Pts',(0.961109557259161,-5.05084406473322,19.5409398437521));
#9470=CARTESIAN_POINT('Ctrl Pts',(0.743582581930314,-5.08741977359763,19.529126018642));
#9471=CARTESIAN_POINT('Ctrl Pts',(0.195183186632527,-5.14369690873679,19.4992824241404));
#9472=CARTESIAN_POINT('Ctrl Pts',(-0.136505696197581,-5.14558740425137,
19.4811420150829));
#9473=CARTESIAN_POINT('Ctrl Pts',(-0.592490824100446,-5.10404490011886,
19.4560588194645));
#9474=CARTESIAN_POINT('Ctrl Pts',(-0.718460756107112,-5.08784190893735,
19.4491224236343));
#9475=CARTESIAN_POINT('Ctrl Pts',(-1.02388383251126,-5.03698596369529,19.4323493632291));
#9476=CARTESIAN_POINT('Ctrl Pts',(-1.20233897843037,-4.99739421619772,19.4225706137207));
#9477=CARTESIAN_POINT('Ctrl Pts',(-1.58954298069361,-4.88954350859193,19.4010211332803));
#9478=CARTESIAN_POINT('Ctrl Pts',(-1.7967906699977,-4.81724231554643,19.3892618014552));
#9479=CARTESIAN_POINT('Ctrl Pts',(-2.28769513182071,-4.60988248520833,19.3604080865111));
#9480=CARTESIAN_POINT('Ctrl Pts',(-2.56482071175491,-4.46164219223895,19.3432292750671));
#9481=CARTESIAN_POINT('Ctrl Pts',(-2.9406328057709,-4.21396527559979,19.3185687856875));
#9482=CARTESIAN_POINT('Ctrl Pts',(-3.05154649102943,-4.13435487165146,19.3111085090113));
#9483=CARTESIAN_POINT('Ctrl Pts',(-3.30622214787486,-3.93571842684582,19.2936094306021));
#9484=CARTESIAN_POINT('Ctrl Pts',(-3.4469307845396,-3.8130899551909,19.2836268860308));
#9485=CARTESIAN_POINT('Ctrl Pts',(-3.73922808706123,-3.52892087326279,19.2617703579193));
#9486=CARTESIAN_POINT('Ctrl Pts',(-3.88767255959531,-3.36468553894342,19.2499080068004));
#9487=CARTESIAN_POINT('Ctrl Pts',(-4.21225799055328,-2.95531055366526,19.2216103869056));
#9488=CARTESIAN_POINT('Ctrl Pts',(-4.378309695436,-2.70321545620731,19.2051098800644));
#9489=CARTESIAN_POINT('Ctrl Pts',(-4.58932323689831,-2.31189330743614,19.1807408091588));
#9490=CARTESIAN_POINT('Ctrl Pts',(-4.65203482714063,-2.18295945966545,19.1729009130736));
#9491=CARTESIAN_POINT('Ctrl Pts',(-4.79073388762263,-1.86458288424742,19.1540783763617));
#9492=CARTESIAN_POINT('Ctrl Pts',(-4.86098627431131,-1.67290645695063,19.143172468624));
#9493=CARTESIAN_POINT('Ctrl Pts',(-4.98416476824743,-1.26277320776459,19.120210720972));
#9494=CARTESIAN_POINT('Ctrl Pts',(-5.03453675361378,-1.04399777864826,19.1081697792498));
#9495=CARTESIAN_POINT('Ctrl Pts',(-5.11087974117963,-0.573445011447198,
19.0823187470383));
#9496=CARTESIAN_POINT('Ctrl Pts',(-5.13288301479651,-0.321617695963115,
19.0685066801584));
#9497=CARTESIAN_POINT('Ctrl Pts',(-5.13852726620075,0.0973098189321237,
19.0455334154845));
#9498=CARTESIAN_POINT('Ctrl Pts',(-5.13267227472482,0.263834269357301,19.0364080184376));
#9499=CARTESIAN_POINT('Ctrl Pts',(-5.10298853574141,0.617370407419794,19.0171609458188));
#9500=CARTESIAN_POINT('Ctrl Pts',(-5.07693775185344,0.803955134054031,19.0070812083906));
#9501=CARTESIAN_POINT('Ctrl Pts',(-4.99743022062426,1.20931325277453,18.984934710332));
#9502=CARTESIAN_POINT('Ctrl Pts',(-4.93972011366581,1.42685321071505,18.9728814821261));
#9503=CARTESIAN_POINT('Ctrl Pts',(-4.76694952668741,1.93970962557575,18.9435787367963));
#9504=CARTESIAN_POINT('Ctrl Pts',(-4.63847493686506,2.22953403684096,18.9262471762037));
#9505=CARTESIAN_POINT('Ctrl Pts',(-4.42388634110982,2.61356094779722,18.902142851062));
#9506=CARTESIAN_POINT('Ctrl Pts',(-4.35973477672137,2.71922474860137,18.8953862161405));
#9507=CARTESIAN_POINT('Ctrl Pts',(-4.29183622819587,2.8224709658109,18.8886809208774));
#9508=CARTESIAN_POINT('',(-2.03116440553747,4.71811103304888,20.));
#9509=CARTESIAN_POINT('Origin',(0.,0.,20.));
#9510=CARTESIAN_POINT('Ctrl Pts',(-2.03116440553748,4.71811103304888,20.));
#9511=CARTESIAN_POINT('Ctrl Pts',(-1.75876294038136,4.83538088027497,19.9838242100236));
#9512=CARTESIAN_POINT('Ctrl Pts',(-1.47671310578932,4.92884170022616,19.9675020813374));
#9513=CARTESIAN_POINT('Ctrl Pts',(-1.02673667725821,5.03582637935673,19.9422943163514));
#9514=CARTESIAN_POINT('Ctrl Pts',(-0.863532856038434,5.06636440626909,19.9333064352754));
#9515=CARTESIAN_POINT('Ctrl Pts',(-0.431451545577099,5.12572502375573,19.9097964073362));
#9516=CARTESIAN_POINT('Ctrl Pts',(-0.161285469164626,5.14132214210612,19.8953967529817));
#9517=CARTESIAN_POINT('Ctrl Pts',(0.211096044340629,5.13342946063892,19.8753425674653));
#9518=CARTESIAN_POINT('Ctrl Pts',(0.313252013380761,5.12820946562538,19.8698131775709));
#9519=CARTESIAN_POINT('Ctrl Pts',(0.664459217167201,5.09972949640327,19.8506286802133));
#9520=CARTESIAN_POINT('Ctrl Pts',(0.9119239339857,5.06133791149605,19.8368700328516));
#9521=CARTESIAN_POINT('Ctrl Pts',(1.30420074646597,4.9707664040537,19.814850744872));
#9522=CARTESIAN_POINT('Ctrl Pts',(1.45119646922876,4.92985683047897,19.8065459912916));
#9523=CARTESIAN_POINT('Ctrl Pts',(1.83322012950886,4.80496724601604,19.7847711270967));
#9524=CARTESIAN_POINT('Ctrl Pts',(2.06432719374341,4.71030387023003,19.7714126359105));
#9525=CARTESIAN_POINT('Ctrl Pts',(2.44210240830701,4.52239937182995,19.7487917799261));
#9526=CARTESIAN_POINT('Ctrl Pts',(2.5925895512669,4.43784154113219,19.7395456576355));
#9527=CARTESIAN_POINT('Ctrl Pts',(2.84885340339452,4.27635801571134,19.7231141398198));
#9528=CARTESIAN_POINT('Ctrl Pts',(2.95648431131262,4.20266619585462,19.7159828904466));
#9529=CARTESIAN_POINT('Ctrl Pts',(3.24673701093696,3.98726546220093,19.6961752000313));
#9530=CARTESIAN_POINT('Ctrl Pts',(3.42278213919766,3.83720630644497,19.6835004441861));
#9531=CARTESIAN_POINT('Ctrl Pts',(3.70898082723071,3.55783425299693,19.6617256398255));
#9532=CARTESIAN_POINT('Ctrl Pts',(3.82394472492539,3.43397319677323,19.6525909097226));
#9533=CARTESIAN_POINT('Ctrl Pts',(4.13971273079861,3.05820548543407,19.6261636191148));
#9534=CARTESIAN_POINT('Ctrl Pts',(4.32319237180496,2.79281963364292,19.609072260082));
#9535=CARTESIAN_POINT('Ctrl Pts',(4.57204856975284,2.34894135533897,19.5814745437388));
#9536=CARTESIAN_POINT('Ctrl Pts',(4.65450356788183,2.18099704756942,19.571220452595));
#9537=CARTESIAN_POINT('Ctrl Pts',(4.81576975519437,1.80149005543778,19.5486093361489));
#9538=CARTESIAN_POINT('Ctrl Pts',(4.89017290886852,1.58846379613654,19.536282487004));
#9539=CARTESIAN_POINT('Ctrl Pts',(5.03514514724615,1.06509540907264,19.5068128983632));
#9540=CARTESIAN_POINT('Ctrl Pts',(5.09136502481458,0.751745249377349,19.489851744901));
#9541=CARTESIAN_POINT('Ctrl Pts',(5.12964176007384,0.30159365592701,19.4656042644915));
#9542=CARTESIAN_POINT('Ctrl Pts',(5.13576651018031,0.167585179481134,19.4583926493008));
#9543=CARTESIAN_POINT('Ctrl Pts',(5.13786573095127,-0.154375327316645,19.4409097676649));
#9544=CARTESIAN_POINT('Ctrl Pts',(5.12878318906439,-0.342165695784814,19.4306008150461));
#9545=CARTESIAN_POINT('Ctrl Pts',(5.08672347758837,-0.74838099282315,19.4082085618613));
#9546=CARTESIAN_POINT('Ctrl Pts',(5.04991038522345,-0.966042645175719,19.3961551733762));
#9547=CARTESIAN_POINT('Ctrl Pts',(4.93085103721109,-1.4701681469757,19.3680573869256));
#9548=CARTESIAN_POINT('Ctrl Pts',(4.83746124673004,-1.75318535202099,19.352157458766));
#9549=CARTESIAN_POINT('Ctrl Pts',(4.66261804777703,-2.16042253749514,19.3283824011532));
#9550=CARTESIAN_POINT('Ctrl Pts',(4.59946231667175,-2.29180666574483,19.3205550036784));
#9551=CARTESIAN_POINT('Ctrl Pts',(4.43450863255362,-2.60059698282352,19.3015524206627));
#9552=CARTESIAN_POINT('Ctrl Pts',(4.32753760437117,-2.77495727721709,19.2903305536088));
#9553=CARTESIAN_POINT('Ctrl Pts',(4.08216582852423,-3.12606590849171,19.2668479553779));
#9554=CARTESIAN_POINT('Ctrl Pts',(3.94199337408599,-3.30106921498769,19.2546185202404));
#9555=CARTESIAN_POINT('Ctrl Pts',(3.62194279043492,-3.65107894683408,19.2289222747411));
#9556=CARTESIAN_POINT('Ctrl Pts',(3.43976506524457,-3.82320106591323,19.2155164664277));
#9557=CARTESIAN_POINT('Ctrl Pts',(3.11278065081963,-4.08977208511344,19.1928968803583));
#9558=CARTESIAN_POINT('Ctrl Pts',(2.97445016187949,-4.19145359471505,19.1836997073477));
#9559=CARTESIAN_POINT('Ctrl Pts',(2.68287896765122,-4.38406208132611,19.1647424728127));
#9560=CARTESIAN_POINT('Ctrl Pts',(2.52947310941184,-4.47432720799941,19.1549898266571));
#9561=CARTESIAN_POINT('Ctrl Pts',(2.16558623509264,-4.66373545881771,19.1324944427109));
#9562=CARTESIAN_POINT('Ctrl Pts',(1.95242925752933,-4.75691244497512,19.1197834178669));
#9563=CARTESIAN_POINT('Ctrl Pts',(1.43531652543014,-4.94232151271111,19.0899739422836));
#9564=CARTESIAN_POINT('Ctrl Pts',(1.12767482714869,-5.02145684046532,19.0730491469159));
#9565=CARTESIAN_POINT('Ctrl Pts',(0.681967033058751,-5.0930536087937,19.0488210854185));
#9566=CARTESIAN_POINT('Ctrl Pts',(0.54844774318353,-5.10915631787797,19.0415915442061));
#9567=CARTESIAN_POINT('Ctrl Pts',(0.226770606839126,-5.13519528115496,19.0240675179371));
#9568=CARTESIAN_POINT('Ctrl Pts',(0.0383985421090806,-5.14005635979088,
19.0137351640574));
#9569=CARTESIAN_POINT('Ctrl Pts',(-0.370040583681346,-5.12813928827051,
18.9913306270689));
#9570=CARTESIAN_POINT('Ctrl Pts',(-0.589631825340411,-5.10755130569912,
18.9792882671527));
#9571=CARTESIAN_POINT('Ctrl Pts',(-1.10031682802839,-5.02628904669437,18.9512386610511));
#9572=CARTESIAN_POINT('Ctrl Pts',(-1.38881776421128,-4.95433827868492,18.9353747119186));
#9573=CARTESIAN_POINT('Ctrl Pts',(-1.80772373185749,-4.8103742465423,18.9116122951975));
#9574=CARTESIAN_POINT('Ctrl Pts',(-1.94386254984276,-4.75699092412569,18.9037607272593));
#9575=CARTESIAN_POINT('Ctrl Pts',(-2.26490235117464,-4.61501774531452,18.884707078263));
#9576=CARTESIAN_POINT('Ctrl Pts',(-2.44713993640201,-4.52102595707778,18.8734581563373));
#9577=CARTESIAN_POINT('Ctrl Pts',(-2.81553184456781,-4.30220698923688,18.8499686921729));
#9578=CARTESIAN_POINT('Ctrl Pts',(-3.00013058062337,-4.17557479132149,18.8377591677673));
#9579=CARTESIAN_POINT('Ctrl Pts',(-3.36346396170165,-3.88976417072007,18.8127133070388));
#9580=CARTESIAN_POINT('Ctrl Pts',(-3.54052077378501,-3.72932472488589,18.7999225102669));
#9581=CARTESIAN_POINT('Ctrl Pts',(-3.83275328361216,-3.4248820219363,18.7772977795739));
#9582=CARTESIAN_POINT('Ctrl Pts',(-3.95255484781583,-3.28589867451037,18.7674765495375));
#9583=CARTESIAN_POINT('Ctrl Pts',(-4.1730526470859,-3.00054246384596,18.7479125947867));
#9584=CARTESIAN_POINT('Ctrl Pts',(-4.27410457203303,-2.8547595135527,18.7381935793223));
#9585=CARTESIAN_POINT('Ctrl Pts',(-4.42859745019339,-2.60523182163145,18.7221001709323));
#9586=CARTESIAN_POINT('Ctrl Pts',(-4.48640740096312,-2.50436761210014,18.7157299162025));
#9587=CARTESIAN_POINT('Ctrl Pts',(-4.57860830881648,-2.33004387857943,18.7049509495119));
#9588=CARTESIAN_POINT('Ctrl Pts',(-4.61477230822775,-2.25757286804229,18.7005344319853));
#9589=CARTESIAN_POINT('Ctrl Pts',(-4.72247152053522,-2.02833632249747,18.6867574872509));
#9590=CARTESIAN_POINT('Ctrl Pts',(-4.78784393728745,-1.86880652217347,18.6774498202014));
#9591=CARTESIAN_POINT('Ctrl Pts',(-4.94616864022449,-1.41923769466512,18.6518102469528));
#9592=CARTESIAN_POINT('Ctrl Pts',(-5.02154789416998,-1.12377448705335,18.6356373139083));
#9593=CARTESIAN_POINT('Ctrl Pts',(-5.10090104584609,-0.635126718511599,
18.6087926659858));
#9594=CARTESIAN_POINT('Ctrl Pts',(-5.12096401959124,-0.445311952233824,
18.5983302540382));
#9595=CARTESIAN_POINT('Ctrl Pts',(-5.14137951378069,-0.034284679017604,
18.5757641295428));
#9596=CARTESIAN_POINT('Ctrl Pts',(-5.13810193422646,0.18673673320556,18.563688843334));
#9597=CARTESIAN_POINT('Ctrl Pts',(-5.0950259670139,0.728873128613459,18.5341740124312));
#9598=CARTESIAN_POINT('Ctrl Pts',(-5.03912318960092,1.04775328274904,18.5169319461479));
#9599=CARTESIAN_POINT('Ctrl Pts',(-4.91889111265508,1.48592026110536,18.4925420780072));
#9600=CARTESIAN_POINT('Ctrl Pts',(-4.87929476383411,1.61118918792427,18.4854771887509));
#9601=CARTESIAN_POINT('Ctrl Pts',(-4.77302687055334,1.9073607047389,18.4683891135196));
#9602=CARTESIAN_POINT('Ctrl Pts',(-4.70191931669328,2.07647863647284,18.4583310561176));
#9603=CARTESIAN_POINT('Ctrl Pts',(-4.5246343402553,2.4420477874444,18.4360531501995));
#9604=CARTESIAN_POINT('Ctrl Pts',(-4.41438337869704,2.63612143528974,18.4238641311583));
#9605=CARTESIAN_POINT('Ctrl Pts',(-4.29185896137503,2.82243639764222,18.4117672979533));
#9606=CARTESIAN_POINT('Ctrl Pts',(-4.2918475948598,2.82245368171457,18.4117661757578));
#9607=CARTESIAN_POINT('Ctrl Pts',(-4.29183622825304,2.82247096572396,18.4117650535551));
#9608=CARTESIAN_POINT('Origin',(0.,0.,0.));
#9609=CARTESIAN_POINT('',(-4.2921400227931,2.82267100337914,16.6620149077712));
#9610=CARTESIAN_POINT('',(-4.29183622825303,2.82247096572397,17.1389378634518));
#9611=CARTESIAN_POINT('',(-4.29183622825304,2.82247096572397,0.));
#9612=CARTESIAN_POINT('',(-5.1367499996765,-5.76498924387363E-5,17.3009584946969));
#9613=CARTESIAN_POINT('Ctrl Pts',(-4.29183622825303,2.82247096572397,17.1389378634518));
#9614=CARTESIAN_POINT('Ctrl Pts',(-4.37359531714591,2.69814847526767,17.1470045559175));
#9615=CARTESIAN_POINT('Ctrl Pts',(-4.44995155153085,2.57026701404298,17.1550712483833));
#9616=CARTESIAN_POINT('Ctrl Pts',(-4.52061197112331,2.43931711120892,17.1631379408491));
#9617=CARTESIAN_POINT('Ctrl Pts',(-4.59127033350124,2.30837102086345,17.1712043984604));
#9618=CARTESIAN_POINT('Ctrl Pts',(-4.65623305756608,2.1743569599479,17.1792708560717));
#9619=CARTESIAN_POINT('Ctrl Pts',(-4.71525317845947,2.03778998562851,17.187337313683));
#9620=CARTESIAN_POINT('Ctrl Pts',(-4.77428652497719,1.90119240846606,17.1954055788802));
#9621=CARTESIAN_POINT('Ctrl Pts',(-4.82737447737193,1.76204107923804,17.2034738440774));
#9622=CARTESIAN_POINT('Ctrl Pts',(-4.87431801938217,1.62087149658026,17.2115421092746));
#9623=CARTESIAN_POINT('Ctrl Pts',(-4.892875195019,1.56506597727393,17.2147315621351));
#9624=CARTESIAN_POINT('Ctrl Pts',(-4.91047273029335,1.50894526372987,17.2179210149957));
#9625=CARTESIAN_POINT('Ctrl Pts',(-4.92710046533172,1.45254313775113,17.2211104678562));
#9626=CARTESIAN_POINT('Ctrl Pts',(-4.96940617618376,1.30904000713293,17.2292253476149));
#9627=CARTESIAN_POINT('Ctrl Pts',(-5.00544537854101,1.16366362598839,17.2373402273735));
#9628=CARTESIAN_POINT('Ctrl Pts',(-5.03507358990828,1.0169732084515,17.2454551071321));
#9629=CARTESIAN_POINT('Ctrl Pts',(-5.06469490923402,0.870316913678134,17.2535680992274));
#9630=CARTESIAN_POINT('Ctrl Pts',(-5.08790814974416,0.722347508930372,17.2616810913227));
#9631=CARTESIAN_POINT('Ctrl Pts',(-5.10461981860422,0.573634962334952,17.269794083418));
#9632=CARTESIAN_POINT('Ctrl Pts',(-5.12132933420445,0.424941577006755,17.277906030173));
#9633=CARTESIAN_POINT('Ctrl Pts',(-5.13153891306429,0.275505561659813,17.286017976928));
#9634=CARTESIAN_POINT('Ctrl Pts',(-5.13520681056804,0.125903038865496,17.2941299236831));
#9635=CARTESIAN_POINT('Ctrl Pts',(-5.13623601269556,0.083924975251689,17.296406114021));
#9636=CARTESIAN_POINT('Ctrl Pts',(-5.13675047094801,0.0419338240484392,
17.298682304359));
#9637=CARTESIAN_POINT('Ctrl Pts',(-5.1367499996765,-5.76498924387363E-5,
17.3009584946969));
#9638=CARTESIAN_POINT('Ctrl Pts',(-4.29183622819587,2.82247096581089,18.8886809208774));
#9639=CARTESIAN_POINT('Ctrl Pts',(-4.28567102649408,2.83184574285497,18.8880720787348));
#9640=CARTESIAN_POINT('Ctrl Pts',(-4.27947493157269,2.84120058855997,18.8874636785894));
#9641=CARTESIAN_POINT('Ctrl Pts',(-4.16840366187836,3.00770793814683,18.8766188854153));
#9642=CARTESIAN_POINT('Ctrl Pts',(-4.0549659063518,3.15897928524874,18.8665078330849));
#9643=CARTESIAN_POINT('Ctrl Pts',(-3.78354837421278,3.48213842336234,18.843881669676));
#9644=CARTESIAN_POINT('Ctrl Pts',(-3.62167446121573,3.65020511107423,18.8313769842141));
#9645=CARTESIAN_POINT('Ctrl Pts',(-3.24892560801987,3.98792386684946,18.8041072757814));
#9646=CARTESIAN_POINT('Ctrl Pts',(-3.03493035403199,4.15310079458692,18.7893320173679));
#9647=CARTESIAN_POINT('Ctrl Pts',(-2.67675336823147,4.38704061934109,18.7658765148313));
#9648=CARTESIAN_POINT('Ctrl Pts',(-2.54063689495991,4.46724746478873,18.757230077586));
#9649=CARTESIAN_POINT('Ctrl Pts',(-2.1976262844609,4.64861099894477,18.7361942724354));
#9650=CARTESIAN_POINT('Ctrl Pts',(-1.9872115651427,4.7423770187691,18.7239105215631));
#9651=CARTESIAN_POINT('Ctrl Pts',(-1.57763255577205,4.8928322999547,18.7005036795224));
#9652=CARTESIAN_POINT('Ctrl Pts',(-1.37994470544255,4.95221995041138,18.6894146110521));
#9653=CARTESIAN_POINT('Ctrl Pts',(-1.01465516975105,5.03837928221641,18.6690532135946));
#9654=CARTESIAN_POINT('Ctrl Pts',(-0.848270549384174,5.06904589571288,18.6598277199854));
#9655=CARTESIAN_POINT('Ctrl Pts',(-0.43721538511567,5.12400015846466,18.6371130870805));
#9656=CARTESIAN_POINT('Ctrl Pts',(-0.191728009324919,5.1390444046113,18.6236045150092));
#9657=CARTESIAN_POINT('Ctrl Pts',(0.22726986279079,5.13464815936065,18.6008770042723));
#9658=CARTESIAN_POINT('Ctrl Pts',(0.400446477283491,5.12405192758401,18.5915844507442));
#9659=CARTESIAN_POINT('Ctrl Pts',(0.818354410610287,5.0771619706189,18.5690376532882));
#9660=CARTESIAN_POINT('Ctrl Pts',(1.06163820392017,5.03191801728217,18.5557985573287));
#9661=CARTESIAN_POINT('Ctrl Pts',(1.51725978741158,4.91265989925699,18.5302814731074));
#9662=CARTESIAN_POINT('Ctrl Pts',(1.72986335144501,4.84188739353601,18.5180600379684));
#9663=CARTESIAN_POINT('Ctrl Pts',(2.12661365437589,4.68033709088422,18.4945758632146));
#9664=CARTESIAN_POINT('Ctrl Pts',(2.31128519370989,4.59194986319994,18.4833443115668));
#9665=CARTESIAN_POINT('Ctrl Pts',(2.61774314215245,4.42209087481972,18.4643256788713));
#9666=CARTESIAN_POINT('Ctrl Pts',(2.74222388080037,4.34599542791154,18.4564918082633));
#9667=CARTESIAN_POINT('Ctrl Pts',(3.11014098228951,4.0989778829039,18.4327186936835));
#9668=CARTESIAN_POINT('Ctrl Pts',(3.3421236306895,3.91213527254424,18.4168269690776));
#9669=CARTESIAN_POINT('Ctrl Pts',(3.71579414655474,3.55355194399674,18.3887347512914));
#9670=CARTESIAN_POINT('Ctrl Pts',(3.86494412048878,3.39073164066515,18.3766783567414));
#9671=CARTESIAN_POINT('Ctrl Pts',(4.12085248980146,3.07246633493118,18.3542860162302));
#9672=CARTESIAN_POINT('Ctrl Pts',(4.2304274473692,2.91975339389395,18.3439800040664));
#9673=CARTESIAN_POINT('Ctrl Pts',(4.40353646433848,2.64822148498378,18.3264943475812));
#9674=CARTESIAN_POINT('Ctrl Pts',(4.47121732212872,2.53227703200014,18.3192771841691));
#9675=CARTESIAN_POINT('Ctrl Pts',(4.6834470684315,2.13360932565539,18.2950371532842));
#9676=CARTESIAN_POINT('Ctrl Pts',(4.8063163666821,1.84018594964896,18.278088669385));
#9677=CARTESIAN_POINT('Ctrl Pts',(4.96722982386203,1.32715383088493,18.2489121923307));
#9678=CARTESIAN_POINT('Ctrl Pts',(5.01955921314604,1.11298309318419,18.2368698918193));
#9679=CARTESIAN_POINT('Ctrl Pts',(5.08960228793428,0.71763845862642,18.2148542208892));
#9680=CARTESIAN_POINT('Ctrl Pts',(5.11175491925199,0.537605427652224,18.2049101328354));
#9681=CARTESIAN_POINT('Ctrl Pts',(5.13337913338866,0.227019551725915,18.1880014756885));
#9682=CARTESIAN_POINT('Ctrl Pts',(5.13748164677116,0.0969655137992032,18.181003285117));
#9683=CARTESIAN_POINT('Ctrl Pts',(5.13454497795426,-0.358674369149742,18.1565426970965));
#9684=CARTESIAN_POINT('Ctrl Pts',(5.10149933775087,-0.683300915123357,18.1391672353028));
#9685=CARTESIAN_POINT('Ctrl Pts',(4.99443205170792,-1.22129784171954,18.1093955110344));
#9686=CARTESIAN_POINT('Ctrl Pts',(4.93671781388726,-1.43691814050995,18.0972005153241));
#9687=CARTESIAN_POINT('Ctrl Pts',(4.80525064743935,-1.82500803399851,18.0747317140419));
#9688=CARTESIAN_POINT('Ctrl Pts',(4.73571723963228,-1.99851753693678,18.0644869468147));
#9689=CARTESIAN_POINT('Ctrl Pts',(4.58361934618337,-2.32524720069935,18.0449414942034));
#9690=CARTESIAN_POINT('Ctrl Pts',(4.50241766359103,-2.47882598243922,18.0356375836716));
#9691=CARTESIAN_POINT('Ctrl Pts',(4.28772277484999,-2.83939527562957,18.0131382829671));
#9692=CARTESIAN_POINT('Ctrl Pts',(4.14682833088724,-3.04147068432655,17.9999575263177));
#9693=CARTESIAN_POINT('Ctrl Pts',(3.85106930918717,-3.40670141279893,17.9744949527394));
#9694=CARTESIAN_POINT('Ctrl Pts',(3.69891246869681,-3.57132917596064,17.9622680148383));
#9695=CARTESIAN_POINT('Ctrl Pts',(3.38824820635048,-3.86623337151898,17.938785663064));
#9696=CARTESIAN_POINT('Ctrl Pts',(3.23172262745006,-3.99799413733433,17.92756151357));
#9697=CARTESIAN_POINT('Ctrl Pts',(2.95081342955522,-4.20715581820003,17.9085513872989));
#9698=CARTESIAN_POINT('Ctrl Pts',(2.83020990250404,-4.28921590616174,17.9007187680953));
#9699=CARTESIAN_POINT('Ctrl Pts',(2.4535433097544,-4.5226918201582,17.8769451451976));
#9700=CARTESIAN_POINT('Ctrl Pts',(2.18768863766049,-4.65710539250038,17.8610517034469));
#9701=CARTESIAN_POINT('Ctrl Pts',(1.70697725034928,-4.84985380145168,17.8329582245202));
#9702=CARTESIAN_POINT('Ctrl Pts',(1.49717687702778,-4.91866965582099,17.8209023604202));
#9703=CARTESIAN_POINT('Ctrl Pts',(1.10173955059713,-5.02072204643755,17.798509766197));
#9704=CARTESIAN_POINT('Ctrl Pts',(0.917430856515096,-5.05764788961084,17.7882029656857));
#9705=CARTESIAN_POINT('Ctrl Pts',(0.598698321023235,-5.10350523942269,17.7707175490202));
#9706=CARTESIAN_POINT('Ctrl Pts',(0.465185571669131,-5.11740253197068,17.7635013785421));
#9707=CARTESIAN_POINT('Ctrl Pts',(0.0144697610531822,-5.14653075311769,
17.7392603899139));
#9708=CARTESIAN_POINT('Ctrl Pts',(-0.303551289442379,-5.1375909656368,17.7223100080063));
#9709=CARTESIAN_POINT('Ctrl Pts',(-0.849440783413805,-5.07135818226045,
17.692470557552));
#9710=CARTESIAN_POINT('Ctrl Pts',(-1.07800685676574,-5.02773515923622,17.6797561353485));
#9711=CARTESIAN_POINT('Ctrl Pts',(-1.47458459914182,-4.9237515809517,17.657274299014));
#9712=CARTESIAN_POINT('Ctrl Pts',(-1.64389383976998,-4.86984025617014,17.6475385489272));
#9713=CARTESIAN_POINT('Ctrl Pts',(-1.97210636722166,-4.7462589722096,17.6285126079779));
#9714=CARTESIAN_POINT('Ctrl Pts',(-2.13095486650566,-4.67709431563192,17.6192323217107));
#9715=CARTESIAN_POINT('Ctrl Pts',(-2.50885491894068,-4.48929526969065,17.5966068682422));
#9716=CARTESIAN_POINT('Ctrl Pts',(-2.72335511615857,-4.36250603516885,17.5832776712024));
#9717=CARTESIAN_POINT('Ctrl Pts',(-3.11179307903059,-4.09305246121396,17.5576643949609));
#9718=CARTESIAN_POINT('Ctrl Pts',(-3.2872237599939,-3.95354154702929,17.5454392737154));
#9719=CARTESIAN_POINT('Ctrl Pts',(-3.60436348847681,-3.66559260309525,17.5219562055037));
#9720=CARTESIAN_POINT('Ctrl Pts',(-3.74739920314977,-3.51923377650921,17.5107294974293));
#9721=CARTESIAN_POINT('Ctrl Pts',(-3.93500875435967,-3.30282027969124,17.4951831740091));
#9722=CARTESIAN_POINT('Ctrl Pts',(-3.98719681820654,-3.23962613228291,17.4907607822306));
#9723=CARTESIAN_POINT('Ctrl Pts',(-4.13608238250839,-3.05029129528728,17.4777986243122));
#9724=CARTESIAN_POINT('Ctrl Pts',(-4.22846405416202,-2.92088116657053,17.4692975507402));
#9725=CARTESIAN_POINT('Ctrl Pts',(-4.42032734598644,-2.62388997790252,17.4503296429262));
#9726=CARTESIAN_POINT('Ctrl Pts',(-4.51657509823625,-2.45451414535387,17.439863364329));
#9727=CARTESIAN_POINT('Ctrl Pts',(-4.67047743021137,-2.1438204908354,17.4210657071102));
#9728=CARTESIAN_POINT('Ctrl Pts',(-4.73189225998554,-2.00462467103621,17.4127791494057));
#9729=CARTESIAN_POINT('Ctrl Pts',(-4.84196947364945,-1.72176421404937,17.3961713318408));
#9730=CARTESIAN_POINT('Ctrl Pts',(-4.89062846405803,-1.57825642847592,17.3878584696979));
#9731=CARTESIAN_POINT('Ctrl Pts',(-4.96275726543717,-1.32993147718,17.3736924384381));
#9732=CARTESIAN_POINT('Ctrl Pts',(-4.98941405036863,-1.22614247813126,17.3678355417351));
#9733=CARTESIAN_POINT('Ctrl Pts',(-5.03187807510936,-1.03635566764883,17.3572685016428));
#9734=CARTESIAN_POINT('Ctrl Pts',(-5.04877269601564,-0.950644272263282,
17.3525519515872));
#9735=CARTESIAN_POINT('Ctrl Pts',(-5.11223467734277,-0.578958407071054,
17.3322558616643));
#9736=CARTESIAN_POINT('Ctrl Pts',(-5.13674744982588,-0.289762218613553,
17.3168255570649));
#9737=CARTESIAN_POINT('Ctrl Pts',(-5.13674999980103,-4.52116533001395E-5,
17.3011889615917));
#9738=CARTESIAN_POINT('',(-5.13710816050031,7.20752253655782E-5,16.8240415053031));
#9739=CARTESIAN_POINT('Ctrl Pts',(-4.29183622825304,2.82247096572396,18.4117650535551));
#9740=CARTESIAN_POINT('Ctrl Pts',(-4.17729142014888,2.99664726838564,18.4004562709275));
#9741=CARTESIAN_POINT('Ctrl Pts',(-4.0522485494874,3.16369132246763,18.3892490601967));
#9742=CARTESIAN_POINT('Ctrl Pts',(-3.76714717503251,3.49982275379707,18.3656070223839));
#9743=CARTESIAN_POINT('Ctrl Pts',(-3.60505464161424,3.66656979677188,18.3532065310692));
#9744=CARTESIAN_POINT('Ctrl Pts',(-3.40233792251312,3.84862474822056,18.3384239057725));
#9745=CARTESIAN_POINT('Ctrl Pts',(-3.3721224706653,3.87512655160327,18.3362377016896));
#9746=CARTESIAN_POINT('Ctrl Pts',(-3.16459498699542,4.05288239833501,18.3213445081467));
#9747=CARTESIAN_POINT('Ctrl Pts',(-2.97747823462929,4.19227149667809,18.308528637086));
#9748=CARTESIAN_POINT('Ctrl Pts',(-2.6276227720543,4.41761479696217,18.285761427677));
#9749=CARTESIAN_POINT('Ctrl Pts',(-2.46850719240987,4.50845832669544,18.2757979316256));
#9750=CARTESIAN_POINT('Ctrl Pts',(-2.23495718032712,4.62572032282574,18.2616626597772));
#9751=CARTESIAN_POINT('Ctrl Pts',(-2.1642419495692,4.65922515641597,18.2574426905591));
#9752=CARTESIAN_POINT('Ctrl Pts',(-1.91113091214703,4.7721427390743,18.2425244393054));
#9753=CARTESIAN_POINT('Ctrl Pts',(-1.72491935742319,4.84256349010087,18.2318918003444));
#9754=CARTESIAN_POINT('Ctrl Pts',(-1.42338688275734,4.93699023108016,18.2149285670648));
#9755=CARTESIAN_POINT('Ctrl Pts',(-1.31051830412915,4.96814288313003,18.2086315397027));
#9756=CARTESIAN_POINT('Ctrl Pts',(-1.02879923236747,5.03563067068677,18.1929225210189));
#9757=CARTESIAN_POINT('Ctrl Pts',(-0.858994116135272,5.06735940509753,18.1834611450474));
#9758=CARTESIAN_POINT('Ctrl Pts',(-0.440305647335727,5.12394016925705,18.1602935892258));
#9759=CARTESIAN_POINT('Ctrl Pts',(-0.190577052903982,5.13929149893427,18.1466237460747));
#9760=CARTESIAN_POINT('Ctrl Pts',(0.283097573035408,5.13382488326603,18.1209350438989));
#9761=CARTESIAN_POINT('Ctrl Pts',(0.506510921764593,5.11661526517205,18.1089163947818));
#9762=CARTESIAN_POINT('Ctrl Pts',(0.930586198121767,5.05589307083235,18.0859453006201));
#9763=CARTESIAN_POINT('Ctrl Pts',(1.13116455350242,5.01482891895945,18.075008035215));
#9764=CARTESIAN_POINT('Ctrl Pts',(1.46969291534403,4.92417416753471,18.0560127457752));
#9765=CARTESIAN_POINT('Ctrl Pts',(1.60895616593196,4.88044536116322,18.0480301927375));
#9766=CARTESIAN_POINT('Ctrl Pts',(2.02565778031868,4.7298237745217,18.0237429862404));
#9767=CARTESIAN_POINT('Ctrl Pts',(2.29586269470293,4.60473069894816,18.0074693807844));
#9768=CARTESIAN_POINT('Ctrl Pts',(2.74505358913806,4.34735559338287,17.9794278079863));
#9769=CARTESIAN_POINT('Ctrl Pts',(2.9291168759043,4.22552916188098,17.9675994920698));
#9770=CARTESIAN_POINT('Ctrl Pts',(3.25452720053356,3.97864093698851,17.9456998901642));
#9771=CARTESIAN_POINT('Ctrl Pts',(3.39791956332195,3.85689916695081,17.9356404723725));
#9772=CARTESIAN_POINT('Ctrl Pts',(3.63175183942997,3.63519027744683,17.9181817162467));
#9773=CARTESIAN_POINT('Ctrl Pts',(3.72552755113281,3.53902143615341,17.9108423986012));
#9774=CARTESIAN_POINT('Ctrl Pts',(4.02786888909865,3.20361490148474,17.8861005576203));
#9775=CARTESIAN_POINT('Ctrl Pts',(4.21802522448991,2.94875379992072,17.8687163620516));
#9776=CARTESIAN_POINT('Ctrl Pts',(4.49743004609412,2.49140974007656,17.8396978938611));
#9777=CARTESIAN_POINT('Ctrl Pts',(4.59938362969397,2.29775370792452,17.8279726521861));
#9778=CARTESIAN_POINT('Ctrl Pts',(4.76359026749968,1.9308117096969,17.8064197243696));
#9779=CARTESIAN_POINT('Ctrl Pts',(4.82947421410003,1.7595461372621,17.7966035667384));
#9780=CARTESIAN_POINT('Ctrl Pts',(4.92659405520577,1.46018039391778,17.7795535273557));
#9781=CARTESIAN_POINT('Ctrl Pts',(4.96232099674567,1.33372583620419,17.772375401574));
#9782=CARTESIAN_POINT('Ctrl Pts',(5.06898965010618,0.892105387063896,17.7474856355408));
#9783=CARTESIAN_POINT('Ctrl Pts',(5.11504369155602,0.571704615707682,17.7297880473185));
#9784=CARTESIAN_POINT('Ctrl Pts',(5.14141410628452,0.0285588752323948,17.7003483308169));
#9785=CARTESIAN_POINT('Ctrl Pts',(5.13789071047248,-0.192447469864089,17.6885093298539));
#9786=CARTESIAN_POINT('Ctrl Pts',(5.10483646691397,-0.602690807280177,17.6664437945442));
#9787=CARTESIAN_POINT('Ctrl Pts',(5.07893563493334,-0.791834426917885,17.6562312185668));
#9788=CARTESIAN_POINT('Ctrl Pts',(4.98456698068468,-1.27785603291861,17.6293697419292));
#9789=CARTESIAN_POINT('Ctrl Pts',(4.90012152203756,-1.57087018022075,17.6125991913699));
#9790=CARTESIAN_POINT('Ctrl Pts',(4.72802933968859,-2.01534667133899,17.5865624835649));
#9791=CARTESIAN_POINT('Ctrl Pts',(4.65777824027157,-2.17278335127782,17.5772047004971));
#9792=CARTESIAN_POINT('Ctrl Pts',(4.54307083848007,-2.39859673866215,17.5635237235733));
#9793=CARTESIAN_POINT('Ctrl Pts',(4.50469127772786,-2.46992219036066,17.5591617511586));
#9794=CARTESIAN_POINT('Ctrl Pts',(4.40715765450393,-2.64133925662669,17.5485584336382));
#9795=CARTESIAN_POINT('Ctrl Pts',(4.34626128713217,-2.7403876877419,17.5423290476631));
#9796=CARTESIAN_POINT('Ctrl Pts',(4.18416721160263,-2.98502157341648,17.5265954811246));
#9797=CARTESIAN_POINT('Ctrl Pts',(4.07869897615658,-3.12759034978395,17.5171007480445));
#9798=CARTESIAN_POINT('Ctrl Pts',(3.84963645989993,-3.40588770933626,17.4975538640286));
#9799=CARTESIAN_POINT('Ctrl Pts',(3.72571187768934,-3.54102149480902,17.4875067109068));
#9800=CARTESIAN_POINT('Ctrl Pts',(3.42427514565471,-3.83634668577909,17.4643662207096));
#9801=CARTESIAN_POINT('Ctrl Pts',(3.24225257793722,-3.99136898997188,17.4513075558077));
#9802=CARTESIAN_POINT('Ctrl Pts',(2.87014197802326,-4.2659710436289,17.426228460559));
#9803=CARTESIAN_POINT('Ctrl Pts',(2.6816964310369,-4.38688170404235,17.4142190445261));
#9804=CARTESIAN_POINT('Ctrl Pts',(2.30674190297485,-4.59424521869185,17.3912439148772));
#9805=CARTESIAN_POINT('Ctrl Pts',(2.12175088500714,-4.68255458339153,17.3802934988848));
#9806=CARTESIAN_POINT('Ctrl Pts',(1.79663375006475,-4.81452456928245,17.3612751315745));
#9807=CARTESIAN_POINT('Ctrl Pts',(1.65900102015976,-4.86366668708399,17.3532828890041));
#9808=CARTESIAN_POINT('Ctrl Pts',(1.2358383332995,-4.99470336099618,17.3290011250798));
#9809=CARTESIAN_POINT('Ctrl Pts',(0.945123498846985,-5.05777693692968,17.31274279804));
#9810=CARTESIAN_POINT('Ctrl Pts',(0.431998916036982,-5.12329363451995,17.2847233468242));
#9811=CARTESIAN_POINT('Ctrl Pts',(0.211838217465618,-5.13710889563219,17.272902084057));
#9812=CARTESIAN_POINT('Ctrl Pts',(-0.196746411185736,-5.13643033591684,
17.2509961470586));
#9813=CARTESIAN_POINT('Ctrl Pts',(-0.384799276862744,-5.12577338476215,
17.2409233903086));
#9814=CARTESIAN_POINT('Ctrl Pts',(-0.705440872973576,-5.08985532941652,
17.2234419372848));
#9815=CARTESIAN_POINT('Ctrl Pts',(-0.838401333636091,-5.06965045985436,
17.2160934956458));
#9816=CARTESIAN_POINT('Ctrl Pts',(-1.28168693270424,-4.98437124144774,17.1913595633278));
#9817=CARTESIAN_POINT('Ctrl Pts',(-1.58675955301951,-4.89580245744769,17.1739926276419));
#9818=CARTESIAN_POINT('Ctrl Pts',(-2.09164237291725,-4.69703415192307,17.1446132711876));
#9819=CARTESIAN_POINT('Ctrl Pts',(-2.29589307964555,-4.60064941949856,17.1325188221545));
#9820=CARTESIAN_POINT('Ctrl Pts',(-2.65656459669882,-4.40043179080046,17.1104026466122));
#9821=CARTESIAN_POINT('Ctrl Pts',(-2.81490597897205,-4.3008646990373,17.1003943481458));
#9822=CARTESIAN_POINT('Ctrl Pts',(-3.10941204607132,-4.09243186596577,17.0808215241124));
#9823=CARTESIAN_POINT('Ctrl Pts',(-3.24616379704547,-3.98482882862778,17.0712887915749));
#9824=CARTESIAN_POINT('Ctrl Pts',(-3.56233202808911,-3.70895723318056,17.0482794560179));
#9825=CARTESIAN_POINT('Ctrl Pts',(-3.73564590013667,-3.53433551753394,17.0348392238272));
#9826=CARTESIAN_POINT('Ctrl Pts',(-3.99530004859555,-3.23219503921335,17.0132352581982));
#9827=CARTESIAN_POINT('Ctrl Pts',(-4.08959266601737,-3.11203153742824,17.0050069522831));
#9828=CARTESIAN_POINT('Ctrl Pts',(-4.32456907535156,-2.78342549388566,16.9833014808359));
#9829=CARTESIAN_POINT('Ctrl Pts',(-4.45554330830702,-2.56855711066458,16.9699079677962));
#9830=CARTESIAN_POINT('Ctrl Pts',(-4.61619745960899,-2.25544806061679,16.950888944624));
#9831=CARTESIAN_POINT('Ctrl Pts',(-4.65948979842799,-2.1645966928949,16.945415547154));
#9832=CARTESIAN_POINT('Ctrl Pts',(-4.82299626053955,-1.79379738452305,16.9232744878646));
#9833=CARTESIAN_POINT('Ctrl Pts',(-4.92087083109501,-1.50467191251198,16.9065229113958));
#9834=CARTESIAN_POINT('Ctrl Pts',(-5.0313610192208,-1.04824654846185,16.8809774766104));
#9835=CARTESIAN_POINT('Ctrl Pts',(-5.06242885400186,-0.886132218254847,
16.8720620011718));
#9836=CARTESIAN_POINT('Ctrl Pts',(-5.11967574179977,-0.483342487670679,
16.8501678933299));
#9837=CARTESIAN_POINT('Ctrl Pts',(-5.13675391529282,-0.241780142526097,
16.837267788286));
#9838=CARTESIAN_POINT('Ctrl Pts',(-5.13674999932672,8.31682109386084E-5,
16.8242476778055));
#9839=CARTESIAN_POINT('Ctrl Pts',(-5.13710816050031,7.20752253655782E-5,
16.8240415053031));
#9840=CARTESIAN_POINT('Ctrl Pts',(-5.13715779729353,0.0723514105409758,
16.8201215600253));
#9841=CARTESIAN_POINT('Ctrl Pts',(-5.1180136959542,0.998597169429349,16.7698867892109));
#9842=CARTESIAN_POINT('Ctrl Pts',(-4.82253505916112,1.98281728759478,16.7158779233678));
#9843=CARTESIAN_POINT('Ctrl Pts',(-4.33041692566161,2.76455369449908,16.6657890028017));
#9844=CARTESIAN_POINT('Ctrl Pts',(-4.2921400227931,2.82267100337914,16.6620149077712));
#9845=CARTESIAN_POINT('Origin',(0.,0.,0.));
#9846=CARTESIAN_POINT('',(-4.29183622825303,2.82247096572397,14.9120225013103));
#9847=CARTESIAN_POINT('',(-4.29193634902365,2.82253681971926,15.3889288619751));
#9848=CARTESIAN_POINT('',(-4.29183622825304,2.82247096572397,0.));
#9849=CARTESIAN_POINT('',(-5.13679173984141,-1.83418071718305E-5,15.5509584943052));
#9850=CARTESIAN_POINT('Ctrl Pts',(-4.29193634902365,2.82253681971926,15.3889288619751));
#9851=CARTESIAN_POINT('Ctrl Pts',(-4.37956752146452,2.68958806914296,15.397563331971));
#9852=CARTESIAN_POINT('Ctrl Pts',(-4.8888867266577,1.83254938415906,15.4515732081804));
#9853=CARTESIAN_POINT('Ctrl Pts',(-5.13701666034835,0.836615721865797,15.5055830843898));
#9854=CARTESIAN_POINT('Ctrl Pts',(-5.13718616213208,-1.8274961578194E-5,
15.5509584906033));
#9855=CARTESIAN_POINT('Ctrl Pts',(-5.13674999996723,-1.83488811297034E-5,
15.5509584946969));
#9856=CARTESIAN_POINT('Ctrl Pts',(-5.13674993810036,-0.0173379132944814,
15.5518979126546));
#9857=CARTESIAN_POINT('Ctrl Pts',(-5.13666228124092,-0.034657405979478,
15.5528373306123));
#9858=CARTESIAN_POINT('Ctrl Pts',(-5.13648703461004,-0.0519760116108816,
15.55377674857));
#9859=CARTESIAN_POINT('Ctrl Pts',(-5.13498191205194,-0.200718523118732,
15.5618450301256));
#9860=CARTESIAN_POINT('Ctrl Pts',(-5.12701123425339,-0.349423111989173,
15.5699133116812));
#9861=CARTESIAN_POINT('Ctrl Pts',(-5.11259965267357,-0.497519199611531,
15.5779815932369));
#9862=CARTESIAN_POINT('Ctrl Pts',(-5.09819097957807,-0.64558539910911,15.5860482464861));
#9863=CARTESIAN_POINT('Ctrl Pts',(-5.07734402803056,-0.793043013100553,
15.5941148997355));
#9864=CARTESIAN_POINT('Ctrl Pts',(-5.05013535894052,-0.939326045033739,
15.6021815529848));
#9865=CARTESIAN_POINT('Ctrl Pts',(-5.02292570899642,-1.08561435037093,15.6102484970315));
#9866=CARTESIAN_POINT('Ctrl Pts',(-4.98935393939874,-1.23072766280729,15.6183154410782));
#9867=CARTESIAN_POINT('Ctrl Pts',(-4.94954793737664,-1.37410908522963,15.626382385125));
#9868=CARTESIAN_POINT('Ctrl Pts',(-4.90974434327348,-1.51748183431567,15.6344488411914));
#9869=CARTESIAN_POINT('Ctrl Pts',(-4.86370736054753,-1.65912258423355,15.6425152972578));
#9870=CARTESIAN_POINT('Ctrl Pts',(-4.81161506599276,-1.79848853741454,15.6505817533242));
#9871=CARTESIAN_POINT('Ctrl Pts',(-4.75950977124494,-1.93788927086987,15.6586502224615));
#9872=CARTESIAN_POINT('Ctrl Pts',(-4.7013462603938,-2.07501376276413,15.6667186915989));
#9873=CARTESIAN_POINT('Ctrl Pts',(-4.63735142535981,-2.20933752971639,15.6747871607363));
#9874=CARTESIAN_POINT('Ctrl Pts',(-4.58993691686327,-2.30885955186182,15.6807651822167));
#9875=CARTESIAN_POINT('Ctrl Pts',(-4.53932232389019,-2.40684448201293,15.686743203697));
#9876=CARTESIAN_POINT('Ctrl Pts',(-4.48561650980242,-2.50308711184569,15.6927212251774));
#9877=CARTESIAN_POINT('Ctrl Pts',(-4.41313205475769,-2.63298169949865,15.7007895067334));
#9878=CARTESIAN_POINT('Ctrl Pts',(-4.33498817017062,-2.75974967557468,15.7088577882893));
#9879=CARTESIAN_POINT('Ctrl Pts',(-4.25147948462556,-2.8829017940797,15.7169260698452));
#9880=CARTESIAN_POINT('Ctrl Pts',(-4.16798765244924,-3.0060290585465,15.7249927230947));
#9881=CARTESIAN_POINT('Ctrl Pts',(-4.07913336499658,-3.12554164748738,15.7330593763443));
#9882=CARTESIAN_POINT('Ctrl Pts',(-3.98525464170453,-3.24097917353267,15.7411260295938));
#9883=CARTESIAN_POINT('Ctrl Pts',(-3.89137253414861,-3.35642086102195,15.7491929736407));
#9884=CARTESIAN_POINT('Ctrl Pts',(-3.79246583420825,-3.46778693246239,15.7572599176875));
#9885=CARTESIAN_POINT('Ctrl Pts',(-3.68891327886389,-3.57464954695165,15.7653268617344));
#9886=CARTESIAN_POINT('Ctrl Pts',(-3.58536698755379,-3.6815056971767,15.7733933178008));
#9887=CARTESIAN_POINT('Ctrl Pts',(-3.47717563402646,-3.78385869829883,15.7814597738673));
#9888=CARTESIAN_POINT('Ctrl Pts',(-3.36475528239498,-3.88131710274941,15.7895262299338));
#9889=CARTESIAN_POINT('Ctrl Pts',(-3.25230687505414,-3.97879982899432,15.7975946990712));
#9890=CARTESIAN_POINT('Ctrl Pts',(-3.13562761053602,-4.07138530033998,15.8056631682087));
#9891=CARTESIAN_POINT('Ctrl Pts',(-3.01516765674759,-4.1587215059683,15.8137316373462));
#9892=CARTESIAN_POINT('Ctrl Pts',(-2.92591749306916,-4.22342990408932,15.8197096588255));
#9893=CARTESIAN_POINT('Ctrl Pts',(-2.83459264143782,-4.28525752760166,15.8256876803049));
#9894=CARTESIAN_POINT('Ctrl Pts',(-2.74138687527713,-4.34407626113519,15.8316657017843));
#9895=CARTESIAN_POINT('Ctrl Pts',(-2.61559101345333,-4.42346140629326,15.83973398334));
#9896=CARTESIAN_POINT('Ctrl Pts',(-2.48632132122764,-4.4973933555963,15.8478022648957));
#9897=CARTESIAN_POINT('Ctrl Pts',(-2.35407058924334,-4.56558344829656,15.8558705464515));
#9898=CARTESIAN_POINT('Ctrl Pts',(-2.22184654754109,-4.63375977916141,15.8639371997008));
#9899=CARTESIAN_POINT('Ctrl Pts',(-2.0866429603596,-4.69619641365086,15.8720038529502));
#9900=CARTESIAN_POINT('Ctrl Pts',(-1.94897691417263,-4.75265079198147,15.8800705061996));
#9901=CARTESIAN_POINT('Ctrl Pts',(-1.81130590521841,-4.809107205454,15.8881374502463));
#9902=CARTESIAN_POINT('Ctrl Pts',(-1.67117256443708,-4.85958080213363,15.896204394293));
#9903=CARTESIAN_POINT('Ctrl Pts',(-1.52911416225848,-4.90387708260317,15.9042713383398));
#9904=CARTESIAN_POINT('Ctrl Pts',(-1.38706435338487,-4.94817068353075,15.9123377944061));
#9905=CARTESIAN_POINT('Ctrl Pts',(-1.24309003234839,-4.98628761806158,15.9204042504725));
#9906=CARTESIAN_POINT('Ctrl Pts',(-1.09774383587324,-5.01808320310677,15.9284707065389));
#9907=CARTESIAN_POINT('Ctrl Pts',(-0.952361366689644,-5.04988672308259,
15.9365391756762));
#9908=CARTESIAN_POINT('Ctrl Pts',(-0.805606661340605,-5.07536566987868,
15.9446076448136));
#9909=CARTESIAN_POINT('Ctrl Pts',(-0.6580434362872,-5.0944263070987,15.9526761139509));
#9910=CARTESIAN_POINT('Ctrl Pts',(-0.548712147532794,-5.10854855219731,
15.9586541354311));
#9911=CARTESIAN_POINT('Ctrl Pts',(-0.438937267950764,-5.11914852251498,
15.9646321569114));
#9912=CARTESIAN_POINT('Ctrl Pts',(-0.328950249182865,-5.12620642347365,
15.9706101783916));
#9913=CARTESIAN_POINT('Ctrl Pts',(-0.180505443845024,-5.1357321724724,15.9786784599477));
#9914=CARTESIAN_POINT('Ctrl Pts',(-0.0316191457278236,-5.13880734577375,
15.9867467415038));
#9915=CARTESIAN_POINT('Ctrl Pts',(0.117137809096552,-5.13541422829552,15.9948150230599));
#9916=CARTESIAN_POINT('Ctrl Pts',(0.265864742422901,-5.13202179560187,16.0028816763096));
#9917=CARTESIAN_POINT('Ctrl Pts',(0.414462053806652,-5.12216368398763,16.0109483295594));
#9918=CARTESIAN_POINT('Ctrl Pts',(0.562359628422229,-5.10587428466671,16.0190149828091));
#9919=CARTESIAN_POINT('Ctrl Pts',(0.710262534644763,-5.08958429812403,16.0270819268562));
#9920=CARTESIAN_POINT('Ctrl Pts',(0.857465324196741,-5.06686259241309,16.0351488709033));
#9921=CARTESIAN_POINT('Ctrl Pts',(1.00340315167862,-5.0377954184049,16.0432158149504));
#9922=CARTESIAN_POINT('Ctrl Pts',(1.14933215118369,-5.00873000270943,16.0512822710171));
#9923=CARTESIAN_POINT('Ctrl Pts',(1.29399601721132,-4.97331995210457,16.0593487270838));
#9924=CARTESIAN_POINT('Ctrl Pts',(1.43684024440614,-4.93170261416429,16.0674151831505));
#9925=CARTESIAN_POINT('Ctrl Pts',(1.57972011991608,-4.89007489016917,16.0754836522882));
#9926=CARTESIAN_POINT('Ctrl Pts',(1.72077913104728,-4.84223687544647,16.0835521214259));
#9927=CARTESIAN_POINT('Ctrl Pts',(1.85947741742588,-4.78837595606101,16.0916205905636));
#9928=CARTESIAN_POINT('Ctrl Pts',(1.9622405712331,-4.74846978210946,16.097598612042));
#9929=CARTESIAN_POINT('Ctrl Pts',(2.06370809445908,-4.70525837990009,16.1035766335203));
#9930=CARTESIAN_POINT('Ctrl Pts',(2.16366727307025,-4.65883510053154,16.1095546549987));
#9931=CARTESIAN_POINT('Ctrl Pts',(2.29857792870794,-4.59617957311044,16.1176229365539));
#9932=CARTESIAN_POINT('Ctrl Pts',(2.43079012661376,-4.52764840371988,16.1256912181092));
#9933=CARTESIAN_POINT('Ctrl Pts',(2.55979412531764,-4.45349914095527,16.1337594996644));
#9934=CARTESIAN_POINT('Ctrl Pts',(2.68877208898131,-4.37936484268057,16.1418261529133));
#9935=CARTESIAN_POINT('Ctrl Pts',(2.81454285834313,-4.29961487788759,16.1498928061621));
#9936=CARTESIAN_POINT('Ctrl Pts',(2.93662225445447,-4.21455220600514,16.1579594594109));
#9937=CARTESIAN_POINT('Ctrl Pts',(3.05870605144513,-4.12948646767112,16.1660264034572));
#9938=CARTESIAN_POINT('Ctrl Pts',(3.17709793515927,-4.03910782512636,16.1740933475034));
#9939=CARTESIAN_POINT('Ctrl Pts',(3.29134316504544,-3.9437622560708,16.1821602915496));
#9940=CARTESIAN_POINT('Ctrl Pts',(3.40558148408308,-3.84842245459773,16.1902267476155));
#9941=CARTESIAN_POINT('Ctrl Pts',(3.5156733974926,-3.74811654043978,16.1982932036813));
#9942=CARTESIAN_POINT('Ctrl Pts',(3.62119769074238,-3.64323041366616,16.2063596597472));
#9943=CARTESIAN_POINT('Ctrl Pts',(3.726748318716,-3.53831811143001,16.214428128884));
#9944=CARTESIAN_POINT('Ctrl Pts',(3.82772881343532,-3.42882354555812,16.2224965980209));
#9945=CARTESIAN_POINT('Ctrl Pts',(3.92375476038674,-3.31516954963731,16.2305650671577));
#9946=CARTESIAN_POINT('Ctrl Pts',(3.99490148773244,-3.23096199828018,16.2365430886405));
#9947=CARTESIAN_POINT('Ctrl Pts',(4.06332917017486,-3.14447190726514,16.2425211101232));
#9948=CARTESIAN_POINT('Ctrl Pts',(4.12889567986362,-3.05588301924395,16.2484991316059));
#9949=CARTESIAN_POINT('Ctrl Pts',(4.21738801171579,-2.93631836170157,16.2565674131628));
#9950=CARTESIAN_POINT('Ctrl Pts',(4.30069967843036,-2.81288517065804,16.2646356947197));
#9951=CARTESIAN_POINT('Ctrl Pts',(4.37850628149582,-2.68605348148574,16.2727039762766));
#9952=CARTESIAN_POINT('Ctrl Pts',(4.45629718196249,-2.55924738894728,16.280770629527));
#9953=CARTESIAN_POINT('Ctrl Pts',(4.52858506228784,-2.42904444859185,16.2888372827775));
#9954=CARTESIAN_POINT('Ctrl Pts',(4.5950896969485,-2.29594234237223,16.296903936028));
#9955=CARTESIAN_POINT('Ctrl Pts',(4.66159672905597,-2.16283543791232,16.3049708800759));
#9956=CARTESIAN_POINT('Ctrl Pts',(4.72231994697923,-2.02682945285514,16.3130378241237));
#9957=CARTESIAN_POINT('Ctrl Pts',(4.77702555701905,-1.8884457604302,16.3211047681716));
#9958=CARTESIAN_POINT('Ctrl Pts',(4.83172785784242,-1.75007043902227,16.329171224239));
#9959=CARTESIAN_POINT('Ctrl Pts',(4.88041315809126,-1.6093180061423,16.3372376803065));
#9960=CARTESIAN_POINT('Ctrl Pts',(4.92289620416854,-1.46672885206603,16.345304136374));
#9961=CARTESIAN_POINT('Ctrl Pts',(4.96538985234736,-1.3241041133312,16.3533726055124));
#9962=CARTESIAN_POINT('Ctrl Pts',(5.00167805827274,-1.17964205468374,16.3614410746508));
#9963=CARTESIAN_POINT('Ctrl Pts',(5.03162555347915,-1.03389789248049,16.3695095437893));
#9964=CARTESIAN_POINT('Ctrl Pts',(5.05381399671215,-0.925914368406157,16.3754875652639));
#9965=CARTESIAN_POINT('Ctrl Pts',(5.07252274191634,-0.817227357277184,16.3814655867385));
#9966=CARTESIAN_POINT('Ctrl Pts',(5.08771489077454,-0.708066206432031,16.3874436082131));
#9967=CARTESIAN_POINT('Ctrl Pts',(5.10821908851433,-0.560736039822586,16.3955118897678));
#9968=CARTESIAN_POINT('Ctrl Pts',(5.122323189392,-0.412487394673058,16.4035801713225));
#9969=CARTESIAN_POINT('Ctrl Pts',(5.12996720927492,-0.26388822304926,16.4116484528772));
#9970=CARTESIAN_POINT('Ctrl Pts',(5.13760968647414,-0.11531904108037,16.4197151061255));
#9971=CARTESIAN_POINT('Ctrl Pts',(5.13879466669358,0.0336001958547929,16.4277817593738));
#9972=CARTESIAN_POINT('Ctrl Pts',(5.13351418218723,0.182298392155877,16.4358484126221));
#9973=CARTESIAN_POINT('Ctrl Pts',(5.12823350732299,0.331001948925982,16.4439153566678));
#9974=CARTESIAN_POINT('Ctrl Pts',(5.11648690929533,0.479484118190521,16.4519823007134));
#9975=CARTESIAN_POINT('Ctrl Pts',(5.09831852795476,0.627175214763183,16.4600492447591));
#9976=CARTESIAN_POINT('Ctrl Pts',(5.08015124564415,0.774857377301651,16.4681157008244));
#9977=CARTESIAN_POINT('Ctrl Pts',(5.05556299840837,0.921748234430995,16.4761821568897));
#9978=CARTESIAN_POINT('Ctrl Pts',(5.02464964873995,1.06728462460466,16.484248612955));
#9979=CARTESIAN_POINT('Ctrl Pts',(4.99372858431214,1.21285733495211,16.4923170820914));
#9980=CARTESIAN_POINT('Ctrl Pts',(4.95647933147031,1.3570745788207,16.5003855512277));
#9981=CARTESIAN_POINT('Ctrl Pts',(4.91304873918663,1.4993840898438,16.508454020364));
#9982=CARTESIAN_POINT('Ctrl Pts',(4.88087051436959,1.60482284162026,16.5144320418494));
#9983=CARTESIAN_POINT('Ctrl Pts',(4.84530010708197,1.70921455443603,16.5204100633349));
#9984=CARTESIAN_POINT('Ctrl Pts',(4.80641484242291,1.81234017917077,16.5263880848203));
#9985=CARTESIAN_POINT('Ctrl Pts',(4.75393305318738,1.95152445243119,16.5344563663762));
#9986=CARTESIAN_POINT('Ctrl Pts',(4.69539174482462,2.08845327215774,16.5425246479321));
#9987=CARTESIAN_POINT('Ctrl Pts',(4.63100996858054,2.22259920665146,16.550592929488));
#9988=CARTESIAN_POINT('Ctrl Pts',(4.56664118559372,2.35671806838113,16.5586595827375));
#9989=CARTESIAN_POINT('Ctrl Pts',(4.49643442939982,2.48805486710282,16.566726235987));
#9990=CARTESIAN_POINT('Ctrl Pts',(4.42065593215064,2.61610429685848,16.5747928892365));
#9991=CARTESIAN_POINT('Ctrl Pts',(4.34487470313824,2.74415834270886,16.5828598332834));
#9992=CARTESIAN_POINT('Ctrl Pts',(4.26352149645798,2.86892449566634,16.5909267773303));
#9993=CARTESIAN_POINT('Ctrl Pts',(4.17690762651911,2.98992361809236,16.5989937213771));
#9994=CARTESIAN_POINT('Ctrl Pts',(4.09029899597056,3.11091542111755,16.6070601774436));
#9995=CARTESIAN_POINT('Ctrl Pts',(3.9984305321498,3.22814038079684,16.6151266335101));
#9996=CARTESIAN_POINT('Ctrl Pts',(3.90165584736817,3.34114983369464,16.6231930895766));
#9997=CARTESIAN_POINT('Ctrl Pts',(3.80485701142197,3.45418748931822,16.631261558714));
#9998=CARTESIAN_POINT('Ctrl Pts',(3.70314972283527,3.56300728402921,16.6393300278515));
#9999=CARTESIAN_POINT('Ctrl Pts',(3.5969271539055,3.66719451515696,16.6473984969889));
#10000=CARTESIAN_POINT('Ctrl Pts',(3.51822563223433,3.74438803166739,16.6533765184684));
#10001=CARTESIAN_POINT('Ctrl Pts',(3.43704628064773,3.81903919663655,16.659354539948));
#10002=CARTESIAN_POINT('Ctrl Pts',(3.35356179983878,3.89099265190287,16.6653325614275));
#10003=CARTESIAN_POINT('Ctrl Pts',(3.24088634369147,3.9881051728762,16.6734008429876));
#10004=CARTESIAN_POINT('Ctrl Pts',(3.12396894054375,4.0803380700494,16.6814691245477));
#10005=CARTESIAN_POINT('Ctrl Pts',(3.00325428376368,4.16733299240115,16.6895374061078));
#10006=CARTESIAN_POINT('Ctrl Pts',(2.88256398910342,4.25431035780681,16.6976040593616));
#10007=CARTESIAN_POINT('Ctrl Pts',(2.75807823807291,4.33605166393318,16.7056707126153));
#10008=CARTESIAN_POINT('Ctrl Pts',(2.63027256922376,4.41224056167488,16.7137373658691));
#10009=CARTESIAN_POINT('Ctrl Pts',(2.50246229306723,4.48843220597449,16.7218043099202));
#10010=CARTESIAN_POINT('Ctrl Pts',(2.37133214197831,4.55907086861316,16.7298712539713));
#10011=CARTESIAN_POINT('Ctrl Pts',(2.23738472272639,4.62388474824044,16.7379381980224));
#10012=CARTESIAN_POINT('Ctrl Pts',(2.10344540613535,4.68869470718832,16.7460046540932));
#10013=CARTESIAN_POINT('Ctrl Pts',(1.96668946065899,4.7476804445871,16.7540711101639));
#10014=CARTESIAN_POINT('Ctrl Pts',(1.82764205620876,4.80061715583289,16.7621375662346));
#10015=CARTESIAN_POINT('Ctrl Pts',(1.68855995098234,4.85356707800466,16.7702060353763));
#10016=CARTESIAN_POINT('Ctrl Pts',(1.54718555337111,4.90046483909873,16.778274504518));
#10017=CARTESIAN_POINT('Ctrl Pts',(1.40406252411984,4.94113438299974,16.7863429736596));
#10018=CARTESIAN_POINT('Ctrl Pts',(1.29802102789186,4.97126691519064,16.792320995118));
#10019=CARTESIAN_POINT('Ctrl Pts',(1.19102001986929,4.99798147585057,16.7982990165764));
#10020=CARTESIAN_POINT('Ctrl Pts',(1.08328548092466,5.02122426598512,16.8042770380347));
#10021=CARTESIAN_POINT('Ctrl Pts',(0.937880751627644,5.05259407218404,16.8123453195757));
#10022=CARTESIAN_POINT('Ctrl Pts',(0.791085612671925,5.07764948186624,16.8204136011166));
#10023=CARTESIAN_POINT('Ctrl Pts',(0.643462006519024,5.09628857195769,16.8284818826575));
#10024=CARTESIAN_POINT('Ctrl Pts',(0.495868193137679,5.11492390038684,16.836548535892));
#10025=CARTESIAN_POINT('Ctrl Pts',(0.347446574330549,5.1271454511757,16.8446151891264));
#10026=CARTESIAN_POINT('Ctrl Pts',(0.198766083575153,5.13290294146696,16.8526818423609));
#10027=CARTESIAN_POINT('Ctrl Pts',(0.0500802329885989,5.13866063931186,
16.8607487863928));
#10028=CARTESIAN_POINT('Ctrl Pts',(-0.0988641776145617,5.13795379376828,
16.8688157304246));
#10029=CARTESIAN_POINT('Ctrl Pts',(-0.247495758396923,5.13078419075248,
16.8768826744565));
#10030=CARTESIAN_POINT('Ctrl Pts',(-0.396118348255007,5.1236150214356,16.8849491305081));
#10031=CARTESIAN_POINT('Ctrl Pts',(-0.544427815545846,5.1099838935302,16.8930155865596));
#10032=CARTESIAN_POINT('Ctrl Pts',(-0.691855441765988,5.08994465688958,
16.9010820426112));
#10033=CARTESIAN_POINT('Ctrl Pts',(-0.839319860141933,5.06990041924111,
16.909150511734));
#10034=CARTESIAN_POINT('Ctrl Pts',(-0.985901669447363,5.04344492126959,
16.9172189808567));
#10035=CARTESIAN_POINT('Ctrl Pts',(-1.13103923659801,5.01068366670415,16.9252874499795));
#10036=CARTESIAN_POINT('Ctrl Pts',(-1.23857332906836,4.98641047646784,16.9312654715336));
#10037=CARTESIAN_POINT('Ctrl Pts',(-1.34531473632737,4.95867681758785,16.9372434930878));
#10038=CARTESIAN_POINT('Ctrl Pts',(-1.45103927964805,4.92754356362463,16.9432215146419));
#10039=CARTESIAN_POINT('Ctrl Pts',(-1.59373120185918,4.88552433409507,16.9512897962328));
#10040=CARTESIAN_POINT('Ctrl Pts',(-1.73462308709432,4.83729505542724,16.9593580778237));
#10041=CARTESIAN_POINT('Ctrl Pts',(-1.87317271602301,4.78303507602097,16.9674263594146));
#10042=CARTESIAN_POINT('Ctrl Pts',(-2.01169438345545,4.72878604713275,16.9754930126992));
#10043=CARTESIAN_POINT('Ctrl Pts',(-2.14787442960605,4.66850886626966,16.9835596659838));
#10044=CARTESIAN_POINT('Ctrl Pts',(-2.28118920234082,4.60243157316039,16.9916263192685));
#10045=CARTESIAN_POINT('Ctrl Pts',(-2.41450878097982,4.53635189801096,16.9996932633503));
#10046=CARTESIAN_POINT('Ctrl Pts',(-2.54496258125869,4.46447183581378,17.0077602074322));
#10047=CARTESIAN_POINT('Ctrl Pts',(-2.67204970527385,4.38706632444119,17.015827151514));
#10048=CARTESIAN_POINT('Ctrl Pts',(-2.79912914161421,4.30966549543438,17.0238936076154));
#10049=CARTESIAN_POINT('Ctrl Pts',(-2.9228420268321,4.22674005883158,17.0319600637167));
#10050=CARTESIAN_POINT('Ctrl Pts',(-3.0427147177022,4.13860939316317,17.040026519818));
#10051=CARTESIAN_POINT('Ctrl Pts',(-3.16261732408451,4.05045673354446,17.0480949889897));
#10052=CARTESIAN_POINT('Ctrl Pts',(-3.27867755390728,3.95709644480316,17.0561634581614));
#10053=CARTESIAN_POINT('Ctrl Pts',(-3.39045269856158,3.85888987421467,17.0642319273331));
#10054=CARTESIAN_POINT('Ctrl Pts',(-3.47326818461293,3.7861275002372,17.0702099486384));
#10055=CARTESIAN_POINT('Ctrl Pts',(-3.55373200387586,3.71070564241949,17.0761879699437));
#10056=CARTESIAN_POINT('Ctrl Pts',(-3.63167642287095,3.63278500906168,17.082165991249));
#10057=CARTESIAN_POINT('Ctrl Pts',(-3.73687374245287,3.52761979165358,17.0902341996702));
#10058=CARTESIAN_POINT('Ctrl Pts',(-3.83751941607202,3.41786264164616,17.0983024080914));
#10059=CARTESIAN_POINT('Ctrl Pts',(-3.93322312273905,3.30393045163648,17.1063706165126));
#10060=CARTESIAN_POINT('Ctrl Pts',(-4.02890965857688,3.19001870294767,17.1144373773636));
#10061=CARTESIAN_POINT('Ctrl Pts',(-4.11965578295557,3.07193366143052,17.1225041382147));
#10062=CARTESIAN_POINT('Ctrl Pts',(-4.20511075000905,2.95012612317818,17.1305708990657));
#10063=CARTESIAN_POINT('Ctrl Pts',(-4.23465580446763,2.90801259279815,17.1333598871944));
#10064=CARTESIAN_POINT('Ctrl Pts',(-4.26356874076661,2.86545437577467,17.1361488753231));
#10065=CARTESIAN_POINT('Ctrl Pts',(-4.29183622825303,2.82247096572397,17.1389378634518));
#10066=CARTESIAN_POINT('',(-5.13670694023125,8.22511334899522E-6,15.0740415053031));
#10067=CARTESIAN_POINT('Ctrl Pts',(-4.2921400227931,2.82267100337914,16.6620149077712));
#10068=CARTESIAN_POINT('Ctrl Pts',(-3.86069158380266,3.47775593229212,16.6194741772661));
#10069=CARTESIAN_POINT('Ctrl Pts',(-2.64190503851504,4.63775144658851,16.5306186212244));
#10070=CARTESIAN_POINT('Ctrl Pts',(-0.171207780293172,5.35198763020908,
16.3954482396483));
#10071=CARTESIAN_POINT('Ctrl Pts',(2.41020538539942,4.78163086175811,16.2565037630408));
#10072=CARTESIAN_POINT('Ctrl Pts',(4.40413631567179,3.04576213958252,16.1175592864337));
#10073=CARTESIAN_POINT('Ctrl Pts',(5.32456875345049,0.567495627922317,15.9786148098264));
#10074=CARTESIAN_POINT('Ctrl Pts',(4.94714932645596,-2.04909668870878,15.8396703332193));
#10075=CARTESIAN_POINT('Ctrl Pts',(3.36387318580941,-4.16622621658075,15.7007258566122));
#10076=CARTESIAN_POINT('Ctrl Pts',(0.96066039128185,-5.26784731276012,15.5617813800049));
#10077=CARTESIAN_POINT('Ctrl Pts',(-1.67671125027514,-5.08544226996355,
15.4228369033978));
#10078=CARTESIAN_POINT('Ctrl Pts',(-3.90538823060865,-3.66347191420326,
15.2838924267906));
#10079=CARTESIAN_POINT('Ctrl Pts',(-4.97373718467484,-1.72639559785503,
15.1676272940924));
#10080=CARTESIAN_POINT('Ctrl Pts',(-5.13628689006179,-0.435997775582432,
15.0976769869299));
#10081=CARTESIAN_POINT('Ctrl Pts',(-5.13631118563065,8.22447965037609E-6,
15.0740415053031));
#10082=CARTESIAN_POINT('Ctrl Pts',(-5.13674999999342,8.22518229806563E-6,
15.0740415053031));
#10083=CARTESIAN_POINT('Ctrl Pts',(-5.13674975849047,0.150830448247622,
15.0658662706561));
#10084=CARTESIAN_POINT('Ctrl Pts',(-5.13010264657814,0.301636878576586,
15.057691036009));
#10085=CARTESIAN_POINT('Ctrl Pts',(-5.11683883531417,0.451841671297237,
15.049515801362));
#10086=CARTESIAN_POINT('Ctrl Pts',(-5.10357056040029,0.602097012204711,
15.0413378155159));
#10087=CARTESIAN_POINT('Ctrl Pts',(-5.08368116440342,0.751750000235891,
15.0331598296698));
#10088=CARTESIAN_POINT('Ctrl Pts',(-5.05725273714425,0.900219592736657,
15.0249818438237));
#10089=CARTESIAN_POINT('Ctrl Pts',(-5.03680889000711,1.01506901695079,15.0186557204079));
#10090=CARTESIAN_POINT('Ctrl Pts',(-5.01245321882611,1.1292103786262,15.0123295969921));
#10091=CARTESIAN_POINT('Ctrl Pts',(-4.98424474906023,1.24237870392465,15.0060034735762));
#10092=CARTESIAN_POINT('Ctrl Pts',(-4.94826626642743,1.3867192037861,14.9979348217373));
#10093=CARTESIAN_POINT('Ctrl Pts',(-4.9060069054024,1.52952246934126,14.9898661698984));
#10094=CARTESIAN_POINT('Ctrl Pts',(-4.85762305893994,1.67023913849334,14.9817975180595));
#10095=CARTESIAN_POINT('Ctrl Pts',(-4.80925007919966,1.81092420352419,14.9737306783915));
#10096=CARTESIAN_POINT('Ctrl Pts',(-4.75475546663133,1.94952329448943,14.9656638387235));
#10097=CARTESIAN_POINT('Ctrl Pts',(-4.69434503816343,2.08550359030387,14.9575969990554));
#10098=CARTESIAN_POINT('Ctrl Pts',(-4.63393365557878,2.22148603377861,14.9495300319805));
#10099=CARTESIAN_POINT('Ctrl Pts',(-4.56760640109698,2.35484929530895,14.9414630649055));
#10100=CARTESIAN_POINT('Ctrl Pts',(-4.49561689424886,2.48508134728911,14.9333960978305));
#10101=CARTESIAN_POINT('Ctrl Pts',(-4.43203766392339,2.60009885457767,14.9262715656571));
#10102=CARTESIAN_POINT('Ctrl Pts',(-4.36404265913438,2.7126742026278,14.9191470334837));
#10103=CARTESIAN_POINT('Ctrl Pts',(-4.29183622825303,2.82247096572397,14.9120225013103));
#10104=CARTESIAN_POINT('Origin',(0.,0.,0.));
#10105=CARTESIAN_POINT('',(-4.29183623954907,2.82247094854727,13.1619495546845));
#10106=CARTESIAN_POINT('',(-4.29183622825304,2.82247096572396,13.6389404220384));
#10107=CARTESIAN_POINT('',(-4.29183622825304,2.82247096572397,0.));
#10108=CARTESIAN_POINT('',(-5.13674999929672,8.50009777041742E-5,13.8009584946969));
#10109=CARTESIAN_POINT('Ctrl Pts',(-4.29183622825304,2.82247096572396,13.6389404220384));
#10110=CARTESIAN_POINT('Ctrl Pts',(-4.37357958870702,2.69817239185872,13.6470067765585));
#10111=CARTESIAN_POINT('Ctrl Pts',(-4.4499279442811,2.57030743963229,13.6550731310786));
#10112=CARTESIAN_POINT('Ctrl Pts',(-4.5205860970387,2.43936506119121,13.6631394855987));
#10113=CARTESIAN_POINT('Ctrl Pts',(-4.59124771236917,2.3084162659743,13.6712062354071));
#10114=CARTESIAN_POINT('Ctrl Pts',(-4.65621840730926,2.17439003276196,13.6792729852155));
#10115=CARTESIAN_POINT('Ctrl Pts',(-4.71524868839109,2.0378003751904,13.6873397350239));
#10116=CARTESIAN_POINT('Ctrl Pts',(-4.77427676683697,1.90121581427913,13.6954061838323));
#10117=CARTESIAN_POINT('Ctrl Pts',(-4.8273647452265,1.76206832492696,13.7034726326407));
#10118=CARTESIAN_POINT('Ctrl Pts',(-4.87431107211784,1.62089238838654,13.7115390814491));
#10119=CARTESIAN_POINT('Ctrl Pts',(-4.92126820165559,1.47968396637121,13.7196073863983));
#10120=CARTESIAN_POINT('Ctrl Pts',(-4.96208075214552,1.33644647894745,13.7276756913476));
#10121=CARTESIAN_POINT('Ctrl Pts',(-4.99659670171705,1.191730658702,13.7357439962968));
#10122=CARTESIAN_POINT('Ctrl Pts',(-5.01335857333664,1.12145277180072,13.7396621817567));
#10123=CARTESIAN_POINT('Ctrl Pts',(-5.02863625144882,1.05082645350585,13.7435803672166));
#10124=CARTESIAN_POINT('Ctrl Pts',(-5.04241664468204,0.979915784102628,
13.7474985526766));
#10125=CARTESIAN_POINT('Ctrl Pts',(-5.07155666765262,0.829968064883282,
13.7557839486281));
#10126=CARTESIAN_POINT('Ctrl Pts',(-5.09400667909746,0.678705261588683,
13.7640693445797));
#10127=CARTESIAN_POINT('Ctrl Pts',(-5.10967360315828,0.526722157961372,
13.7723547405312));
#10128=CARTESIAN_POINT('Ctrl Pts',(-5.12533565923321,0.374786278128614,
13.7806375620661));
#10129=CARTESIAN_POINT('Ctrl Pts',(-5.1342188057037,0.222130834218837,13.788920383601));
#10130=CARTESIAN_POINT('Ctrl Pts',(-5.13628175387216,0.0693563792299268,
13.7972032051359));
#10131=CARTESIAN_POINT('Ctrl Pts',(-5.13659352233936,0.0462679379463962,
13.7984549683229));
#10132=CARTESIAN_POINT('Ctrl Pts',(-5.13674961718268,0.0231767855100868,
13.7997067315099));
#10133=CARTESIAN_POINT('Ctrl Pts',(-5.13674999929672,8.50009777041742E-5,
13.8009584946969));
#10134=CARTESIAN_POINT('Ctrl Pts',(-5.1364024164725,8.49952260370549E-5,
13.8009584946969));
#10135=CARTESIAN_POINT('Ctrl Pts',(-5.13609293759186,-0.525535431478061,
13.8294533395592));
#10136=CARTESIAN_POINT('Ctrl Pts',(-4.92543237478305,-1.90572893214436,
13.9042630099572));
#10137=CARTESIAN_POINT('Ctrl Pts',(-3.70837745769343,-3.86277367330787,
14.0253875058909));
#10138=CARTESIAN_POINT('Ctrl Pts',(-1.40835915724232,-5.16619863188995,
14.1643319824982));
#10139=CARTESIAN_POINT('Ctrl Pts',(1.23494357489379,-5.21037409278427,14.3032764591053));
#10140=CARTESIAN_POINT('Ctrl Pts',(3.57723154024265,-3.98453238503892,14.4422209357125));
#10141=CARTESIAN_POINT('Ctrl Pts',(5.04757722440252,-1.78746971544192,14.5811654123197));
#10142=CARTESIAN_POINT('Ctrl Pts',(5.28758711676144,0.845284746454227,14.7201098889269));
#10143=CARTESIAN_POINT('Ctrl Pts',(4.23875933654995,3.2720029197328,14.8590543655341));
#10144=CARTESIAN_POINT('Ctrl Pts',(2.15674333697306,4.90117761342644,14.9979988421412));
#10145=CARTESIAN_POINT('Ctrl Pts',(-0.450974083946612,5.33570109690734,
15.1369433187485));
#10146=CARTESIAN_POINT('Ctrl Pts',(-2.79354640822019,4.52347794157121,15.2672533253597));
#10147=CARTESIAN_POINT('Ctrl Pts',(-3.90951869796817,3.40271790699677,15.3512485064353));
#10148=CARTESIAN_POINT('Ctrl Pts',(-4.29193634902365,2.82253681971926,15.3889288619751));
#10149=CARTESIAN_POINT('',(-5.13674999926869,-8.66784045078238E-5,13.3240415053031));
#10150=CARTESIAN_POINT('Ctrl Pts',(-4.29183622825303,2.82247096572397,14.9120225013103));
#10151=CARTESIAN_POINT('Ctrl Pts',(-4.21006206974841,2.94681637096182,14.9039539315706));
#10152=CARTESIAN_POINT('Ctrl Pts',(-4.12288583257787,3.06759728781872,14.8958853618309));
#10153=CARTESIAN_POINT('Ctrl Pts',(-4.03064505549953,3.18435252430965,14.8878167920912));
#10154=CARTESIAN_POINT('Ctrl Pts',(-3.95154325620129,3.28447688987175,14.8808975270505));
#10155=CARTESIAN_POINT('Ctrl Pts',(-3.86871774776158,3.38164113034757,14.8739782620097));
#10156=CARTESIAN_POINT('Ctrl Pts',(-3.78240512199835,3.47557362971649,14.8670589969689));
#10157=CARTESIAN_POINT('Ctrl Pts',(-3.68175937965753,3.58510460557681,14.8589907154131));
#10158=CARTESIAN_POINT('Ctrl Pts',(-3.57633413088022,3.69028113992072,14.8509224338573));
#10159=CARTESIAN_POINT('Ctrl Pts',(-3.46652948335297,3.79069570178676,14.8428541523014));
#10160=CARTESIAN_POINT('Ctrl Pts',(-3.35674699613402,3.89108999841176,14.834787499052));
#10161=CARTESIAN_POINT('Ctrl Pts',(-3.2425871175593,3.9867240166137,14.8267208458025));
#10162=CARTESIAN_POINT('Ctrl Pts',(-3.12448546588943,4.07722836445859,14.8186541925531));
#10163=CARTESIAN_POINT('Ctrl Pts',(-3.00637955673554,4.16773597492353,14.8105872485062));
#10164=CARTESIAN_POINT('Ctrl Pts',(-2.88433185056216,4.25311334065131,14.8025203044594));
#10165=CARTESIAN_POINT('Ctrl Pts',(-2.75881002016174,4.33303217564273,14.7944533604126));
#10166=CARTESIAN_POINT('Ctrl Pts',(-2.63329578274698,4.4129461762355,14.7863869043462));
#10167=CARTESIAN_POINT('Ctrl Pts',(-2.50430812121457,4.48740212958203,14.7783204482798));
#10168=CARTESIAN_POINT('Ctrl Pts',(-2.37234257241721,4.55611581081922,14.7702539922134));
#10169=CARTESIAN_POINT('Ctrl Pts',(-2.24034409019586,4.62484664029563,14.7621855230759));
#10170=CARTESIAN_POINT('Ctrl Pts',(-2.10536652916291,4.68783218062042,14.7541170539385));
#10171=CARTESIAN_POINT('Ctrl Pts',(-1.96792944869695,4.74483448051155,14.7460485848011));
#10172=CARTESIAN_POINT('Ctrl Pts',(-1.86610073681253,4.78706813938064,14.7400705633214));
#10173=CARTESIAN_POINT('Ctrl Pts',(-1.76292238556871,4.8260182535111,14.7340925418416));
#10174=CARTESIAN_POINT('Ctrl Pts',(-1.65861260668985,4.86160516531624,14.7281145203618));
#10175=CARTESIAN_POINT('Ctrl Pts',(-1.51783013077032,4.90963530791749,14.720046238806));
#10176=CARTESIAN_POINT('Ctrl Pts',(-1.37493393765075,4.95155504608902,14.7119779572501));
#10177=CARTESIAN_POINT('Ctrl Pts',(-1.23047034706621,4.98719793947371,14.7039096756943));
#10178=CARTESIAN_POINT('Ctrl Pts',(-1.08603591151098,5.02283363956078,14.6958430224448));
#10179=CARTESIAN_POINT('Ctrl Pts',(-0.940035030750641,5.05219494285085,
14.6877763691954));
#10180=CARTESIAN_POINT('Ctrl Pts',(-0.793026960456183,5.07516588915965,
14.6797097159459));
#10181=CARTESIAN_POINT('Ctrl Pts',(-0.64601359062089,5.09813766355542,14.6716427718991));
#10182=CARTESIAN_POINT('Ctrl Pts',(-0.497993285043127,5.11471856514564,
14.6635758278523));
#10183=CARTESIAN_POINT('Ctrl Pts',(-0.349533781033704,5.12484406576593,
14.6555088838054));
#10184=CARTESIAN_POINT('Ctrl Pts',(-0.201083257540819,5.13496895388097,
14.647442427739));
#10185=CARTESIAN_POINT('Ctrl Pts',(-0.0521939190847952,5.13863920054417,
14.6393759716725));
#10186=CARTESIAN_POINT('Ctrl Pts',(0.0965631090010042,5.13584229980634,
14.6313095156061));
#10187=CARTESIAN_POINT('Ctrl Pts',(0.245357261005208,5.13304470107181,14.6232410464687));
#10188=CARTESIAN_POINT('Ctrl Pts',(0.394018705526142,5.1237767355219,14.6151725773312));
#10189=CARTESIAN_POINT('Ctrl Pts',(0.54197736105783,5.10807802432586,14.6071041081938));
#10190=CARTESIAN_POINT('Ctrl Pts',(0.651601628785827,5.09644666884379,14.6011260867141));
#10191=CARTESIAN_POINT('Ctrl Pts',(0.760840106234247,5.08128624006824,14.5951480652344));
#10192=CARTESIAN_POINT('Ctrl Pts',(0.869463065472354,5.06263118746363,14.5891700437547));
#10193=CARTESIAN_POINT('Ctrl Pts',(1.01606685763618,5.03745325570746,14.5811017621988));
#10194=CARTESIAN_POINT('Ctrl Pts',(1.16160336386802,5.00589835418219,14.573033480643));
#10195=CARTESIAN_POINT('Ctrl Pts',(1.30551321661218,4.96808170260423,14.5649651990871));
#10196=CARTESIAN_POINT('Ctrl Pts',(1.44939402607999,4.93027268302256,14.5568985458377));
#10197=CARTESIAN_POINT('Ctrl Pts',(1.59164851704583,4.88620451862095,14.5488318925882));
#10198=CARTESIAN_POINT('Ctrl Pts',(1.731730113762,4.83604294600346,14.5407652393387));
#10199=CARTESIAN_POINT('Ctrl Pts',(1.87181676032434,4.78587956509544,14.5326982952919));
#10200=CARTESIAN_POINT('Ctrl Pts',(2.00973004299052,4.72962244443411,14.5246313512451));
#10201=CARTESIAN_POINT('Ctrl Pts',(2.14494054464602,4.66748654228736,14.5165644071983));
#10202=CARTESIAN_POINT('Ctrl Pts',(2.28014286723538,4.60535439882539,14.5084979511318));
#10203=CARTESIAN_POINT('Ctrl Pts',(2.41264243545598,4.5373443242932,14.5004314950653));
#10204=CARTESIAN_POINT('Ctrl Pts',(2.54193174603147,4.46371857995297,14.4923650389989));
#10205=CARTESIAN_POINT('Ctrl Pts',(2.67125332214657,4.39007446151546,14.4842965698614));
#10206=CARTESIAN_POINT('Ctrl Pts',(2.79736275163924,4.31081203620864,14.476228100724));
#10207=CARTESIAN_POINT('Ctrl Pts',(2.91977838698316,4.22623884008063,14.4681596315866));
#10208=CARTESIAN_POINT('Ctrl Pts',(3.01047753759911,4.16357758743804,14.4621816101069));
#10209=CARTESIAN_POINT('Ctrl Pts',(3.09914950382448,4.09800193676208,14.4562035886272));
#10210=CARTESIAN_POINT('Ctrl Pts',(3.18560903719751,4.02965204758743,14.4502255671475));
#10211=CARTESIAN_POINT('Ctrl Pts',(3.30229979530371,3.93740310668865,14.4421572855916));
#10212=CARTESIAN_POINT('Ctrl Pts',(3.41500241293278,3.84006500296762,14.4340890040358));
#10213=CARTESIAN_POINT('Ctrl Pts',(3.52328081931377,3.73800653166306,14.4260207224799));
#10214=CARTESIAN_POINT('Ctrl Pts',(3.63153737340575,3.63596865736657,14.4179540692305));
#10215=CARTESIAN_POINT('Ctrl Pts',(3.73537125682889,3.52921254294249,14.409887415981));
#10216=CARTESIAN_POINT('Ctrl Pts',(3.83438180038918,3.41814522385229,14.4018207627315));
#10217=CARTESIAN_POINT('Ctrl Pts',(3.93339591321226,3.30707390086075,14.3937538186847));
#10218=CARTESIAN_POINT('Ctrl Pts',(4.02758611514645,3.19169130676403,14.3856868746379));
#10219=CARTESIAN_POINT('Ctrl Pts',(4.11659035352502,3.07243949065962,14.377619930591));
#10220=CARTESIAN_POINT('Ctrl Pts',(4.20558920791671,2.95319488825903,14.3695534745246));
#10221=CARTESIAN_POINT('Ctrl Pts',(4.28940252901126,2.83008179787626,14.3614870184581));
#10222=CARTESIAN_POINT('Ctrl Pts',(4.36771013839118,2.70357332238187,14.3534205623917));
#10223=CARTESIAN_POINT('Ctrl Pts',(4.44603729027829,2.57703327533508,14.3453520932542));
#10224=CARTESIAN_POINT('Ctrl Pts',(4.51885581004324,2.44709643124632,14.3372836241168));
#10225=CARTESIAN_POINT('Ctrl Pts',(4.58588988465929,2.31426327981058,14.3292151549793));
#10226=CARTESIAN_POINT('Ctrl Pts',(4.63555620067292,2.2158456718391,14.3232371334997));
#10227=CARTESIAN_POINT('Ctrl Pts',(4.68204805989948,2.11583871917326,14.31725911202));
#10228=CARTESIAN_POINT('Ctrl Pts',(4.72526984724929,2.01445412784126,14.3112810905403));
#10229=CARTESIAN_POINT('Ctrl Pts',(4.78360445693056,1.8776196532467,14.3032128089844));
#10230=CARTESIAN_POINT('Ctrl Pts',(4.83600217201594,1.73822429496611,14.2951445274286));
#10231=CARTESIAN_POINT('Ctrl Pts',(4.88225650980574,1.59680053073623,14.2870762458728));
#10232=CARTESIAN_POINT('Ctrl Pts',(4.92850151274114,1.45540530805098,14.2790095926233));
#10233=CARTESIAN_POINT('Ctrl Pts',(4.96860550904096,1.31198281053287,14.2709429393739));
#10234=CARTESIAN_POINT('Ctrl Pts',(5.00241139829535,1.16708215850673,14.2628762861245));
#10235=CARTESIAN_POINT('Ctrl Pts',(5.03621850622907,1.02217628291059,14.2548093420776));
#10236=CARTESIAN_POINT('Ctrl Pts',(5.06372697389811,0.875792467660107,14.2467423980308));
#10237=CARTESIAN_POINT('Ctrl Pts',(5.08483036262077,0.728492104191907,14.238675453984));
#10238=CARTESIAN_POINT('Ctrl Pts',(5.10593247477088,0.581200651122109,14.2306089979176));
#10239=CARTESIAN_POINT('Ctrl Pts',(5.1206302369751,0.432993088553311,14.2225425418511));
#10240=CARTESIAN_POINT('Ctrl Pts',(5.12886883845637,0.284438043185459,14.2144760857847));
#10241=CARTESIAN_POINT('Ctrl Pts',(5.13710949596936,0.13584592430631,14.2064076166473));
#10242=CARTESIAN_POINT('Ctrl Pts',(5.13888775276455,-0.0130935200164274,
14.1983391475099));
#10243=CARTESIAN_POINT('Ctrl Pts',(5.13420085913043,-0.161808839697807,
14.1902706783724));
#10244=CARTESIAN_POINT('Ctrl Pts',(5.1307282857908,-0.271993728589038,14.1842926568926));
#10245=CARTESIAN_POINT('Ctrl Pts',(5.12370775009287,-0.382055509579282,
14.1783146354129));
#10246=CARTESIAN_POINT('Ctrl Pts',(5.11315657628578,-0.491762533023262,
14.1723366139331));
#10247=CARTESIAN_POINT('Ctrl Pts',(5.09891610536943,-0.639829440576593,
14.1642683323772));
#10248=CARTESIAN_POINT('Ctrl Pts',(5.0782370906738,-0.7873047429416,14.1562000508214));
#10249=CARTESIAN_POINT('Ctrl Pts',(5.05119296727215,-0.933622070154904,
14.1481317692655));
#10250=CARTESIAN_POINT('Ctrl Pts',(5.02415430180085,-1.0799098682255,14.1400651160161));
#10251=CARTESIAN_POINT('Ctrl Pts',(4.99075315052114,-1.22503983207459,14.1319984627666));
#10252=CARTESIAN_POINT('Ctrl Pts',(4.951114274685,-1.36845460337946,14.1239318095172));
#10253=CARTESIAN_POINT('Ctrl Pts',(4.91147396989435,-1.51187454468931,14.1158648654703));
#10254=CARTESIAN_POINT('Ctrl Pts',(4.86559557510579,-1.65357884967861,14.1077979214235));
#10255=CARTESIAN_POINT('Ctrl Pts',(4.81365420981613,-1.79302362249343,14.0997309773767));
#10256=CARTESIAN_POINT('Ctrl Pts',(4.76171598652996,-1.93245996010518,14.0916645213102));
#10257=CARTESIAN_POINT('Ctrl Pts',(4.70371564279289,-2.06963672906724,14.0835980652438));
#10258=CARTESIAN_POINT('Ctrl Pts',(4.63987709547407,-2.20402838035157,14.0755316091773));
#10259=CARTESIAN_POINT('Ctrl Pts',(4.5760226165583,-2.33845357051968,14.0674631400399));
#10260=CARTESIAN_POINT('Ctrl Pts',(4.50632716422018,-2.47009195472382,14.0593946709024));
#10261=CARTESIAN_POINT('Ctrl Pts',(4.43106172229953,-2.59844041218419,14.051326201765));
#10262=CARTESIAN_POINT('Ctrl Pts',(4.37529669168255,-2.69353525886649,14.0453481802853));
#10263=CARTESIAN_POINT('Ctrl Pts',(4.316475001119,-2.78682455233121,14.0393701588056));
#10264=CARTESIAN_POINT('Ctrl Pts',(4.25472269144943,-2.87811316340504,14.0333921373259));
#10265=CARTESIAN_POINT('Ctrl Pts',(4.17137822324551,-3.00132152247264,14.02532385577));
#10266=CARTESIAN_POINT('Ctrl Pts',(4.08266294289405,-3.12092998993459,14.0172555742142));
#10267=CARTESIAN_POINT('Ctrl Pts',(3.98891230360449,-3.2364763550276,14.0091872926583));
#10268=CARTESIAN_POINT('Ctrl Pts',(3.89518058467149,-3.35199940104307,14.0011206394089));
#10269=CARTESIAN_POINT('Ctrl Pts',(3.7964157426101,-3.46346172331502,13.9930539861594));
#10270=CARTESIAN_POINT('Ctrl Pts',(3.6929939900547,-3.57043358038206,13.9849873329099));
#10271=CARTESIAN_POINT('Ctrl Pts',(3.5895685092155,-3.67740929371177,13.9769203888631));
#10272=CARTESIAN_POINT('Ctrl Pts',(3.48148600929417,-3.7798939773071,13.9688534448163));
#10273=CARTESIAN_POINT('Ctrl Pts',(3.36916048297568,-3.87749380430906,13.9607865007695));
#10274=CARTESIAN_POINT('Ctrl Pts',(3.25684175138037,-3.97508772736532,13.952720044703));
#10275=CARTESIAN_POINT('Ctrl Pts',(3.14028075728999,-4.06779716848725,13.9446535886365));
#10276=CARTESIAN_POINT('Ctrl Pts',(3.01992556597796,-4.15526775773267,13.9365871325701));
#10277=CARTESIAN_POINT('Ctrl Pts',(2.89954033873187,-4.24276017620558,13.9285186634326));
#10278=CARTESIAN_POINT('Ctrl Pts',(2.7753592897203,-4.325010935101,13.9204501942952));
#10279=CARTESIAN_POINT('Ctrl Pts',(2.64786108462242,-4.40170787752234,13.9123817251578));
#10280=CARTESIAN_POINT('Ctrl Pts',(2.55339619968378,-4.45853352330625,13.9064037036781));
#10281=CARTESIAN_POINT('Ctrl Pts',(2.45711101131606,-4.51231127016196,13.9004256821984));
#10282=CARTESIAN_POINT('Ctrl Pts',(2.3592095547749,-4.56293007169284,13.8944476607187));
#10283=CARTESIAN_POINT('Ctrl Pts',(2.22707611919215,-4.63124811707906,13.8863793791628));
#10284=CARTESIAN_POINT('Ctrl Pts',(2.09194872668348,-4.69383545006435,13.878311097607));
#10285=CARTESIAN_POINT('Ctrl Pts',(1.95434308261613,-4.75044668193745,13.8702428160512));
#10286=CARTESIAN_POINT('Ctrl Pts',(1.81676520953644,-4.80704648877175,13.8621761628017));
#10287=CARTESIAN_POINT('Ctrl Pts',(1.67671038864624,-4.85767247477758,13.8541095095522));
#10288=CARTESIAN_POINT('Ctrl Pts',(1.53471458296422,-4.90212726388626,13.8460428563028));
#10289=CARTESIAN_POINT('Ctrl Pts',(1.3927136584301,-4.94658365555981,13.8379759122559));
#10290=CARTESIAN_POINT('Ctrl Pts',(1.24877192383751,-4.98486830265642,13.8299089682091));
#10291=CARTESIAN_POINT('Ctrl Pts',(1.10344133525766,-5.0168334417384,13.8218420241623));
#10292=CARTESIAN_POINT('Ctrl Pts',(0.958119537921845,-5.04879664720586,
13.8137755680959));
#10293=CARTESIAN_POINT('Ctrl Pts',(0.811409378153299,-5.07444103912968,
13.8057091120294));
#10294=CARTESIAN_POINT('Ctrl Pts',(0.663873854709686,-5.0936698035437,13.7976426559629));
#10295=CARTESIAN_POINT('Ctrl Pts',(0.516301512187403,-5.11290336670295,
13.7895741868255));
#10296=CARTESIAN_POINT('Ctrl Pts',(0.367903722721964,-5.12571805960758,
13.7815057176881));
#10297=CARTESIAN_POINT('Ctrl Pts',(0.21925016013056,-5.13206877679779,13.7734372485507));
#10298=CARTESIAN_POINT('Ctrl Pts',(0.10911102777809,-5.13677409612517,13.7674592270709));
#10299=CARTESIAN_POINT('Ctrl Pts',(-0.00116835654856688,-5.13793208944069,
13.7614812055912));
#10300=CARTESIAN_POINT('Ctrl Pts',(-0.111355696321223,-5.13554286043811,
13.7555031841115));
#10301=CARTESIAN_POINT('Ctrl Pts',(-0.26007086641402,-5.13231821958333,
13.7474349025556));
#10302=CARTESIAN_POINT('Ctrl Pts',(-0.408673367827961,-5.12262889401346,
13.7393666209998));
#10303=CARTESIAN_POINT('Ctrl Pts',(-0.5565929450814,-5.10650613002527,13.7312983394439));
#10304=CARTESIAN_POINT('Ctrl Pts',(-0.704482669832755,-5.09038661986495,
13.7232316861944));
#10305=CARTESIAN_POINT('Ctrl Pts',(-0.851689416522729,-5.06783629741423,
13.715165032945));
#10306=CARTESIAN_POINT('Ctrl Pts',(-0.997648111549489,-5.03893826197759,
13.7070983796955));
#10307=CARTESIAN_POINT('Ctrl Pts',(-1.14361206828793,-5.01003918478643,
13.6990314356487));
#10308=CARTESIAN_POINT('Ctrl Pts',(-1.28832755789921,-4.97479199727496,
13.6909644916018));
#10309=CARTESIAN_POINT('Ctrl Pts',(-1.43123919899822,-4.93333101643818,
13.682897547555));
#10310=CARTESIAN_POINT('Ctrl Pts',(-1.57414219517855,-4.89187254363226,
13.6748310914886));
#10311=CARTESIAN_POINT('Ctrl Pts',(-1.71524124345498,-4.8442011225082,13.6667646354221));
#10312=CARTESIAN_POINT('Ctrl Pts',(-1.8539956412884,-4.79050109326609,13.6586981793556));
#10313=CARTESIAN_POINT('Ctrl Pts',(-1.99278466677606,-4.73678766260338,
13.6506297102182));
#10314=CARTESIAN_POINT('Ctrl Pts',(-2.12922756351663,-4.67704273644587,
13.6425612410808));
#10315=CARTESIAN_POINT('Ctrl Pts',(-2.26280250628869,-4.61149925512665,
13.6344927719433));
#10316=CARTESIAN_POINT('Ctrl Pts',(-2.36176971598311,-4.56293733681169,
13.6285147504636));
#10317=CARTESIAN_POINT('Ctrl Pts',(-2.45916294008812,-4.51119331827604,
13.622536728984));
#10318=CARTESIAN_POINT('Ctrl Pts',(-2.5547782425683,-4.45637842802871,13.6165587075043));
#10319=CARTESIAN_POINT('Ctrl Pts',(-2.68382615316517,-4.38239710001397,
13.6084904259485));
#10320=CARTESIAN_POINT('Ctrl Pts',(-2.80968223221986,-4.30279286758047,
13.6004221443926));
#10321=CARTESIAN_POINT('Ctrl Pts',(-2.93186067264955,-4.21786599581719,
13.5923538628368));
#10322=CARTESIAN_POINT('Ctrl Pts',(-3.05401445554449,-4.13295626363504,
13.5842872095874));
#10323=CARTESIAN_POINT('Ctrl Pts',(-3.17249180889903,-4.04272622398234,
13.5762205563379));
#10324=CARTESIAN_POINT('Ctrl Pts',(-3.28683628396969,-3.94751919626496,
13.5681539030885));
#10325=CARTESIAN_POINT('Ctrl Pts',(-3.40118488108078,-3.85230873639908,
13.5600869590417));
#10326=CARTESIAN_POINT('Ctrl Pts',(-3.51140004498186,-3.75212113832894,
13.5520200149948));
#10327=CARTESIAN_POINT('Ctrl Pts',(-3.61705834195898,-3.64734006001153,
13.543953070948));
#10328=CARTESIAN_POINT('Ctrl Pts',(-3.72271024752267,-3.54256532004342,
13.5358866148816));
#10329=CARTESIAN_POINT('Ctrl Pts',(-3.82380560316017,-3.43319788940275,
13.5278201588152));
#10330=CARTESIAN_POINT('Ctrl Pts',(-3.91995779759971,-3.31965832993958,
13.5197537027487));
#10331=CARTESIAN_POINT('Ctrl Pts',(-4.01613398785483,-3.20609043545664,
13.5116852336113));
#10332=CARTESIAN_POINT('Ctrl Pts',(-4.10736433736911,-3.08834858393419,
13.5036167644739));
#10333=CARTESIAN_POINT('Ctrl Pts',(-4.19330206326122,-2.96688698280693,
13.4955482953365));
#10334=CARTESIAN_POINT('Ctrl Pts',(-4.25697431168338,-2.87689468710158,
13.4895702738567));
#10335=CARTESIAN_POINT('Ctrl Pts',(-4.31774199246088,-2.78486114686199,
13.4835922523769));
#10336=CARTESIAN_POINT('Ctrl Pts',(-4.37547923900897,-2.69098160370923,
13.4776142308972));
#10337=CARTESIAN_POINT('Ctrl Pts',(-4.45340474713679,-2.56427637371713,
13.4695459493413));
#10338=CARTESIAN_POINT('Ctrl Pts',(-4.5258372627426,-2.4341605901263,13.4614776677855));
#10339=CARTESIAN_POINT('Ctrl Pts',(-4.59249384154503,-2.30113034786624,
13.4534093862297));
#10340=CARTESIAN_POINT('Ctrl Pts',(-4.65913696799926,-2.1681269532058,13.4453427329802));
#10341=CARTESIAN_POINT('Ctrl Pts',(-4.72000633500855,-2.03221056908114,
13.4372760797307));
#10342=CARTESIAN_POINT('Ctrl Pts',(-4.77486537706007,-1.89390105165317,
13.4292094264813));
#10343=CARTESIAN_POINT('Ctrl Pts',(-4.82972639674276,-1.75558654826113,
13.4211424824344));
#10344=CARTESIAN_POINT('Ctrl Pts',(-4.87857653234138,-1.61487904521717,
13.4130755383876));
#10345=CARTESIAN_POINT('Ctrl Pts',(-4.92122750884501,-1.47231802566128,
13.4050085943408));
#10346=CARTESIAN_POINT('Ctrl Pts',(-4.96387590533327,-1.32976562981468,
13.3969421382743));
#10347=CARTESIAN_POINT('Ctrl Pts',(-5.00032579884621,-1.18536025914133,
13.3888756822079));
#10348=CARTESIAN_POINT('Ctrl Pts',(-5.03043890502238,-1.03965618611985,
13.3808092261414));
#10349=CARTESIAN_POINT('Ctrl Pts',(-5.06055952624849,-0.893915751077784,
13.372740757004));
#10350=CARTESIAN_POINT('Ctrl Pts',(-5.08434013248878,-0.746876290254184,
13.3646722878666));
#10351=CARTESIAN_POINT('Ctrl Pts',(-5.10169351076287,-0.599102566127044,
13.3566038187291));
#10352=CARTESIAN_POINT('Ctrl Pts',(-5.11455082809301,-0.489615316200809,
13.3506257972494));
#10353=CARTESIAN_POINT('Ctrl Pts',(-5.12388097766677,-0.379725226270334,
13.3446477757697));
#10354=CARTESIAN_POINT('Ctrl Pts',(-5.12966684205185,-0.269663961355155,
13.3386697542899));
#10355=CARTESIAN_POINT('Ctrl Pts',(-5.13438618858459,-0.179890469548952,
13.3337936712943));
#10356=CARTESIAN_POINT('Ctrl Pts',(-5.13674848218115,-0.0899925721050492,
13.3289175882987));
#10357=CARTESIAN_POINT('Ctrl Pts',(-5.13674999926869,-8.66784045078238E-5,
13.3240415053031));
#10358=CARTESIAN_POINT('Ctrl Pts',(-5.13674999942792,-7.66631357963787E-5,
13.3242245870723));
#10359=CARTESIAN_POINT('Ctrl Pts',(-5.13675482000189,0.322921907747067,
13.3065553374322));
#10360=CARTESIAN_POINT('Ctrl Pts',(-5.10629412606806,0.645211665566582,
13.2888158745499));
#10361=CARTESIAN_POINT('Ctrl Pts',(-5.0354960278084,1.01635935148288,13.2683148233289));
#10362=CARTESIAN_POINT('Ctrl Pts',(-5.02436109757278,1.0700477581446,13.2653458440043));
#10363=CARTESIAN_POINT('Ctrl Pts',(-4.93693907417981,1.46005464630582,13.2437409801159));
#10364=CARTESIAN_POINT('Ctrl Pts',(-4.8278152561397,1.78810590632312,13.2254297836528));
#10365=CARTESIAN_POINT('Ctrl Pts',(-4.65003687406371,2.18434367576704,13.201989082554));
#10366=CARTESIAN_POINT('Ctrl Pts',(-4.61130000993693,2.26497503841401,13.1971366758318));
#10367=CARTESIAN_POINT('Ctrl Pts',(-4.48624034085036,2.50876666159917,13.1821954669199));
#10368=CARTESIAN_POINT('Ctrl Pts',(-4.3932231057094,2.66830254988752,13.1720601586962));
#10369=CARTESIAN_POINT('Ctrl Pts',(-4.29183623954907,2.82247094854728,13.1619495546845));
#10370=CARTESIAN_POINT('Origin',(0.,0.,0.));
#10371=CARTESIAN_POINT('',(-4.29183622844418,2.82247096543331,11.4121712634621));
#10372=CARTESIAN_POINT('',(-4.29155726418515,2.82228712074135,11.8889308194183));
#10373=CARTESIAN_POINT('',(-4.29183622825304,2.82247096572397,0.));
#10374=CARTESIAN_POINT('',(-5.13674999832603,-0.000131139391237522,12.0509584946969));
#10375=CARTESIAN_POINT('Ctrl Pts',(-4.29155726418515,2.82228712074135,11.8889308194183));
#10376=CARTESIAN_POINT('Ctrl Pts',(-4.46838982832423,2.55377308187227,11.9063606652066));
#10377=CARTESIAN_POINT('Ctrl Pts',(-4.9388247281808,1.67089962616198,11.9603698894268));
#10378=CARTESIAN_POINT('Ctrl Pts',(-5.13610861091696,0.674465849271032,
12.014379113647));
#10379=CARTESIAN_POINT('Ctrl Pts',(-5.13680565136043,-0.00013109253210184,
12.050958492079));
#10380=CARTESIAN_POINT('Ctrl Pts',(-5.13674999832603,-0.000131139391237522,
12.0509584946969));
#10381=CARTESIAN_POINT('Ctrl Pts',(-5.13674597131034,-0.157869959281706,
12.0595118252836));
#10382=CARTESIAN_POINT('Ctrl Pts',(-5.12947186524448,-0.315573404970336,
12.0680651558703));
#10383=CARTESIAN_POINT('Ctrl Pts',(-5.11496338830488,-0.472599300465667,
12.076618486457));
#10384=CARTESIAN_POINT('Ctrl Pts',(-5.11295823985499,-0.494301111913994,
12.0778006021015));
#10385=CARTESIAN_POINT('Ctrl Pts',(-5.11081499098403,-0.515989987668825,
12.0789827177459));
#10386=CARTESIAN_POINT('Ctrl Pts',(-5.10853381397671,-0.537664239053161,
12.0801648333904));
#10387=CARTESIAN_POINT('Ctrl Pts',(-5.09296412038498,-0.685597280548789,
12.0882331149463));
#10388=CARTESIAN_POINT('Ctrl Pts',(-5.07096145592205,-0.832880915801725,
12.0963013965022));
#10389=CARTESIAN_POINT('Ctrl Pts',(-5.04260433929914,-0.978949457214977,
12.1043696780582));
#10390=CARTESIAN_POINT('Ctrl Pts',(-5.0142529455893,-1.12498851969439,12.1124363313077));
#10391=CARTESIAN_POINT('Ctrl Pts',(-4.97954972124561,-1.26981265281502,
12.1205029845572));
#10392=CARTESIAN_POINT('Ctrl Pts',(-4.93862442815397,-1.41286564122031,
12.1285696378067));
#10393=CARTESIAN_POINT('Ctrl Pts',(-4.89769765973334,-1.55592378658856,
12.1366365818536));
#10394=CARTESIAN_POINT('Ctrl Pts',(-4.85054846112362,-1.697210340201,12.1447035259005));
#10395=CARTESIAN_POINT('Ctrl Pts',(-4.79735682951735,-1.83618300089704,
12.1527704699474));
#10396=CARTESIAN_POINT('Ctrl Pts',(-4.7441684155448,-1.97514725494891,12.1608369260139));
#10397=CARTESIAN_POINT('Ctrl Pts',(-4.68493841891923,-2.11179758724498,
12.1689033820804));
#10398=CARTESIAN_POINT('Ctrl Pts',(-4.61989546746367,-2.24561048096251,
12.1769698381469));
#10399=CARTESIAN_POINT('Ctrl Pts',(-4.55483628383924,-2.37945676912844,
12.1850383072844));
#10400=CARTESIAN_POINT('Ctrl Pts',(-4.48396139081855,-2.5104639056216,12.1931067764219));
#10401=CARTESIAN_POINT('Ctrl Pts',(-4.40754627986778,-2.638131223674,12.2011752455594));
#10402=CARTESIAN_POINT('Ctrl Pts',(-4.35092944626179,-2.73272140633764,
12.2071532670387));
#10403=CARTESIAN_POINT('Ctrl Pts',(-4.29127229175841,-2.82547865657246,
12.2131312885181));
#10404=CARTESIAN_POINT('Ctrl Pts',(-4.22870260458065,-2.91620898505453,
12.2191093099975));
#10405=CARTESIAN_POINT('Ctrl Pts',(-4.14425495668391,-3.03866385383857,
12.2271775915533));
#10406=CARTESIAN_POINT('Ctrl Pts',(-4.05446904407064,-3.15747074064452,
12.2352458731091));
#10407=CARTESIAN_POINT('Ctrl Pts',(-3.95968445756145,-3.2721704660739,12.2433141546649));
#10408=CARTESIAN_POINT('Ctrl Pts',(-3.86491900007579,-3.38684704329083,
12.2513808079144));
#10409=CARTESIAN_POINT('Ctrl Pts',(-3.76515709203226,-3.49741785778094,
12.2594474611638));
#10410=CARTESIAN_POINT('Ctrl Pts',(-3.66077879042398,-3.60345656420081,
12.2675141144133));
#10411=CARTESIAN_POINT('Ctrl Pts',(-3.55639672604888,-3.70949909324397,
12.2755810584601));
#10412=CARTESIAN_POINT('Ctrl Pts',(-3.44739816459536,-3.81100894873496,
12.2836480025069));
#10413=CARTESIAN_POINT('Ctrl Pts',(-3.33420061903242,-3.90759603778894,
12.2917149465537));
#10414=CARTESIAN_POINT('Ctrl Pts',(-3.22100992094223,-4.00417728415917,
12.2997814026201));
#10415=CARTESIAN_POINT('Ctrl Pts',(-3.10362099924908,-4.09583614559698,
12.3078478586866));
#10416=CARTESIAN_POINT('Ctrl Pts',(-2.98248508377152,-4.18222229055085,
12.315914314753));
#10417=CARTESIAN_POINT('Ctrl Pts',(-2.86131893752182,-4.26862999409742,
12.3239827838904));
#10418=CARTESIAN_POINT('Ctrl Pts',(-2.73640419822553,-4.3497621589822,12.3320512530278));
#10419=CARTESIAN_POINT('Ctrl Pts',(-2.60822231575517,-4.4253109398207,12.3401197221653));
#10420=CARTESIAN_POINT('Ctrl Pts',(-2.51325088639444,-4.48128589949841,
12.3460977436451));
#10421=CARTESIAN_POINT('Ctrl Pts',(-2.41648660036535,-4.53419673492632,
12.3520757651249));
#10422=CARTESIAN_POINT('Ctrl Pts',(-2.31813448200849,-4.58393423663814,
12.3580537866048));
#10423=CARTESIAN_POINT('Ctrl Pts',(-2.18539280732642,-4.65106282910802,
12.3661220681606));
#10424=CARTESIAN_POINT('Ctrl Pts',(-2.04970876430788,-4.71243405140835,
12.3741903497165));
#10425=CARTESIAN_POINT('Ctrl Pts',(-1.9116002413709,-4.76780715630265,12.3822586312723));
#10426=CARTESIAN_POINT('Ctrl Pts',(-1.77351959091066,-4.8231690860316,12.3903252845218));
#10427=CARTESIAN_POINT('Ctrl Pts',(-1.63301574374822,-4.87253519025532,
12.3983919377713));
#10428=CARTESIAN_POINT('Ctrl Pts',(-1.49062641393189,-4.9157129143786,12.4064585910207));
#10429=CARTESIAN_POINT('Ctrl Pts',(-1.348231951077,-4.95889219502949,12.4145255350676));
#10430=CARTESIAN_POINT('Ctrl Pts',(-1.20395218521327,-4.99588254949151,
12.4225924791144));
#10431=CARTESIAN_POINT('Ctrl Pts',(-1.05834037722278,-5.02654117743404,
12.4306594231612));
#10432=CARTESIAN_POINT('Ctrl Pts',(-0.912737377487716,-5.05719795079465,
12.4387258792277));
#10433=CARTESIAN_POINT('Ctrl Pts',(-0.765802820923515,-5.08152369649344,
12.4467923352941));
#10434=CARTESIAN_POINT('Ctrl Pts',(-0.61810055307335,-5.09942666079143,
12.4548587913606));
#10435=CARTESIAN_POINT('Ctrl Pts',(-0.470361424531666,-5.11733409296695,
12.462927260498));
#10436=CARTESIAN_POINT('Ctrl Pts',(-0.321854530562556,-5.12881550037983,
12.4709957296355));
#10437=CARTESIAN_POINT('Ctrl Pts',(-0.173149927102597,-5.13383089566109,
12.4790641987729));
#10438=CARTESIAN_POINT('Ctrl Pts',(-0.062972977985472,-5.13754685964505,
12.4850422202526));
#10439=CARTESIAN_POINT('Ctrl Pts',(0.0473123587203552,-5.13771438107194,
12.4910202417323));
#10440=CARTESIAN_POINT('Ctrl Pts',(0.157473796786609,-5.13433564989918,
12.4969982632119));
#10441=CARTESIAN_POINT('Ctrl Pts',(0.306154008448005,-5.12977552001405,
12.5050665447678));
#10442=CARTESIAN_POINT('Ctrl Pts',(0.454663496287294,-5.11875197802132,
12.5131348263236));
#10443=CARTESIAN_POINT('Ctrl Pts',(0.602432308446221,-5.10130139045324,
12.5212031078794));
#10444=CARTESIAN_POINT('Ctrl Pts',(0.750171298529824,-5.08385432468878,
12.5292697611289));
#10445=CARTESIAN_POINT('Ctrl Pts',(0.897169582619754,-5.05998283985507,
12.5373364143783));
#10446=CARTESIAN_POINT('Ctrl Pts',(1.04286285622328,-5.02977510686212,12.5454030676277));
#10447=CARTESIAN_POINT('Ctrl Pts',(1.18856138197026,-4.99956628490093,12.5534700116746));
#10448=CARTESIAN_POINT('Ctrl Pts',(1.33295447821516,-4.96302082119344,12.5615369557214));
#10449=CARTESIAN_POINT('Ctrl Pts',(1.47548799227996,-4.92027801522817,12.5696038997682));
#10450=CARTESIAN_POINT('Ctrl Pts',(1.61801288429949,-4.87753779483311,12.5776703558346));
#10451=CARTESIAN_POINT('Ctrl Pts',(1.75867810234035,-4.82860107804601,12.5857368119011));
#10452=CARTESIAN_POINT('Ctrl Pts',(1.89694462123966,-4.77365705371154,12.5938032679675));
#10453=CARTESIAN_POINT('Ctrl Pts',(2.03524564603772,-4.71869931750411,12.6018717371049));
#10454=CARTESIAN_POINT('Ctrl Pts',(2.17114646751808,-4.65773139976573,12.6099402062423));
#10455=CARTESIAN_POINT('Ctrl Pts',(2.30412737355467,-4.59099091797578,12.6180086753798));
#10456=CARTESIAN_POINT('Ctrl Pts',(2.40265445460921,-4.54154212825909,12.6239866968596));
#10457=CARTESIAN_POINT('Ctrl Pts',(2.49957903493763,-4.48892550270796,12.6299647183393));
#10458=CARTESIAN_POINT('Ctrl Pts',(2.5946981856787,-4.43325409690621,12.6359427398191));
#10459=CARTESIAN_POINT('Ctrl Pts',(2.72307646135506,-4.35811676624644,12.644011021375));
#10460=CARTESIAN_POINT('Ctrl Pts',(2.84821253460503,-4.27738542395611,12.6520793029308));
#10461=CARTESIAN_POINT('Ctrl Pts',(2.96962331463579,-4.1913646860744,12.6601475844867));
#10462=CARTESIAN_POINT('Ctrl Pts',(3.09100959205767,-4.10536130853331,12.6682142377361));
#10463=CARTESIAN_POINT('Ctrl Pts',(3.20867180623876,-4.01407085630716,12.6762808909856));
#10464=CARTESIAN_POINT('Ctrl Pts',(3.32215661021474,-3.91784073434673,12.684347544235));
#10465=CARTESIAN_POINT('Ctrl Pts',(3.43564550524069,-3.82160714335588,12.6924144882819));
#10466=CARTESIAN_POINT('Ctrl Pts',(3.54495643380937,-3.72043373748103,12.7004814323287));
#10467=CARTESIAN_POINT('Ctrl Pts',(3.64966942493724,-3.61470796208743,12.7085483763755));
#10468=CARTESIAN_POINT('Ctrl Pts',(3.75437608183454,-3.5089885821891,12.716614832442));
#10469=CARTESIAN_POINT('Ctrl Pts',(3.85448512536721,-3.39871761946791,12.7246812885084));
#10470=CARTESIAN_POINT('Ctrl Pts',(3.94961373694471,-3.28431909098944,12.7327477445749));
#10471=CARTESIAN_POINT('Ctrl Pts',(4.04476608889159,-3.1698920131263,12.7408162137123));
#10472=CARTESIAN_POINT('Ctrl Pts',(4.13493531302918,-3.05133556542775,12.7488846828497));
#10473=CARTESIAN_POINT('Ctrl Pts',(4.21977871972388,-2.92910705148608,12.7569531519872));
#10474=CARTESIAN_POINT('Ctrl Pts',(4.2826401744799,-2.8385465412665,12.7629311734669));
#10475=CARTESIAN_POINT('Ctrl Pts',(4.34257884620506,-2.74597095491807,12.7689091949466));
#10476=CARTESIAN_POINT('Ctrl Pts',(4.39947062686654,-2.65157665660236,12.7748872164263));
#10477=CARTESIAN_POINT('Ctrl Pts',(4.47625504561576,-2.52417668344032,12.7829554979822));
#10478=CARTESIAN_POINT('Ctrl Pts',(4.54751606300949,-2.39341562709532,12.791023779538));
#10479=CARTESIAN_POINT('Ctrl Pts',(4.61297520163336,-2.25979210362715,12.7990920610938));
#10480=CARTESIAN_POINT('Ctrl Pts',(4.67842112957137,-2.12619554749205,12.8071587143433));
#10481=CARTESIAN_POINT('Ctrl Pts',(4.73806736920513,-1.98973797382458,12.8152253675928));
#10482=CARTESIAN_POINT('Ctrl Pts',(4.79168203341927,-1.8509413424274,12.8232920208422));
#10483=CARTESIAN_POINT('Ctrl Pts',(4.84529863040559,-1.71213970750606,12.831358964889));
#10484=CARTESIAN_POINT('Ctrl Pts',(4.89288309406887,-1.57099915352256,12.8394259089359));
#10485=CARTESIAN_POINT('Ctrl Pts',(4.93425200211901,-1.42806083276747,12.8474928529827));
#10486=CARTESIAN_POINT('Ctrl Pts',(4.9756184077079,-1.28513115854491,12.8555593090491));
#10487=CARTESIAN_POINT('Ctrl Pts',(5.01076991864176,-1.14040425332142,12.8636257651156));
#10488=CARTESIAN_POINT('Ctrl Pts',(5.03957323408765,-0.994435609160971,
12.871692221182));
#10489=CARTESIAN_POINT('Ctrl Pts',(5.06838373771108,-0.848430536953496,
12.8797606903195));
#10490=CARTESIAN_POINT('Ctrl Pts',(5.09084281542292,-0.701183431376395,
12.8878291594569));
#10491=CARTESIAN_POINT('Ctrl Pts',(5.10686832992285,-0.553259815395071,
12.8958976285944));
#10492=CARTESIAN_POINT('Ctrl Pts',(5.11874181772727,-0.443661508872842,
12.901875650074));
#10493=CARTESIAN_POINT('Ctrl Pts',(5.12708466209961,-0.333692056279775,
12.9078536715537));
#10494=CARTESIAN_POINT('Ctrl Pts',(5.13188182689416,-0.223583267024828,
12.9138316930334));
#10495=CARTESIAN_POINT('Ctrl Pts',(5.13835635636243,-0.074974113227048,
12.9218999745893));
#10496=CARTESIAN_POINT('Ctrl Pts',(5.13837260241816,0.0739439387092463,
12.9299682561451));
#10497=CARTESIAN_POINT('Ctrl Pts',(5.13192457927966,0.222599809266103,12.938036537701));
#10498=CARTESIAN_POINT('Ctrl Pts',(5.12547785745385,0.371225678725344,12.9461031909504));
#10499=CARTESIAN_POINT('Ctrl Pts',(5.11256948346549,0.51958914186445,12.9541698441999));
#10500=CARTESIAN_POINT('Ctrl Pts',(5.09324555201993,0.667120910577073,12.9622364974493));
#10501=CARTESIAN_POINT('Ctrl Pts',(5.07392092395979,0.814657997709612,12.9703034414962));
#10502=CARTESIAN_POINT('Ctrl Pts',(5.04818031487552,0.961363001730773,12.978370385543));
#10503=CARTESIAN_POINT('Ctrl Pts',(5.01612155994829,1.1066729680994,12.9864373295898));
#10504=CARTESIAN_POINT('Ctrl Pts',(4.98406474429854,1.25197414447146,12.9945037856563));
#10505=CARTESIAN_POINT('Ctrl Pts',(4.94569061953874,1.39588012893846,13.0025702417228));
#10506=CARTESIAN_POINT('Ctrl Pts',(4.90114789437699,1.53783935440083,13.0106366977892));
#10507=CARTESIAN_POINT('Ctrl Pts',(4.85659405309853,1.67983400731659,13.0187051669267));
#10508=CARTESIAN_POINT('Ctrl Pts',(4.80586863383362,1.81988061424758,13.0267736360641));
#10509=CARTESIAN_POINT('Ctrl Pts',(4.74917007240058,1.95744327782818,13.0348421052015));
#10510=CARTESIAN_POINT('Ctrl Pts',(4.70716145684518,2.05936503568366,13.0408201266812));
#10511=CARTESIAN_POINT('Ctrl Pts',(4.66187492398926,2.15992354351756,13.0467981481609));
#10512=CARTESIAN_POINT('Ctrl Pts',(4.61340817460148,2.25890804970459,13.0527761696406));
#10513=CARTESIAN_POINT('Ctrl Pts',(4.54799466254168,2.39250323137016,13.0608444511965));
#10514=CARTESIAN_POINT('Ctrl Pts',(4.47676217731939,2.52327983289129,13.0689127327523));
#10515=CARTESIAN_POINT('Ctrl Pts',(4.39997868380664,2.65073351066214,13.0769810143081));
#10516=CARTESIAN_POINT('Ctrl Pts',(4.3232106864131,2.77816146627195,13.0850476675576));
#10517=CARTESIAN_POINT('Ctrl Pts',(4.24089408643114,2.90226755266968,13.093114320807));
#10518=CARTESIAN_POINT('Ctrl Pts',(4.15334172490436,3.02257391616292,13.1011809740565));
#10519=CARTESIAN_POINT('Ctrl Pts',(4.06578620717445,3.1428846166188,13.1092479181033));
#10520=CARTESIAN_POINT('Ctrl Pts',(3.97299474191275,3.25939505020903,13.1173148621501));
#10521=CARTESIAN_POINT('Ctrl Pts',(3.8753225746625,3.37165767906696,13.1253818061969));
#10522=CARTESIAN_POINT('Ctrl Pts',(3.77765631573385,3.48391351700653,13.1334482622634));
#10523=CARTESIAN_POINT('Ctrl Pts',(3.67511016337259,3.59192181507812,13.1415147183298));
#10524=CARTESIAN_POINT('Ctrl Pts',(3.56807858840896,3.69526937440798,13.1495811743962));
#10525=CARTESIAN_POINT('Ctrl Pts',(3.46102030256325,3.79864272523414,13.1576496435337));
#10526=CARTESIAN_POINT('Ctrl Pts',(3.34947459514941,3.89735278262419,13.1657181126711));
#10527=CARTESIAN_POINT('Ctrl Pts',(3.23387210681231,3.99102389861065,13.1737865818085));
#10528=CARTESIAN_POINT('Ctrl Pts',(3.14822089508619,4.06042590460018,13.1797646032883));
#10529=CARTESIAN_POINT('Ctrl Pts',(3.06034347728788,4.12706255365521,13.1857426247681));
#10530=CARTESIAN_POINT('Ctrl Pts',(2.97042647675405,4.19079552217697,13.1917206462478));
#10531=CARTESIAN_POINT('Ctrl Pts',(2.84906932214722,4.27681320146484,13.1997889278037));
#10532=CARTESIAN_POINT('Ctrl Pts',(2.72395086647462,4.35757184500561,13.2078572093595));
#10533=CARTESIAN_POINT('Ctrl Pts',(2.59554770941672,4.43275677774471,13.2159254909154));
#10534=CARTESIAN_POINT('Ctrl Pts',(2.46717046613967,4.50792653697939,13.2239921441648));
#10535=CARTESIAN_POINT('Ctrl Pts',(2.33551012946518,4.57752466238813,13.2320587974143));
#10536=CARTESIAN_POINT('Ctrl Pts',(2.20107003246214,4.6412812104738,13.2401254506638));
#10537=CARTESIAN_POINT('Ctrl Pts',(2.06662508898502,4.70504005693967,13.2481923947106));
#10538=CARTESIAN_POINT('Ctrl Pts',(1.92940048210627,4.76295675943438,13.2562593387574));
#10539=CARTESIAN_POINT('Ctrl Pts',(1.78992227741529,4.81480828313158,13.2643262828042));
#10540=CARTESIAN_POINT('Ctrl Pts',(1.65045250994969,4.86665667025993,13.2723927388707));
#10541=CARTESIAN_POINT('Ctrl Pts',(1.50872972796709,4.91244049801187,13.2804591949372));
#10542=CARTESIAN_POINT('Ctrl Pts',(1.36529801302686,4.9519856520516,13.2885256510036));
#10543=CARTESIAN_POINT('Ctrl Pts',(1.22183050315766,4.99154067501036,13.2965941201411));
#10544=CARTESIAN_POINT('Ctrl Pts',(1.07665352722731,5.02485382454942,13.3046625892785));
#10545=CARTESIAN_POINT('Ctrl Pts',(0.93032496300189,5.05180126546121,13.3127310584159));
#10546=CARTESIAN_POINT('Ctrl Pts',(0.82190844865043,5.07176693402233,13.3187090798956));
#10547=CARTESIAN_POINT('Ctrl Pts',(0.712860072264733,5.08823918837666,13.3246871013753));
#10548=CARTESIAN_POINT('Ctrl Pts',(0.603409890723613,5.10118584902343,13.330665122855));
#10549=CARTESIAN_POINT('Ctrl Pts',(0.455689631769934,5.11865940673158,13.3387334044109));
#10550=CARTESIAN_POINT('Ctrl Pts',(0.307182552668397,5.12971535142931,13.3468016859667));
#10551=CARTESIAN_POINT('Ctrl Pts',(0.158457717789245,5.13430537796234,13.3548699675226));
#10552=CARTESIAN_POINT('Ctrl Pts',(0.00976289792575968,5.13889447815568,
13.362936620772));
#10553=CARTESIAN_POINT('Ctrl Pts',(-0.139149259385165,5.13702025333934,
13.3710032740215));
#10554=CARTESIAN_POINT('Ctrl Pts',(-0.287707615372341,5.12868646834224,
13.379069927271));
#10555=CARTESIAN_POINT('Ctrl Pts',(-0.436271326787243,5.12035238291785,
13.3871368713178));
#10556=CARTESIAN_POINT('Ctrl Pts',(-0.584480880663312,5.10555828609689,
13.3952038153646));
#10557=CARTESIAN_POINT('Ctrl Pts',(-0.731767618689695,5.08436001033928,
13.4032707594114));
#10558=CARTESIAN_POINT('Ctrl Pts',(-0.879045447141863,5.06316301689407,
13.4113372154779));
#10559=CARTESIAN_POINT('Ctrl Pts',(-1.02540024388673,5.03556266750755,13.4194036715444));
#10560=CARTESIAN_POINT('Ctrl Pts',(-1.1702709353133,5.00166637236641,13.4274701276108));
#10561=CARTESIAN_POINT('Ctrl Pts',(-1.31517778078097,4.9677616180398,13.4355385967483));
#10562=CARTESIAN_POINT('Ctrl Pts',(-1.4585994582288,4.92755785315958,13.4436070658857));
#10563=CARTESIAN_POINT('Ctrl Pts',(-1.59998683424193,4.88121323983623,13.4516755350231));
#10564=CARTESIAN_POINT('Ctrl Pts',(-1.70474236547937,4.84687598338817,13.4576535565028));
#10565=CARTESIAN_POINT('Ctrl Pts',(-1.8083813997389,4.8091687674524,13.4636315779825));
#10566=CARTESIAN_POINT('Ctrl Pts',(-1.91068652245528,4.76817340030831,13.4696095994622));
#10567=CARTESIAN_POINT('Ctrl Pts',(-2.04876339914168,4.71284369536714,13.4776778810181));
#10568=CARTESIAN_POINT('Ctrl Pts',(-2.18446082938609,4.65150207913866,13.4857461625739));
#10569=CARTESIAN_POINT('Ctrl Pts',(-2.31725599231094,4.5843783906435,13.4938144441298));
#10570=CARTESIAN_POINT('Ctrl Pts',(-2.45002435507905,4.51726824876654,13.5018810973793));
#10571=CARTESIAN_POINT('Ctrl Pts',(-2.57989132382215,4.44437851188141,13.5099477506287));
#10572=CARTESIAN_POINT('Ctrl Pts',(-2.70635716787987,4.36598573547432,13.5180144038782));
#10573=CARTESIAN_POINT('Ctrl Pts',(-2.83282757094512,4.28759013306104,13.526081347925));
#10574=CARTESIAN_POINT('Ctrl Pts',(-2.95589632064838,4.20369126532515,13.5341482919719));
#10575=CARTESIAN_POINT('Ctrl Pts',(-3.07509077516368,4.11461022297413,13.5422152360187));
#10576=CARTESIAN_POINT('Ctrl Pts',(-3.19427801944507,4.02553456925596,13.5502816920851));
#10577=CARTESIAN_POINT('Ctrl Pts',(-3.30959117273334,3.93127756688894,13.5583481481516));
#10578=CARTESIAN_POINT('Ctrl Pts',(-3.42058892981839,3.83220196958666,13.5664146042181));
#10579=CARTESIAN_POINT('Ctrl Pts',(-3.53161438758902,3.73310164690216,13.5744830733555));
#10580=CARTESIAN_POINT('Ctrl Pts',(-3.63832204968099,3.62918054642988,13.5825515424929));
#10581=CARTESIAN_POINT('Ctrl Pts',(-3.74030537708679,3.52084027593352,13.5906200116304));
#10582=CARTESIAN_POINT('Ctrl Pts',(-3.81586599601171,3.44056972484016,13.5965980331101));
#10583=CARTESIAN_POINT('Ctrl Pts',(-3.88883390261718,3.35787408915469,13.6025760545898));
#10584=CARTESIAN_POINT('Ctrl Pts',(-3.95905731897123,3.2729292243494,13.6085540760694));
#10585=CARTESIAN_POINT('Ctrl Pts',(-4.0538341891485,3.15828358558858,13.6166222988235));
#10586=CARTESIAN_POINT('Ctrl Pts',(-4.14364540353534,3.03949718774696,13.6246905215776));
#10587=CARTESIAN_POINT('Ctrl Pts',(-4.22814182866341,2.91702198126905,13.6327587443317));
#10588=CARTESIAN_POINT('Ctrl Pts',(-4.24972153642287,2.88574279804247,13.6348193035673));
#10589=CARTESIAN_POINT('Ctrl Pts',(-4.2709547958896,2.85422317469389,13.6368798628028));
#10590=CARTESIAN_POINT('Ctrl Pts',(-4.29183622825304,2.82247096572396,13.6389404220384));
#10591=CARTESIAN_POINT('Ctrl Pts',(-4.29183623954907,2.82247094854727,13.1619495546845));
#10592=CARTESIAN_POINT('Ctrl Pts',(-4.27694788375811,2.84511011334144,13.1604648429513));
#10593=CARTESIAN_POINT('Ctrl Pts',(-4.26187904818184,2.86763352754246,13.1589805421803));
#10594=CARTESIAN_POINT('Ctrl Pts',(-4.16093974471724,3.01595400996317,13.1491586060886));
#10595=CARTESIAN_POINT('Ctrl Pts',(-4.06968960576698,3.137997118523,13.1408514072985));
#10596=CARTESIAN_POINT('Ctrl Pts',(-3.77192941324118,3.50136210079973,13.1153590904081));
#10597=CARTESIAN_POINT('Ctrl Pts',(-3.54837648818902,3.72773607014882,13.0984083992163));
#10598=CARTESIAN_POINT('Ctrl Pts',(-3.20264554166019,4.01836621106547,13.0741672541801));
#10599=CARTESIAN_POINT('Ctrl Pts',(-3.09659155107452,4.10064938220204,13.0669512453703));
#10600=CARTESIAN_POINT('Ctrl Pts',(-2.83464457250743,4.28792130895749,13.0494663601919));
#10601=CARTESIAN_POINT('Ctrl Pts',(-2.67597616762272,4.38869330300458,13.0391599348284));
#10602=CARTESIAN_POINT('Ctrl Pts',(-2.31975579620537,4.58841852998751,13.0167674912027));
#10603=CARTESIAN_POINT('Ctrl Pts',(-2.12061153784892,4.68378711199637,13.0047114042907));
#10604=CARTESIAN_POINT('Ctrl Pts',(-1.64006458124989,4.87696655148323,12.9766174890269));
#10605=CARTESIAN_POINT('Ctrl Pts',(-1.35506677707031,4.96370954684383,12.9607238377605));
#10606=CARTESIAN_POINT('Ctrl Pts',(-0.921521330346854,5.05551767954514,
12.9369501121487));
#10607=CARTESIAN_POINT('Ctrl Pts',(-0.777657732610997,5.07963658288696,
12.9291176039509));
#10608=CARTESIAN_POINT('Ctrl Pts',(-0.430106790533545,5.12279168066443,
12.9101078301565));
#10609=CARTESIAN_POINT('Ctrl Pts',(-0.225928294720977,5.13584861424016,
12.8988839253612));
#10610=CARTESIAN_POINT('Ctrl Pts',(0.2024130186388,5.1376430220503,12.8754016531683));
#10611=CARTESIAN_POINT('Ctrl Pts',(0.426170633355844,5.12393688968866,12.8631745524838));
#10612=CARTESIAN_POINT('Ctrl Pts',(0.894375700366544,5.06436719888638,12.8376028269245));
#10613=CARTESIAN_POINT('Ctrl Pts',(1.1378409355763,5.01528105320431,12.8243159654074));
#10614=CARTESIAN_POINT('Ctrl Pts',(1.54133081496255,4.90302585910194,12.8018610211369));
#10615=CARTESIAN_POINT('Ctrl Pts',(1.70346547231188,4.84907893628779,12.792708243885));
#10616=CARTESIAN_POINT('Ctrl Pts',(2.03990341334884,4.71817620875839,12.773131893461));
#10617=CARTESIAN_POINT('Ctrl Pts',(2.21322660189523,4.63939850648156,12.7626962755128));
#10618=CARTESIAN_POINT('Ctrl Pts',(2.57759304934542,4.4487144054424,12.7401458882247));
#10619=CARTESIAN_POINT('Ctrl Pts',(2.76659457459465,4.33370552808602,12.7280595992305));
#10620=CARTESIAN_POINT('Ctrl Pts',(3.21258915589885,4.02121390944499,12.6985047889758));
#10621=CARTESIAN_POINT('Ctrl Pts',(3.45944206411802,3.8109257157081,12.6812347620744));
#10622=CARTESIAN_POINT('Ctrl Pts',(3.77618668904046,3.48479454645855,12.65683021443));
#10623=CARTESIAN_POINT('Ctrl Pts',(3.86386780007027,3.38731512600791,12.6497794423507));
#10624=CARTESIAN_POINT('Ctrl Pts',(4.06474417199863,3.14603018619013,12.6327292376255));
#10625=CARTESIAN_POINT('Ctrl Pts',(4.17417195529512,2.99932292928893,12.622695197408));
#10626=CARTESIAN_POINT('Ctrl Pts',(4.39679822601708,2.66500050505871,12.600670836019));
#10627=CARTESIAN_POINT('Ctrl Pts',(4.50630075151071,2.47534223162136,12.5887092463883));
#10628=CARTESIAN_POINT('Ctrl Pts',(4.74450149151707,1.99425659393549,12.5595784550069));
#10629=CARTESIAN_POINT('Ctrl Pts',(4.85884977599643,1.696742899886,12.5425975696677));
#10630=CARTESIAN_POINT('Ctrl Pts',(4.98119209192641,1.26168531451468,12.5183413937063));
#10631=CARTESIAN_POINT('Ctrl Pts',(5.01238159027475,1.1314390876598,12.5111414052029));
#10632=CARTESIAN_POINT('Ctrl Pts',(5.07492676279779,0.816347627802187,12.4936978806807));
#10633=CARTESIAN_POINT('Ctrl Pts',(5.10132354831581,0.630715080651572,12.483417067094));
#10634=CARTESIAN_POINT('Ctrl Pts',(5.13619445156669,0.228848147858504,12.4612994593529));
#10635=CARTESIAN_POINT('Ctrl Pts',(5.14127489907074,0.0126700805803074,
12.449490302741));
#10636=CARTESIAN_POINT('Ctrl Pts',(5.12024888680174,-0.518468830665231,
12.4206471108741));
#10637=CARTESIAN_POINT('Ctrl Pts',(5.07874522800982,-0.831931102533435,
12.4037983456324));
#10638=CARTESIAN_POINT('Ctrl Pts',(4.97874548083299,-1.27144673564097,12.3796072818303));
#10639=CARTESIAN_POINT('Ctrl Pts',(4.94355449794596,-1.40205256011753,12.3723365704161));
#10640=CARTESIAN_POINT('Ctrl Pts',(4.84680110178377,-1.71189584239804,12.354711560401));
#10641=CARTESIAN_POINT('Ctrl Pts',(4.78039617850477,-1.88941234290117,12.3443188062455));
#10642=CARTESIAN_POINT('Ctrl Pts',(4.61609835217616,-2.26409390721354,12.3218866113472));
#10643=CARTESIAN_POINT('Ctrl Pts',(4.51503098505734,-2.45946820235544,12.3098767248542));
#10644=CARTESIAN_POINT('Ctrl Pts',(4.24939101342763,-2.90107875766833,12.2819232038512));
#10645=CARTESIAN_POINT('Ctrl Pts',(4.07543835190121,-3.14076233381926,12.2661211137436));
#10646=CARTESIAN_POINT('Ctrl Pts',(3.78561896444567,-3.47517974901731,12.2423821719534));
#10647=CARTESIAN_POINT('Ctrl Pts',(3.68468308490064,-3.58202380726063,12.2344908577794));
#10648=CARTESIAN_POINT('Ctrl Pts',(3.43154529156971,-3.82794166823245,12.2153349307228));
#10649=CARTESIAN_POINT('Ctrl Pts',(3.27528254605842,-3.96246928792975,12.2040228135355));
#10650=CARTESIAN_POINT('Ctrl Pts',(2.93407652322816,-4.22220814896818,12.1805151065899));
#10651=CARTESIAN_POINT('Ctrl Pts',(2.74818948803948,-4.34549249156184,12.16834989307));
#10652=CARTESIAN_POINT('Ctrl Pts',(2.34821702770868,-4.57480346760217,12.1433710880637));
#10653=CARTESIAN_POINT('Ctrl Pts',(2.13355075891114,-4.67877349436502,12.1306018926181));
#10654=CARTESIAN_POINT('Ctrl Pts',(1.74199567743333,-4.83584349816913,12.1079834482912));
#10655=CARTESIAN_POINT('Ctrl Pts',(1.56801725073646,-4.89502230494025,12.098147981642));
#10656=CARTESIAN_POINT('Ctrl Pts',(1.22081083018172,-4.99271168462182,12.0785802687795));
#10657=CARTESIAN_POINT('Ctrl Pts',(1.04801034427448,-5.03182091013587,12.0688728460095));
#10658=CARTESIAN_POINT('Ctrl Pts',(0.75894002071506,-5.08170587791294,12.0527870960109));
#10659=CARTESIAN_POINT('Ctrl Pts',(0.64370193501755,-5.09758498577776,12.0464129556961));
#10660=CARTESIAN_POINT('Ctrl Pts',(0.447458996757989,-5.11786489007452,
12.0356294002439));
#10661=CARTESIAN_POINT('Ctrl Pts',(0.366707872342953,-5.12428396099191,
12.031212166141));
#10662=CARTESIAN_POINT('Ctrl Pts',(0.1138367927602,-5.13837699370879,12.0174358132956));
#10663=CARTESIAN_POINT('Ctrl Pts',(-0.0585403322878479,-5.13930460856412,
12.0081294257262));
#10664=CARTESIAN_POINT('Ctrl Pts',(-0.534759809341479,-5.11790073709783,
11.9824861011697));
#10665=CARTESIAN_POINT('Ctrl Pts',(-0.837055304337044,-5.07722433240468,
11.9663083528191));
#10666=CARTESIAN_POINT('Ctrl Pts',(-1.32000612392216,-4.96791415071457,
11.9394573374936));
#10667=CARTESIAN_POINT('Ctrl Pts',(-1.50356008218921,-4.91547475334482,
11.9289935131619));
#10668=CARTESIAN_POINT('Ctrl Pts',(-1.89279561245778,-4.78042648073306,
11.906401947339));
#10669=CARTESIAN_POINT('Ctrl Pts',(-2.09692245108785,-4.69447251309896,
11.8943028392958));
#10670=CARTESIAN_POINT('Ctrl Pts',(-2.59734217930105,-4.44458269703522,
11.8639478713378));
#10671=CARTESIAN_POINT('Ctrl Pts',(-2.88416196309347,-4.26404908910189,
11.8459240815326));
#10672=CARTESIAN_POINT('Ctrl Pts',(-3.24638423165515,-3.98267858431652,
11.8212860429036));
#10673=CARTESIAN_POINT('Ctrl Pts',(-3.33897108149012,-3.90538229021187,
11.8147912500703));
#10674=CARTESIAN_POINT('Ctrl Pts',(-3.58248587675597,-3.68708847015701,
11.7970207386546));
#10675=CARTESIAN_POINT('Ctrl Pts',(-3.72776945354604,-3.54013555732661,
11.7856806415028));
#10676=CARTESIAN_POINT('Ctrl Pts',(-4.00583540217605,-3.22272186408579,
11.7625517642465));
#10677=CARTESIAN_POINT('Ctrl Pts',(-4.13751607794587,-3.05182202124432,
11.7507893483979));
#10678=CARTESIAN_POINT('Ctrl Pts',(-4.40844481800982,-2.65030002825791,
11.7245500082159));
#10679=CARTESIAN_POINT('Ctrl Pts',(-4.54109025864236,-2.41598390962851,
11.7101701848864));
#10680=CARTESIAN_POINT('Ctrl Pts',(-4.71976620185243,-2.03312951712328,
11.6875101452456));
#10681=CARTESIAN_POINT('Ctrl Pts',(-4.7784646404832,-1.89105337558102,11.679261924774));
#10682=CARTESIAN_POINT('Ctrl Pts',(-4.88758287393664,-1.58925028925234,
11.6618454136832));
#10683=CARTESIAN_POINT('Ctrl Pts',(-4.93674089618645,-1.42925528175306,
11.6526772545995));
#10684=CARTESIAN_POINT('Ctrl Pts',(-5.02105464071223,-1.09802838236001,
11.633935117075));
#10685=CARTESIAN_POINT('Ctrl Pts',(-5.05545848627692,-0.92682079579276,
11.6243733966469));
#10686=CARTESIAN_POINT('Ctrl Pts',(-5.09239223521895,-0.677994207856829,
11.6106635818307));
#10687=CARTESIAN_POINT('Ctrl Pts',(-5.10198717475003,-0.601549559696101,
11.606475931118));
#10688=CARTESIAN_POINT('Ctrl Pts',(-5.1277785174244,-0.350481287022635,
11.5927912891983));
#10689=CARTESIAN_POINT('Ctrl Pts',(-5.13675406642089,-0.175239897197318,
11.5833522487284));
#10690=CARTESIAN_POINT('Ctrl Pts',(-5.13674532147658,0.201746395123558,
11.5631162684455));
#10691=CARTESIAN_POINT('Ctrl Pts',(-5.12486929042445,0.403196514690206,
11.5523466561477));
#10692=CARTESIAN_POINT('Ctrl Pts',(-5.08956653666402,0.701636399335537,
11.5361450535164));
#10693=CARTESIAN_POINT('Ctrl Pts',(-5.07511543220857,0.799489803161525,
11.5307860856218));
#10694=CARTESIAN_POINT('Ctrl Pts',(-5.01650915027294,1.12999859525954,11.512486978629));
#10695=CARTESIAN_POINT('Ctrl Pts',(-4.9591002514135,1.35999468364453,11.4994660930734));
#10696=CARTESIAN_POINT('Ctrl Pts',(-4.83030861967047,1.75696454065474,11.4766397854257));
#10697=CARTESIAN_POINT('Ctrl Pts',(-4.76556619713695,1.92566529187235,11.4668168454676));
#10698=CARTESIAN_POINT('Ctrl Pts',(-4.66008657145207,2.1623993146635,11.452801983407));
#10699=CARTESIAN_POINT('Ctrl Pts',(-4.62645574087763,2.23344690984212,11.4485639156551));
#10700=CARTESIAN_POINT('Ctrl Pts',(-4.50159121627279,2.48229881749279,11.4335806477222));
#10701=CARTESIAN_POINT('Ctrl Pts',(-4.40163066974278,2.65551804842615,11.4229009965103));
#10702=CARTESIAN_POINT('Ctrl Pts',(-4.29183622844418,2.82247096543331,11.4121712634621));
#10703=CARTESIAN_POINT('Origin',(0.,0.,0.));
#10704=CARTESIAN_POINT('',(-4.29147790789384,2.82223516558083,9.66201704729454));
#10705=CARTESIAN_POINT('',(-4.29183622628417,2.82247096871782,10.1386883748835));
#10706=CARTESIAN_POINT('',(-4.29183622825304,2.82247096572397,0.));
#10707=CARTESIAN_POINT('',(-5.13684723413363,0.000128082860076971,10.3009584946969));
#10708=CARTESIAN_POINT('Ctrl Pts',(-4.29183622628417,2.82247096871782,10.1386883748835));
#10709=CARTESIAN_POINT('Ctrl Pts',(-4.34083109202366,2.74796960377439,10.1435395218449));
#10710=CARTESIAN_POINT('Ctrl Pts',(-4.38788013653966,2.672201517456,10.1484139523655));
#10711=CARTESIAN_POINT('Ctrl Pts',(-4.56670902924153,2.36674391274659,10.1677992315681));
#10712=CARTESIAN_POINT('Ctrl Pts',(-4.68261820116927,2.12823849428426,10.1823314494109));
#10713=CARTESIAN_POINT('Ctrl Pts',(-4.83954528871763,1.72966906163324,10.2056276174853));
#10714=CARTESIAN_POINT('Ctrl Pts',(-4.892164775472,1.57469968683397,10.2144657681278));
#10715=CARTESIAN_POINT('Ctrl Pts',(-5.02439454951934,1.11412362911239,10.2402507046387));
#10716=CARTESIAN_POINT('Ctrl Pts',(-5.08334220896111,0.803390581211435,
10.257011770707));
#10717=CARTESIAN_POINT('Ctrl Pts',(-5.12895407492712,0.326652854974812,
10.2829990761926));
#10718=CARTESIAN_POINT('Ctrl Pts',(-5.13674602407281,0.163434288575042,
10.2919476345316));
#10719=CARTESIAN_POINT('Ctrl Pts',(-5.13674999847882,0.00012501145318828,
10.3009025249688));
#10720=CARTESIAN_POINT('Ctrl Pts',(-5.13684723413363,0.000128082860076971,
10.3009584946969));
#10721=CARTESIAN_POINT('Ctrl Pts',(-5.13614064254843,-0.687574204925511,
10.3382493678326));
#10722=CARTESIAN_POINT('Ctrl Pts',(-4.82448783135896,-2.23001569616463,
10.4218550665042));
#10723=CARTESIAN_POINT('Ctrl Pts',(-3.32632042058165,-4.19626932876706,
10.5517755907113));
#10724=CARTESIAN_POINT('Ctrl Pts',(-0.913310824303407,-5.27626261269656,
10.6907200673184));
#10725=CARTESIAN_POINT('Ctrl Pts',(1.72231626671068,-5.07017854689106,10.8296645439257));
#10726=CARTESIAN_POINT('Ctrl Pts',(3.93813257454472,-3.6282496668833,10.9686090205328));
#10727=CARTESIAN_POINT('Ctrl Pts',(5.19403777177804,-1.3019429500838,11.10755349714));
#10728=CARTESIAN_POINT('Ctrl Pts',(5.18390774250871,1.34170948311754,11.2464979737472));
#10729=CARTESIAN_POINT('Ctrl Pts',(3.91021165898081,3.65832319538621,11.3854424503544));
#10730=CARTESIAN_POINT('Ctrl Pts',(1.68341012630706,5.08322871476155,11.5243869269616));
#10731=CARTESIAN_POINT('Ctrl Pts',(-0.953718903816859,5.26910847036118,
11.6633314035688));
#10732=CARTESIAN_POINT('Ctrl Pts',(-3.05672897793555,4.30844986953081,11.7848460343876));
#10733=CARTESIAN_POINT('Ctrl Pts',(-3.99850791102981,3.26727227258147,11.8600458396708));
#10734=CARTESIAN_POINT('Ctrl Pts',(-4.29155726418515,2.82228712074135,11.8889308194183));
#10735=CARTESIAN_POINT('',(-5.13658335629485,-0.000126015287452153,9.82404150530312));
#10736=CARTESIAN_POINT('Ctrl Pts',(-4.29183622844418,2.82247096543331,11.4121712634621));
#10737=CARTESIAN_POINT('Ctrl Pts',(-4.28994791435063,2.82534232706525,11.4119867267416));
#10738=CARTESIAN_POINT('Ctrl Pts',(-4.28805669151549,2.82821183506285,11.4118021730424));
#10739=CARTESIAN_POINT('Ctrl Pts',(-4.2474485640806,2.8896912235692,11.4078451540581));
#10740=CARTESIAN_POINT('Ctrl Pts',(-4.20753668038186,2.94750226562249,11.4040669279646));
#10741=CARTESIAN_POINT('Ctrl Pts',(-4.10824353578134,3.08519686448068,11.3949026479613));
#10742=CARTESIAN_POINT('Ctrl Pts',(-4.04770306037154,3.16420666041538,11.3894981061057));
#10743=CARTESIAN_POINT('Ctrl Pts',(-3.9029307218828,3.34218623597612,11.3769747001215));
#10744=CARTESIAN_POINT('Ctrl Pts',(-3.8171617097086,3.43981876560561,11.3698496147885));
#10745=CARTESIAN_POINT('Ctrl Pts',(-3.56864371293256,3.7019571099109,11.3500426044299));
#10746=CARTESIAN_POINT('Ctrl Pts',(-3.39834304240547,3.85888233888637,11.3373971069978));
#10747=CARTESIAN_POINT('Ctrl Pts',(-3.04479348620101,4.14304715807517,11.3127984920234));
#10748=CARTESIAN_POINT('Ctrl Pts',(-2.8626847733648,4.27090691818338,11.3008621114949));
#10749=CARTESIAN_POINT('Ctrl Pts',(-2.49628564729489,4.49416459800045,11.2778550967654));
#10750=CARTESIAN_POINT('Ctrl Pts',(-2.31337396437934,4.59099719008163,11.2668007368887));
#10751=CARTESIAN_POINT('Ctrl Pts',(-1.99090324041689,4.73753541914524,11.2476015538077));
#10752=CARTESIAN_POINT('Ctrl Pts',(-1.85411610055745,4.79272254575252,11.2395343469497));
#10753=CARTESIAN_POINT('Ctrl Pts',(-1.43727006089289,4.94038058340897,11.2152934471992));
#10754=CARTESIAN_POINT('Ctrl Pts',(-1.15142682466936,5.01471131485522,11.1991520408148));
#10755=CARTESIAN_POINT('Ctrl Pts',(-0.64452096905599,5.10087395656544,11.171300297607));
#10756=CARTESIAN_POINT('Ctrl Pts',(-0.426121213311639,5.12374332014506,
11.1595314524612));
#10757=CARTESIAN_POINT('Ctrl Pts',(-0.0169939703559984,5.14023781924363,
11.1375784423278));
#10758=CARTESIAN_POINT('Ctrl Pts',(0.173214079208224,5.1373463946278,11.1274065948019));
#10759=CARTESIAN_POINT('Ctrl Pts',(0.498162248590264,5.11433714102349,11.1097555289829));
#10760=CARTESIAN_POINT('Ctrl Pts',(0.633069238389082,5.0993952412627,11.102338301211));
#10761=CARTESIAN_POINT('Ctrl Pts',(1.0783485223739,5.03213401156622,11.0776624747847));
#10762=CARTESIAN_POINT('Ctrl Pts',(1.38450712203306,4.95664781813367,11.0604240957339));
#10763=CARTESIAN_POINT('Ctrl Pts',(1.90152583266395,4.77749519085442,11.0307954595874));
#10764=CARTESIAN_POINT('Ctrl Pts',(2.11579872560115,4.686540208976,11.018335390638));
#10765=CARTESIAN_POINT('Ctrl Pts',(2.48246751895757,4.50060603847139,10.9962940172645));
#10766=CARTESIAN_POINT('Ctrl Pts',(2.63743670803161,4.41157850905834,10.9867261142502));
#10767=CARTESIAN_POINT('Ctrl Pts',(3.05750386593181,4.14019777102209,10.9596040627519));
#10768=CARTESIAN_POINT('Ctrl Pts',(3.31058060893463,3.94076439789699,10.9418788746898));
#10769=CARTESIAN_POINT('Ctrl Pts',(3.66590715162429,3.60221876841865,10.9150897212574));
#10770=CARTESIAN_POINT('Ctrl Pts',(3.782618036974,3.47946231159423,10.9059042506902));
#10771=CARTESIAN_POINT('Ctrl Pts',(4.11356483860027,3.09500071104522,10.8785226599394));
#10772=CARTESIAN_POINT('Ctrl Pts',(4.3082478311266,2.8177011514594,10.8605818924567));
#10773=CARTESIAN_POINT('Ctrl Pts',(4.5260579832811,2.43148329251716,10.8366112656184));
#10774=CARTESIAN_POINT('Ctrl Pts',(4.57499822588214,2.33809795426995,10.8308730381771));
#10775=CARTESIAN_POINT('Ctrl Pts',(4.69208663977523,2.09690194140828,10.8162166512067));
#10776=CARTESIAN_POINT('Ctrl Pts',(4.75614850802074,1.94723547338733,10.8072825660391));
#10777=CARTESIAN_POINT('Ctrl Pts',(4.87725248574582,1.62247550730087,10.7882956303873));
#10778=CARTESIAN_POINT('Ctrl Pts',(4.93220779666497,1.44684035708545,10.7782636247326));
#10779=CARTESIAN_POINT('Ctrl Pts',(5.03496889322559,1.04364591474228,10.7557066859083));
#10780=CARTESIAN_POINT('Ctrl Pts',(5.07699163525871,0.815026068638081,10.7432498333393));
#10781=CARTESIAN_POINT('Ctrl Pts',(5.12490878482816,0.396540013934391,10.7206663874709));
#10782=CARTESIAN_POINT('Ctrl Pts',(5.13602910212463,0.207693518775206,10.7105503519872));
#10783=CARTESIAN_POINT('Ctrl Pts',(5.13720662253577,-0.116308156197909,
10.6929950160979));
#10784=CARTESIAN_POINT('Ctrl Pts',(5.13237683428155,-0.251248834867124,
10.6856167286514));
#10785=CARTESIAN_POINT('Ctrl Pts',(5.09850530505004,-0.700912836497425,
10.6609083338576));
#10786=CARTESIAN_POINT('Ctrl Pts',(5.04575103091411,-1.01313430145774,10.6435975141725));
#10787=CARTESIAN_POINT('Ctrl Pts',(4.90513714330223,-1.54258652848114,10.6139356606848));
#10788=CARTESIAN_POINT('Ctrl Pts',(4.83053091859768,-1.7623612582539,10.6015120011097));
#10789=CARTESIAN_POINT('Ctrl Pts',(4.67246591390906,-2.14156558158247,10.5794861141244));
#10790=CARTESIAN_POINT('Ctrl Pts',(4.59500939537069,-2.30306906815642,10.5698972670432));
#10791=CARTESIAN_POINT('Ctrl Pts',(4.42726639454091,-2.61052450520569,10.5509026113368));
#10792=CARTESIAN_POINT('Ctrl Pts',(4.33778470847257,-2.75665521805149,10.5415176360143));
#10793=CARTESIAN_POINT('Ctrl Pts',(4.09994198056717,-3.10472908850223,10.5184005935865));
#10794=CARTESIAN_POINT('Ctrl Pts',(3.94378684083705,-3.30082067618229,10.5047047641667));
#10795=CARTESIAN_POINT('Ctrl Pts',(3.62214065505836,-3.64916123866251,10.4789931638158));
#10796=CARTESIAN_POINT('Ctrl Pts',(3.45974175700126,-3.80348137401556,10.4669770503808));
#10797=CARTESIAN_POINT('Ctrl Pts',(3.1305729833851,-4.07769373658459,10.4440048452982));
#10798=CARTESIAN_POINT('Ctrl Pts',(2.96566780625345,-4.19915286595873,10.4330639655872));
#10799=CARTESIAN_POINT('Ctrl Pts',(2.67148765708166,-4.3898355796708,10.4140623026202));
#10800=CARTESIAN_POINT('Ctrl Pts',(2.54568756441235,-4.46396414770112,10.4060770551772));
#10801=CARTESIAN_POINT('Ctrl Pts',(2.15473449075717,-4.67242933519697,10.3817913667956));
#10802=CARTESIAN_POINT('Ctrl Pts',(1.88092231938915,-4.78921870273098,10.3655220146556));
#10803=CARTESIAN_POINT('Ctrl Pts',(1.38903662920752,-4.95029095580603,10.3374866115439));
#10804=CARTESIAN_POINT('Ctrl Pts',(1.17532187686411,-5.00533957868389,10.3256602702292));
#10805=CARTESIAN_POINT('Ctrl Pts',(0.773999581664107,-5.08158264302437,
10.303758895609));
#10806=CARTESIAN_POINT('Ctrl Pts',(0.587484770776609,-5.10650728876771,
10.2936957441874));
#10807=CARTESIAN_POINT('Ctrl Pts',(0.26611697357661,-5.13161026139412,10.276230647042));
#10808=CARTESIAN_POINT('Ctrl Pts',(0.131850023161423,-5.13681381527077,
10.2688887876281));
#10809=CARTESIAN_POINT('Ctrl Pts',(-0.319670293464739,-5.13659730232582,
10.24414915484));
#10810=CARTESIAN_POINT('Ctrl Pts',(-0.636191331126812,-5.10706286114678,
10.226769772693));
#10811=CARTESIAN_POINT('Ctrl Pts',(-1.16368883788394,-5.00801422346111,
10.1977091727481));
#10812=CARTESIAN_POINT('Ctrl Pts',(-1.37659671361609,-4.95372203897602,
10.1859381440721));
#10813=CARTESIAN_POINT('Ctrl Pts',(-1.75878345598588,-4.82971176552803,
10.1643962789253));
#10814=CARTESIAN_POINT('Ctrl Pts',(-1.92906550853401,-4.76425639343368,
10.1546368134859));
#10815=CARTESIAN_POINT('Ctrl Pts',(-2.21484103151283,-4.63656815932604,
10.1376804923676));
#10816=CARTESIAN_POINT('Ctrl Pts',(-2.3320969802161,-4.57871240481641,10.1305383988846));
#10817=CARTESIAN_POINT('Ctrl Pts',(-2.73213353207538,-4.36197227744395,
10.1056133316696));
#10818=CARTESIAN_POINT('Ctrl Pts',(-3.00199190604444,-4.18083849722328,
10.0878433831701));
#10819=CARTESIAN_POINT('Ctrl Pts',(-3.42441108922433,-3.8351897508475,10.0582948030191));
#10820=CARTESIAN_POINT('Ctrl Pts',(-3.5865992131806,-3.68396256473145,10.0464181690309));
#10821=CARTESIAN_POINT('Ctrl Pts',(-3.86831467972195,-3.38499081771354,
10.0243946730317));
#10822=CARTESIAN_POINT('Ctrl Pts',(-3.99039562212548,-3.24017923506791,
10.0142615884703));
#10823=CARTESIAN_POINT('Ctrl Pts',(-4.15204132140484,-3.02540601636154,
9.99967824203985));
#10824=CARTESIAN_POINT('Ctrl Pts',(-4.19839473964942,-2.96074484281005,
9.99534049302957));
#10825=CARTESIAN_POINT('Ctrl Pts',(-4.33817387080808,-2.7558717423584,9.98178039695737));
#10826=CARTESIAN_POINT('Ctrl Pts',(-4.42621679630225,-2.61212296408422,
9.97252916752709));
#10827=CARTESIAN_POINT('Ctrl Pts',(-4.60079611551422,-2.2928304044208,9.95260019882058));
#10828=CARTESIAN_POINT('Ctrl Pts',(-4.68469406441972,-2.11613808559128,
9.94194944602537));
#10829=CARTESIAN_POINT('Ctrl Pts',(-4.8157527953289,-1.79386956005154,9.92311509375324));
#10830=CARTESIAN_POINT('Ctrl Pts',(-4.86686984338799,-1.65015817626784,
9.91491157199256));
#10831=CARTESIAN_POINT('Ctrl Pts',(-4.98332760266446,-1.26994653246926,
9.89356600498713));
#10832=CARTESIAN_POINT('Ctrl Pts',(-5.03825652933309,-1.03067216725358,
9.88049178783821));
#10833=CARTESIAN_POINT('Ctrl Pts',(-5.08249254213491,-0.745870143370513,
9.86488239127982));
#10834=CARTESIAN_POINT('Ctrl Pts',(-5.08856307846514,-0.703262702007987,
9.86254492289813));
#10835=CARTESIAN_POINT('Ctrl Pts',(-5.12249743520096,-0.44157785562199,
9.84817827333096));
#10836=CARTESIAN_POINT('Ctrl Pts',(-5.13674435468852,-0.220969231918046,
9.8360385854582));
#10837=CARTESIAN_POINT('Ctrl Pts',(-5.13674999832263,-0.000131272438793767,
9.82394557894206));
#10838=CARTESIAN_POINT('Ctrl Pts',(-5.13658335629485,-0.000126015287452153,
9.82404150530312));
#10839=CARTESIAN_POINT('Ctrl Pts',(-5.13603076124125,0.601945860711958,
9.79139879103644));
#10840=CARTESIAN_POINT('Ctrl Pts',(-4.96092370381945,1.59840118087525,9.73739063836703));
#10841=CARTESIAN_POINT('Ctrl Pts',(-4.50810837244381,2.49298111405563,9.68338248569762));
#10842=CARTESIAN_POINT('Ctrl Pts',(-4.29147790789737,2.82223516557546,9.66201704729489));
#10843=CARTESIAN_POINT('Origin',(0.,0.,0.));
#10844=CARTESIAN_POINT('',(-4.29183622825303,2.82247096572398,7.9120163777544));
#10845=CARTESIAN_POINT('',(-4.2918361854396,2.82247103082588,8.38917442239304));
#10846=CARTESIAN_POINT('',(-4.29183622825304,2.82247096572397,0.));
#10847=CARTESIAN_POINT('Ctrl Pts',(-4.2918361854396,2.82247103082587,8.38917442239304));
#10848=CARTESIAN_POINT('Ctrl Pts',(-4.32942666324407,2.7653111269306,8.39289704544047));
#10849=CARTESIAN_POINT('Ctrl Pts',(-4.36587935814393,2.70739398876421,8.3966115467939));
#10850=CARTESIAN_POINT('Ctrl Pts',(-4.53974565731834,2.41849759257399,8.41487322461712));
#10851=CARTESIAN_POINT('Ctrl Pts',(-4.66003820603287,2.17772084036754,8.42924495813878));
#10852=CARTESIAN_POINT('Ctrl Pts',(-4.81768645716247,1.78855813720054,8.45176628056113));
#10853=CARTESIAN_POINT('Ctrl Pts',(-4.86822148280676,1.64604411757638,8.45988135237389));
#10854=CARTESIAN_POINT('Ctrl Pts',(-4.96087873692471,1.34290348903069,8.47708499786189));
#10855=CARTESIAN_POINT('Ctrl Pts',(-5.001648045299,1.18204187236612,8.48617450672251));
#10856=CARTESIAN_POINT('Ctrl Pts',(-5.0692829089734,0.848040512523393,8.50486124080666));
#10857=CARTESIAN_POINT('Ctrl Pts',(-5.09522129246755,0.674924561328445,
8.51444624124013));
#10858=CARTESIAN_POINT('Ctrl Pts',(-5.1285844725791,0.334360770111465,8.53309680238365));
#10859=CARTESIAN_POINT('Ctrl Pts',(-5.13675206408452,0.167200064917802,
8.54215599106349));
#10860=CARTESIAN_POINT('Ctrl Pts',(-5.13674781081197,-0.177400897830959,
8.56072997932663));
#10861=CARTESIAN_POINT('Ctrl Pts',(-5.12756223984905,-0.354620084305676,
8.57022652294575));
#10862=CARTESIAN_POINT('Ctrl Pts',(-5.09291255051512,-0.688009915850673,
8.58819917488626));
#10863=CARTESIAN_POINT('Ctrl Pts',(-5.06936758864144,-0.844172066190319,
8.5966641612302));
#10864=CARTESIAN_POINT('Ctrl Pts',(-5.01134173026516,-1.13683823145349,
8.61283338519319));
#10865=CARTESIAN_POINT('Ctrl Pts',(-4.97836871468566,-1.27349537275126,
8.62051834504953));
#10866=CARTESIAN_POINT('Ctrl Pts',(-4.85591195726063,-1.70293260456988,
8.64499165791791));
#10867=CARTESIAN_POINT('Ctrl Pts',(-4.74585227860605,-1.98915940995312,
8.6617540699206));
#10868=CARTESIAN_POINT('Ctrl Pts',(-4.51168988908008,-2.46608947792636,
8.69052851677994));
#10869=CARTESIAN_POINT('Ctrl Pts',(-4.39921808421094,-2.66154574572552,
8.70260723033787));
#10870=CARTESIAN_POINT('Ctrl Pts',(-4.16806657052589,-3.00833749445266,
8.72495131001155));
#10871=CARTESIAN_POINT('Ctrl Pts',(-4.05302833689728,-3.16161858676421,
8.73520293859328));
#10872=CARTESIAN_POINT('Ctrl Pts',(-3.90379168677842,-3.33889651685975,
8.74777572921798));
#10873=CARTESIAN_POINT('Ctrl Pts',(-3.87751884141328,-3.36937191105137,
8.74996448116534));
#10874=CARTESIAN_POINT('Ctrl Pts',(-3.69660354323565,-3.57430729532129,
8.764864381742));
#10875=CARTESIAN_POINT('Ctrl Pts',(-3.53059768632202,-3.73837266183361,
8.77768418346644));
#10876=CARTESIAN_POINT('Ctrl Pts',(-3.21544982334438,-4.01005700651953,
8.80044795031635));
#10877=CARTESIAN_POINT('Ctrl Pts',(-3.07058983767729,-4.1220328871384,8.81040426448793));
#10878=CARTESIAN_POINT('Ctrl Pts',(-2.85568071382351,-4.27052832946172,
8.82453325447938));
#10879=CARTESIAN_POINT('Ctrl Pts',(-2.79029039042693,-4.31353732575679,
8.82875402004098));
#10880=CARTESIAN_POINT('Ctrl Pts',(-2.55512989400085,-4.46062306936487,
8.84368368490406));
#10881=CARTESIAN_POINT('Ctrl Pts',(-2.38032081507339,-4.55630552231217,
8.85432681695324));
#10882=CARTESIAN_POINT('Ctrl Pts',(-2.12261798781973,-4.67847229921776,
8.86963794109643));
#10883=CARTESIAN_POINT('Ctrl Pts',(-2.04392250491921,-4.71338420801666,
8.87426664389985));
#10884=CARTESIAN_POINT('Ctrl Pts',(-1.86995470124771,-4.78538557809084,
8.88443906677613));
#10885=CARTESIAN_POINT('Ctrl Pts',(-1.77437882957508,-4.82164127052871,
8.8899970342641));
#10886=CARTESIAN_POINT('Ctrl Pts',(-1.5392714222834,-4.90288914249991,8.90358666416002));
#10887=CARTESIAN_POINT('Ctrl Pts',(-1.39877136566293,-4.94480705344718,
8.91163020087048));
#10888=CARTESIAN_POINT('Ctrl Pts',(-1.05825295254069,-5.03072339208759,
8.93088047800941));
#10889=CARTESIAN_POINT('Ctrl Pts',(-0.857015884089,-5.06888585489178,8.94205571851761));
#10890=CARTESIAN_POINT('Ctrl Pts',(-0.430356935771449,-5.12365597973203,
8.96538236898676));
#10891=CARTESIAN_POINT('Ctrl Pts',(-0.205026528604712,-5.1376088565812,
8.9774898008687));
#10892=CARTESIAN_POINT('Ctrl Pts',(0.222658495080942,-5.13590256001789,
9.00042215367395));
#10893=CARTESIAN_POINT('Ctrl Pts',(0.424595931256993,-5.12316183784548,
9.01123296641682));
#10894=CARTESIAN_POINT('Ctrl Pts',(0.768382873847419,-5.08100215192302,
9.0300054891934));
#10895=CARTESIAN_POINT('Ctrl Pts',(0.910708465476806,-5.05743053196932,
9.03789399559456));
#10896=CARTESIAN_POINT('Ctrl Pts',(1.3454060112074,-4.9664906699621,9.06223595442882));
#10897=CARTESIAN_POINT('Ctrl Pts',(1.63302740111484,-4.87948527626849,9.07865984223037));
#10898=CARTESIAN_POINT('Ctrl Pts',(2.11734392780056,-4.68532579871062,9.10692137379542));
#10899=CARTESIAN_POINT('Ctrl Pts',(2.31771092573,-4.58951432417861,9.11882139747107));
#10900=CARTESIAN_POINT('Ctrl Pts',(2.67299298145714,-4.39040808357771,9.1406565700454));
#10901=CARTESIAN_POINT('Ctrl Pts',(2.82970033856075,-4.29108007870171,9.15058029104005));
#10902=CARTESIAN_POINT('Ctrl Pts',(3.08870354238832,-4.10654355515846,9.16780972892288));
#10903=CARTESIAN_POINT('Ctrl Pts',(3.19369232684526,-4.02543381076006,9.17505780346289));
#10904=CARTESIAN_POINT('Ctrl Pts',(3.54125067764628,-3.73476160166513,9.19988140672701));
#10905=CARTESIAN_POINT('Ctrl Pts',(3.76730783603636,-3.50660834278117,9.21744096575631));
#10906=CARTESIAN_POINT('Ctrl Pts',(4.11209520275527,-3.0865181355885,9.24686493306114));
#10907=CARTESIAN_POINT('Ctrl Pts',(4.24218806005543,-2.90512719706977,9.25881979989336));
#10908=CARTESIAN_POINT('Ctrl Pts',(4.45998145893393,-2.55547777415373,9.28090461136454));
#10909=CARTESIAN_POINT('Ctrl Pts',(4.55095273561851,-2.38971292614888,9.29102088209895));
#10910=CARTESIAN_POINT('Ctrl Pts',(4.70763340107648,-2.06265913850851,9.31069510406448));
#10911=CARTESIAN_POINT('Ctrl Pts',(4.77468752598387,-1.90229659749899,9.32021743700051));
#10912=CARTESIAN_POINT('Ctrl Pts',(4.91655960543361,-1.50793391116183,9.34319946234509));
#10913=CARTESIAN_POINT('Ctrl Pts',(4.9829785750852,-1.27135838606004,9.35662279810002));
#10914=CARTESIAN_POINT('Ctrl Pts',(5.07717176535824,-0.811581733700417,
9.38207393788696));
#10915=CARTESIAN_POINT('Ctrl Pts',(5.10772062678173,-0.589517568411141,
9.39409681822295));
#10916=CARTESIAN_POINT('Ctrl Pts',(5.13825617788038,-0.162240924357992,
9.41706605270614));
#10917=CARTESIAN_POINT('Ctrl Pts',(5.14064202539698,0.0423692804226592,
9.42799728093886));
#10918=CARTESIAN_POINT('Ctrl Pts',(5.12382892039803,0.392227266607594,9.44698197646185));
#10919=CARTESIAN_POINT('Ctrl Pts',(5.11063011848982,0.537515763965234,9.45496008194773));
#10920=CARTESIAN_POINT('Ctrl Pts',(5.0517920130541,0.976726816741831,9.47924978230916));
#10921=CARTESIAN_POINT('Ctrl Pts',(4.98680389238003,1.2674354846541,9.49553039678682));
#10922=CARTESIAN_POINT('Ctrl Pts',(4.83044261394475,1.76115612285127,9.52358208494756));
#10923=CARTESIAN_POINT('Ctrl Pts',(4.7503775364277,1.96691700526646,9.53541360440793));
#10924=CARTESIAN_POINT('Ctrl Pts',(4.57809158669411,2.33721314615637,9.5573103080189));
#10925=CARTESIAN_POINT('Ctrl Pts',(4.48956731930333,2.50305227564106,9.56736364606978));
#10926=CARTESIAN_POINT('Ctrl Pts',(4.32257337074313,2.77841121080462,9.58481201868659));
#10927=CARTESIAN_POINT('Ctrl Pts',(4.2485169968991,2.89038253748007,9.59214713848556));
#10928=CARTESIAN_POINT('Ctrl Pts',(3.98481282681463,3.25702842951064,9.616892617349));
#10929=CARTESIAN_POINT('Ctrl Pts',(3.77596713451508,3.49700574906384,9.63428475367893));
#10930=CARTESIAN_POINT('Ctrl Pts',(3.49043469271816,3.76948679348533,9.6556548384305));
#10931=CARTESIAN_POINT('Ctrl Pts',(3.43336716062839,3.8215383215272,9.65982465083243));
#10932=CARTESIAN_POINT('Ctrl Pts',(3.23692358867472,3.99276182997105,9.67386403913218));
#10933=CARTESIAN_POINT('Ctrl Pts',(3.09234774183542,4.1057529714019,9.68367736941564));
#10934=CARTESIAN_POINT('Ctrl Pts',(2.81844129077601,4.29712968250449,9.70159814533755));
#10935=CARTESIAN_POINT('Ctrl Pts',(2.69110238561239,4.37800196239046,9.70969152151099));
#10936=CARTESIAN_POINT('Ctrl Pts',(2.29712595106992,4.60452335805537,9.73434171391499));
#10937=CARTESIAN_POINT('Ctrl Pts',(2.02095459424152,4.73224738755845,9.75107592839753));
#10938=CARTESIAN_POINT('Ctrl Pts',(1.57232861944532,4.89325030892307,9.77711683769016));
#10939=CARTESIAN_POINT('Ctrl Pts',(1.40668495195599,4.94341535015533,9.78651271782279));
#10940=CARTESIAN_POINT('Ctrl Pts',(1.16054607375624,5.00458182317777,9.800214153655));
#10941=CARTESIAN_POINT('Ctrl Pts',(1.08182020652955,5.02218793258555,9.80455916285547));
#10942=CARTESIAN_POINT('Ctrl Pts',(0.890469366146186,5.06027295078329,9.8150497012534));
#10943=CARTESIAN_POINT('Ctrl Pts',(0.777511210125311,5.078855633468,9.82118374686248));
#10944=CARTESIAN_POINT('Ctrl Pts',(0.482940025866521,5.11725698742121,9.83711018054788));
#10945=CARTESIAN_POINT('Ctrl Pts',(0.300726894008224,5.13119001399218,9.84689106824658));
#10946=CARTESIAN_POINT('Ctrl Pts',(-0.0526382873010328,5.13932081579788,
9.86606281062832));
#10947=CARTESIAN_POINT('Ctrl Pts',(-0.223527398324413,5.13472716916811,
9.87542618281519));
#10948=CARTESIAN_POINT('Ctrl Pts',(-0.642936894665256,5.10247347976002,
9.89849249545521));
#10949=CARTESIAN_POINT('Ctrl Pts',(-0.890283390993074,5.06517558887105,
9.91215918905798));
#10950=CARTESIAN_POINT('Ctrl Pts',(-1.35225273499904,4.96061658693881,9.9378450687349));
#10951=CARTESIAN_POINT('Ctrl Pts',(-1.56710881927051,4.89698654769837,9.9498639791003));
#10952=CARTESIAN_POINT('Ctrl Pts',(-1.96905247810535,4.74877613486292,9.97283494715439));
#10953=CARTESIAN_POINT('Ctrl Pts',(-2.15657176427373,4.66660878841429,9.98377182860388));
#10954=CARTESIAN_POINT('Ctrl Pts',(-2.46858797968162,4.50705672920182,10.0027664384314));
#10955=CARTESIAN_POINT('Ctrl Pts',(-2.59559676521082,4.43512827049158,10.0107487027106));
#10956=CARTESIAN_POINT('Ctrl Pts',(-2.97150424125781,4.20055825525717,10.0350360557838));
#10957=CARTESIAN_POINT('Ctrl Pts',(-3.20951645387419,4.02163389510829,10.0513101009946));
#10958=CARTESIAN_POINT('Ctrl Pts',(-3.59483444624534,3.67586540971379,10.0793522664599));
#10959=CARTESIAN_POINT('Ctrl Pts',(-3.74929573901876,3.51818208393124,10.0911807423333));
#10960=CARTESIAN_POINT('Ctrl Pts',(-4.01554928564948,3.20885776302716,10.1130624072754));
#10961=CARTESIAN_POINT('Ctrl Pts',(-4.13006583069576,3.06005849625197,10.1231038241817));
#10962=CARTESIAN_POINT('Ctrl Pts',(-4.25500336145006,2.87789057874498,10.1350716196598));
#10963=CARTESIAN_POINT('Ctrl Pts',(-4.27355524320318,2.85026894655662,10.1368783130702));
#10964=CARTESIAN_POINT('Ctrl Pts',(-4.29183622628417,2.82247096871782,10.1386883748835));
#10965=CARTESIAN_POINT('',(-5.13674999921714,8.96808918659131E-5,8.07404150530312));
#10966=CARTESIAN_POINT('Ctrl Pts',(-4.29147790789737,2.82223516557546,9.66201704729489));
#10967=CARTESIAN_POINT('Ctrl Pts',(-4.03850873296674,3.20671998828925,9.63706766016189));
#10968=CARTESIAN_POINT('Ctrl Pts',(-3.16988399740047,4.20897597709122,9.56580344749316));
#10969=CARTESIAN_POINT('Ctrl Pts',(-1.17621811440022,5.22394435702451,9.44822440928873));
#10970=CARTESIAN_POINT('Ctrl Pts',(1.466419928428,5.15001905738628,9.30927993268152));
#10971=CARTESIAN_POINT('Ctrl Pts',(3.75162135492562,3.82078799558379,9.17033545607434));
#10972=CARTESIAN_POINT('Ctrl Pts',(5.12237336835931,1.56024830493584,9.03139097946715));
#10973=CARTESIAN_POINT('Ctrl Pts',(5.24455819522407,-1.0805984614274,8.89244650285997));
#10974=CARTESIAN_POINT('Ctrl Pts',(4.08839355403644,-3.45805174126212,8.75350202625278));
#10975=CARTESIAN_POINT('Ctrl Pts',(1.93569202061813,-4.99261255248659,8.61455754964559));
#10976=CARTESIAN_POINT('Ctrl Pts',(-0.688830164370685,-5.31023508920132,
8.4756130730384));
#10977=CARTESIAN_POINT('Ctrl Pts',(-3.14545151931376,-4.33349956012211,
8.33666859643121));
#10978=CARTESIAN_POINT('Ctrl Pts',(-4.7735013873256,-2.37491963879568,8.2028114111729));
#10979=CARTESIAN_POINT('Ctrl Pts',(-5.13643863329629,-0.760120718689461,
8.11526905145029));
#10980=CARTESIAN_POINT('Ctrl Pts',(-5.13705846939083,8.94657369160089E-5,
8.07404151726341));
#10981=CARTESIAN_POINT('Ctrl Pts',(-5.13674999921714,8.96808918659132E-5,
8.07404150530312));
#10982=CARTESIAN_POINT('Ctrl Pts',(-5.13674836157881,0.0938904733295929,
8.06895421794103));
#10983=CARTESIAN_POINT('Ctrl Pts',(-5.13417692765489,0.187682302088804,
8.06386693057893));
#10984=CARTESIAN_POINT('Ctrl Pts',(-5.12904010520378,0.28133283084496,8.05877964321683));
#10985=CARTESIAN_POINT('Ctrl Pts',(-5.1208932625175,0.42985969400276,8.05071136166081));
#10986=CARTESIAN_POINT('Ctrl Pts',(-5.10628901009753,0.578059904085605,
8.0426430801048));
#10987=CARTESIAN_POINT('Ctrl Pts',(-5.08527745830825,0.725364552843592,
8.0345747985488));
#10988=CARTESIAN_POINT('Ctrl Pts',(-5.06427014698131,0.872639473201553,
8.02650814529918));
#10989=CARTESIAN_POINT('Ctrl Pts',(-5.03685816275778,1.01901886531461,8.01844149204957));
#10990=CARTESIAN_POINT('Ctrl Pts',(-5.00314326900692,1.16394071682829,8.01037483879997));
#10991=CARTESIAN_POINT('Ctrl Pts',(-4.96942715985699,1.30886779267649,8.00230789475298));
#10992=CARTESIAN_POINT('Ctrl Pts',(-4.9294077578192,1.4523368995334,7.99424095070599));
#10993=CARTESIAN_POINT('Ctrl Pts',(-4.88323769496126,1.59379740776846,7.98617400665901));
#10994=CARTESIAN_POINT('Ctrl Pts',(-4.83707042499281,1.73524935886621,7.97810755059237));
#10995=CARTESIAN_POINT('Ctrl Pts',(-4.7847533420389,1.87469263998323,7.97004109452573));
#10996=CARTESIAN_POINT('Ctrl Pts',(-4.72648858792753,2.01159294855864,7.9619746384591));
#10997=CARTESIAN_POINT('Ctrl Pts',(-4.66820929321946,2.14852742208,7.9539061693215));
#10998=CARTESIAN_POINT('Ctrl Pts',(-4.60397949050707,2.28291734996498,7.94583770018391));
#10999=CARTESIAN_POINT('Ctrl Pts',(-4.53404927007515,2.414248905774,7.93776923104631));
#11000=CARTESIAN_POINT('Ctrl Pts',(-4.48223716636189,2.51155396427908,7.93179120956743));
#11001=CARTESIAN_POINT('Ctrl Pts',(-4.42729682191331,2.60718054062894,7.92581318808856));
#11002=CARTESIAN_POINT('Ctrl Pts',(-4.3693461565897,2.70092849338793,7.91983516660969));
#11003=CARTESIAN_POINT('Ctrl Pts',(-4.3440811633814,2.74180017926973,7.91722890365792));
#11004=CARTESIAN_POINT('Ctrl Pts',(-4.31824113528876,2.78231978684708,7.91462264070616));
#11005=CARTESIAN_POINT('Ctrl Pts',(-4.29183622825303,2.82247096572398,7.9120163777544));
#11006=CARTESIAN_POINT('Origin',(0.,0.,0.));
#11007=CARTESIAN_POINT('',(-4.29183649439966,2.8224705610226,6.16186016520308));
#11008=CARTESIAN_POINT('',(-4.29183621579633,2.82247098466558,6.63882185511496));
#11009=CARTESIAN_POINT('',(-4.29183622825304,2.82247096572397,0.));
#11010=CARTESIAN_POINT('',(-5.13675014872027,-9.28711217083157E-6,6.80070473863792));
#11011=CARTESIAN_POINT('Ctrl Pts',(-4.29183621579632,2.82247098466558,6.63882185511496));
#11012=CARTESIAN_POINT('Ctrl Pts',(-4.36054432246575,2.71799375810604,6.64553053324447));
#11013=CARTESIAN_POINT('Ctrl Pts',(-4.42542236198481,2.61103060857702,6.65224907493801));
#11014=CARTESIAN_POINT('Ctrl Pts',(-4.52854727960716,2.42610201637113,6.66371519269886));
#11015=CARTESIAN_POINT('Ctrl Pts',(-4.56883348544287,2.34935554169067,6.66843578009576));
#11016=CARTESIAN_POINT('Ctrl Pts',(-4.67535713383931,2.13331169675636,6.68159938307984));
#11017=CARTESIAN_POINT('Ctrl Pts',(-4.73729251546422,1.99199459944635,6.69006542486853));
#11018=CARTESIAN_POINT('Ctrl Pts',(-4.86290062692858,1.66624949149274,6.70919725108917));
#11019=CARTESIAN_POINT('Ctrl Pts',(-4.9226188023489,1.48054602995318,6.71983565717192));
#11020=CARTESIAN_POINT('Ctrl Pts',(-5.00997839377238,1.1443576750663,6.73866897165481));
#11021=CARTESIAN_POINT('Ctrl Pts',(-5.04173063842234,0.99518408487013,6.74688367030938));
#11022=CARTESIAN_POINT('Ctrl Pts',(-5.11335581407559,0.565611415626293,
6.77028080514691));
#11023=CARTESIAN_POINT('Ctrl Pts',(-5.13675051331794,0.283040576761006,
6.78534315712252));
#11024=CARTESIAN_POINT('Ctrl Pts',(-5.13674999999155,-9.31577570951679E-6,
6.80070448240941));
#11025=CARTESIAN_POINT('Ctrl Pts',(-5.13674999999158,-9.30106097508931E-6,
6.80070448161083));
#11026=CARTESIAN_POINT('Ctrl Pts',(-5.13674950345215,-0.27423596180585,
6.81558696362695));
#11027=CARTESIAN_POINT('Ctrl Pts',(-5.11478964040234,-0.548021090301936,
6.83068431061558));
#11028=CARTESIAN_POINT('Ctrl Pts',(-5.04678958992111,-0.969196820943226,
6.85402175161803));
#11029=CARTESIAN_POINT('Ctrl Pts',(-5.01581385299244,-1.11849915175892,
6.86232311664869));
#11030=CARTESIAN_POINT('Ctrl Pts',(-4.93217527169861,-1.44733483946227,
6.88071042563993));
#11031=CARTESIAN_POINT('Ctrl Pts',(-4.87625374014481,-1.62581745964357,
6.89075940774323));
#11032=CARTESIAN_POINT('Ctrl Pts',(-4.75471855226032,-1.95048110662605,
6.90935726438368));
#11033=CARTESIAN_POINT('Ctrl Pts',(-4.69175846614595,-2.09740958552241,
6.91790335404333));
#11034=CARTESIAN_POINT('Ctrl Pts',(-4.58659378739211,-2.31429550917129,
6.93087454579517));
#11035=CARTESIAN_POINT('Ctrl Pts',(-4.54940313229822,-2.3865743567122,6.93526035462519));
#11036=CARTESIAN_POINT('Ctrl Pts',(-4.4086137130355,-2.64493403091877,6.9512287255878));
#11037=CARTESIAN_POINT('Ctrl Pts',(-4.29518531803503,-2.82540829394662,
6.96292550732711));
#11038=CARTESIAN_POINT('Ctrl Pts',(-4.07791257783295,-3.12765094233414,
6.98332890063532));
#11039=CARTESIAN_POINT('Ctrl Pts',(-3.97897322645356,-3.25259046098966,
6.9920375634287));
#11040=CARTESIAN_POINT('Ctrl Pts',(-3.76110983985535,-3.50285857226653,
7.01008565733192));
#11041=CARTESIAN_POINT('Ctrl Pts',(-3.64134660308096,-3.62719756988625,
7.01940526766324));
#11042=CARTESIAN_POINT('Ctrl Pts',(-3.29319917853703,-3.95399069951888,
7.04508999435205));
#11043=CARTESIAN_POINT('Ctrl Pts',(-3.05270619465187,-4.14248481942735,
7.0612956912011));
#11044=CARTESIAN_POINT('Ctrl Pts',(-2.66938000634769,-4.3913248169919,7.08608277178135));
#11045=CARTESIAN_POINT('Ctrl Pts',(-2.53822428951772,-4.46841575447014,
7.09440807688176));
#11046=CARTESIAN_POINT('Ctrl Pts',(-2.24217403483129,-4.62518352009839,
7.11277421305259));
#11047=CARTESIAN_POINT('Ctrl Pts',(-2.07604374735069,-4.70209640571389,
7.12280514878522));
#11048=CARTESIAN_POINT('Ctrl Pts',(-1.83446541981166,-4.79863510057314,
7.13699356723012));
#11049=CARTESIAN_POINT('Ctrl Pts',(-1.76212929828872,-4.82566707517999,
7.14119411453483));
#11050=CARTESIAN_POINT('Ctrl Pts',(-1.39095217583523,-4.95491648113349,
7.16252117329537));
#11051=CARTESIAN_POINT('Ctrl Pts',(-1.08374941351432,-5.03104724260106,
7.17938545784351));
#11052=CARTESIAN_POINT('Ctrl Pts',(-0.637978411693939,-5.09876691955784,
7.20358407265057));
#11053=CARTESIAN_POINT('Ctrl Pts',(-0.503709634645125,-5.11377710239055,
7.21084638396267));
#11054=CARTESIAN_POINT('Ctrl Pts',(-0.180344330600151,-5.13706672041347,
7.22845003050856));
#11055=CARTESIAN_POINT('Ctrl Pts',(0.00892203440674387,-5.1402234677049,
7.23882968510254));
#11056=CARTESIAN_POINT('Ctrl Pts',(0.417628408824725,-5.12446359669769,
7.26125584076046));
#11057=CARTESIAN_POINT('Ctrl Pts',(0.636562282602356,-5.10189499334267,
7.27327272826308));
#11058=CARTESIAN_POINT('Ctrl Pts',(1.14514014747377,-5.01621327712766,7.30124785130825));
#11059=CARTESIAN_POINT('Ctrl Pts',(1.4321114669278,-4.94194316041895,7.3170641337704));
#11060=CARTESIAN_POINT('Ctrl Pts',(1.84945646942886,-4.7945015518509,7.34080839480143));
#11061=CARTESIAN_POINT('Ctrl Pts',(1.98565890163175,-4.73971432203543,7.34869052454216));
#11062=CARTESIAN_POINT('Ctrl Pts',(2.30675754579164,-4.59427981672183,7.36782354348952));
#11063=CARTESIAN_POINT('Ctrl Pts',(2.48891569475288,-4.49820343995965,7.37912180059713));
#11064=CARTESIAN_POINT('Ctrl Pts',(2.85545396747633,-4.27578152793372,7.40262550403596));
#11065=CARTESIAN_POINT('Ctrl Pts',(3.03835895787385,-4.14780708862957,7.41480043167686));
#11066=CARTESIAN_POINT('Ctrl Pts',(3.41066832135115,-3.84943105993617,7.44065023755202));
#11067=CARTESIAN_POINT('Ctrl Pts',(3.5969012665231,-3.67601444936041,7.45425755686874));
#11068=CARTESIAN_POINT('Ctrl Pts',(3.88120336409985,-3.36889917276742,7.47669736174359));
#11069=CARTESIAN_POINT('Ctrl Pts',(3.98701407184942,-3.24298289477458,7.48551136401496));
#11070=CARTESIAN_POINT('Ctrl Pts',(4.20211610597592,-2.96053545335588,7.50476328492376));
#11071=CARTESIAN_POINT('Ctrl Pts',(4.30909291233613,-2.80254634427599,7.51522171498177));
#11072=CARTESIAN_POINT('Ctrl Pts',(4.52076144299933,-2.4490646034915,7.53781399444568));
#11073=CARTESIAN_POINT('Ctrl Pts',(4.62209166797824,-2.25199321670785,7.54991916621719));
#11074=CARTESIAN_POINT('Ctrl Pts',(4.83862930088939,-1.75419992452382,7.579379020834));
#11075=CARTESIAN_POINT('Ctrl Pts',(4.93890802903207,-1.44801318948668,7.59654013623497));
#11076=CARTESIAN_POINT('Ctrl Pts',(5.03908604070774,-1.00561689752975,7.62088785368799));
#11077=CARTESIAN_POINT('Ctrl Pts',(5.06328068884328,-0.875694757219264,
7.62799393891609));
#11078=CARTESIAN_POINT('Ctrl Pts',(5.10921062119309,-0.562351432419921,
7.64519180436847));
#11079=CARTESIAN_POINT('Ctrl Pts',(5.12611713371375,-0.37840961972383,7.65531921411957));
#11080=CARTESIAN_POINT('Ctrl Pts',(5.14130917804655,0.0236422561292717,
7.67738033787116));
#11081=CARTESIAN_POINT('Ctrl Pts',(5.13568644781166,0.241551216386984,7.68928568880778));
#11082=CARTESIAN_POINT('Ctrl Pts',(5.08795681011533,0.774211612571511,7.71830557852863));
#11083=CARTESIAN_POINT('Ctrl Pts',(5.03049090999706,1.08667988858655,7.73523311872986));
#11084=CARTESIAN_POINT('Ctrl Pts',(4.9182480240667,1.48542448513362,7.75746574893529));
#11085=CARTESIAN_POINT('Ctrl Pts',(4.88925868754023,1.57822641515211,7.76269079107157));
#11086=CARTESIAN_POINT('Ctrl Pts',(4.82378547465927,1.76865629021999,7.77357480614793));
#11087=CARTESIAN_POINT('Ctrl Pts',(4.78692917595042,1.86610809546057,7.77924340018738));
#11088=CARTESIAN_POINT('Ctrl Pts',(4.62425516613131,2.2596300912493,7.80251582822976));
#11089=CARTESIAN_POINT('Ctrl Pts',(4.47372032211606,2.54469994475272,7.82019763137673));
#11090=CARTESIAN_POINT('Ctrl Pts',(4.19690789804165,2.96747326399253,7.84764644609172));
#11091=CARTESIAN_POINT('Ctrl Pts',(4.08812953926978,3.11562713685656,7.8575471454494));
#11092=CARTESIAN_POINT('Ctrl Pts',(3.82404402320297,3.43759499336962,7.8799145038888));
#11093=CARTESIAN_POINT('Ctrl Pts',(3.66438115743665,3.6073092984431,7.89232976661486));
#11094=CARTESIAN_POINT('Ctrl Pts',(3.46445092934173,3.79280625070061,7.90705158945612));
#11095=CARTESIAN_POINT('Ctrl Pts',(3.43482142564496,3.8196598313788,7.90921427837658));
#11096=CARTESIAN_POINT('Ctrl Pts',(3.26450702536935,3.97043350904541,7.92155006128397));
#11097=CARTESIAN_POINT('Ctrl Pts',(3.11743648472242,4.08692256940132,7.93183294366476));
#11098=CARTESIAN_POINT('Ctrl Pts',(2.78054770698615,4.32497351435593,7.95445273793627));
#11099=CARTESIAN_POINT('Ctrl Pts',(2.5884261283377,4.44262255558441,7.96675956819401));
#11100=CARTESIAN_POINT('Ctrl Pts',(2.10820033422106,4.69493937488908,7.9961965505212));
#11101=CARTESIAN_POINT('Ctrl Pts',(1.81411126625045,4.81621932101812,8.01314528483233));
#11102=CARTESIAN_POINT('Ctrl Pts',(1.38244396156637,4.94904631125324,8.03738545033428));
#11103=CARTESIAN_POINT('Ctrl Pts',(1.25268244173541,4.98347233519436,8.04460249167849));
#11104=CARTESIAN_POINT('Ctrl Pts',(0.938400275493735,5.05380009908791,8.06209008455252));
#11105=CARTESIAN_POINT('Ctrl Pts',(0.752967681060348,5.08473485470611,8.07239820350146));
#11106=CARTESIAN_POINT('Ctrl Pts',(0.347051752675588,5.12975626699935,8.0947914169983));
#11107=CARTESIAN_POINT('Ctrl Pts',(0.126500503417814,5.13992658941099,8.10684658735286));
#11108=CARTESIAN_POINT('Ctrl Pts',(-0.391286155929265,5.13044738554987,
8.13493782728548));
#11109=CARTESIAN_POINT('Ctrl Pts',(-0.687516963178789,5.09920773431871,
8.1508297683649));
#11110=CARTESIAN_POINT('Ctrl Pts',(-1.1225351821779,5.01471647054983,8.17460282635074));
#11111=CARTESIAN_POINT('Ctrl Pts',(-1.26443690610858,4.98082971179623,8.18243641530185));
#11112=CARTESIAN_POINT('Ctrl Pts',(-1.6013561040864,4.88504425765085,8.20144892022648));
#11113=CARTESIAN_POINT('Ctrl Pts',(-1.7944939123785,4.81744626305338,8.21267449240564));
#11114=CARTESIAN_POINT('Ctrl Pts',(-2.18963931515588,4.65207662813501,8.23615723463917));
#11115=CARTESIAN_POINT('Ctrl Pts',(-2.39032342437481,4.55221869165,8.24838315455969));
#11116=CARTESIAN_POINT('Ctrl Pts',(-2.79869236062219,4.31454651966576,8.27398290723136));
#11117=CARTESIAN_POINT('Ctrl Pts',(-3.00417370239928,4.17407881933512,8.28729817806015));
#11118=CARTESIAN_POINT('Ctrl Pts',(-3.32947334607747,3.91519475790035,8.30958846485193));
#11119=CARTESIAN_POINT('Ctrl Pts',(-3.45510707732345,3.80478329143979,8.31854826171555));
#11120=CARTESIAN_POINT('Ctrl Pts',(-3.74476813162638,3.52402104508847,8.3404146004508));
#11121=CARTESIAN_POINT('Ctrl Pts',(-3.90285678186919,3.34809175122058,8.35340004403069));
#11122=CARTESIAN_POINT('Ctrl Pts',(-4.13404672687069,3.05209360572302,8.3739803016593));
#11123=CARTESIAN_POINT('Ctrl Pts',(-4.21529978690164,2.93885191876446,8.38159494541361));
#11124=CARTESIAN_POINT('Ctrl Pts',(-4.2918361854396,2.82247103082588,8.38917442239304));
#11125=CARTESIAN_POINT('',(-5.13674999998633,-1.18511375680025E-5,6.32404150530312));
#11126=CARTESIAN_POINT('Ctrl Pts',(-4.29183622825303,2.82247096572398,7.9120163777544));
#11127=CARTESIAN_POINT('Ctrl Pts',(-4.21009995288661,2.946758766038,7.90394870207524));
#11128=CARTESIAN_POINT('Ctrl Pts',(-4.12294775268111,3.06751403657549,7.89588102639609));
#11129=CARTESIAN_POINT('Ctrl Pts',(-4.0307097059894,3.18427069021194,7.88781335071693));
#11130=CARTESIAN_POINT('Ctrl Pts',(-3.938487576668,3.3010071953418,7.8797470672635));
#11131=CARTESIAN_POINT('Ctrl Pts',(-3.8411815570887,3.41374620077307,7.87168078381006));
#11132=CARTESIAN_POINT('Ctrl Pts',(-3.73916284912825,3.52205362682045,7.86361450035663));
#11133=CARTESIAN_POINT('Ctrl Pts',(-3.63713879186065,3.63036673192122,7.85554779395108));
#11134=CARTESIAN_POINT('Ctrl Pts',(-3.53040177689899,3.73424755003897,7.84748108754553));
#11135=CARTESIAN_POINT('Ctrl Pts',(-3.41936117223181,3.83329750167313,7.83941438113999));
#11136=CARTESIAN_POINT('Ctrl Pts',(-3.30832402994983,3.93234436480569,7.83134792626445));
#11137=CARTESIAN_POINT('Ctrl Pts',(-3.19298381480945,4.02656044402617,7.82328147138892));
#11138=CARTESIAN_POINT('Ctrl Pts',(-3.07378440728717,4.11558622555988,7.81521501651338));
#11139=CARTESIAN_POINT('Ctrl Pts',(-2.95455811294958,4.20463208789598,7.80714674215496));
#11140=CARTESIAN_POINT('Ctrl Pts',(-2.83147115284758,4.28848511611201,7.79907846779654));
#11141=CARTESIAN_POINT('Ctrl Pts',(-2.70499840189602,4.36682770535316,7.79101019343812));
#11142=CARTESIAN_POINT('Ctrl Pts',(-2.65212293018557,4.39958101648127,7.78763702562623));
#11143=CARTESIAN_POINT('Ctrl Pts',(-2.59865600441084,4.43137168571285,7.78426385781434));
#11144=CARTESIAN_POINT('Ctrl Pts',(-2.54463373986122,4.46217880552314,7.78089069000245));
#11145=CARTESIAN_POINT('Ctrl Pts',(-2.41541786179681,4.53586636879189,7.77282240844658));
#11146=CARTESIAN_POINT('Ctrl Pts',(-2.28297517347506,4.60395102761205,7.76475412689072));
#11147=CARTESIAN_POINT('Ctrl Pts',(-2.14781086612749,4.66616641857582,7.75668584533485));
#11148=CARTESIAN_POINT('Ctrl Pts',(-2.01267383706738,4.72836925349316,7.74861919208537));
#11149=CARTESIAN_POINT('Ctrl Pts',(-1.87481658528843,4.78470504536419,7.74055253883589));
#11150=CARTESIAN_POINT('Ctrl Pts',(-1.73476651462124,4.83495457085678,7.7324858855864));
#11151=CARTESIAN_POINT('Ctrl Pts',(-1.59471139524434,4.88520590781056,7.72441894153956));
#11152=CARTESIAN_POINT('Ctrl Pts',(-1.45246360907001,4.92937042399138,7.71635199749271));
#11153=CARTESIAN_POINT('Ctrl Pts',(-1.30856857724477,4.96727780994254,7.70828505344587));
#11154=CARTESIAN_POINT('Ctrl Pts',(-1.16468224982467,5.00518290282465,7.70021859737939));
#11155=CARTESIAN_POINT('Ctrl Pts',(-1.01914919641765,5.03683153917223,7.69215214131291));
#11156=CARTESIAN_POINT('Ctrl Pts',(-0.87252796420602,5.06210386244479,7.68408568524642));
#11157=CARTESIAN_POINT('Ctrl Pts',(-0.725870141087082,5.08738249269776,
7.67601721610897));
#11158=CARTESIAN_POINT('Ctrl Pts',(-0.578123922775169,5.10628157328747,
7.66794874697151));
#11159=CARTESIAN_POINT('Ctrl Pts',(-0.429856649723374,5.11873263837726,
7.65988027783406));
#11160=CARTESIAN_POINT('Ctrl Pts',(-0.320003723731571,5.12795777554795,
7.65390225635447));
#11161=CARTESIAN_POINT('Ctrl Pts',(-0.209864963383611,5.1336443408075,7.64792423487488));
#11162=CARTESIAN_POINT('Ctrl Pts',(-0.099672473439093,5.13578289655419,
7.64194621339529));
#11163=CARTESIAN_POINT('Ctrl Pts',(0.0490496476247377,5.13866921436787,
7.63387793183946));
#11164=CARTESIAN_POINT('Ctrl Pts',(0.197924721660986,5.13509167512214,7.62580965028363));
#11165=CARTESIAN_POINT('Ctrl Pts',(0.346381691016817,5.12505807641517,7.61774136872781));
#11166=CARTESIAN_POINT('Ctrl Pts',(0.494808699416362,5.11502650264655,7.60967471547836));
#11167=CARTESIAN_POINT('Ctrl Pts',(0.642817441416092,5.09854149111461,7.60160806222892));
#11168=CARTESIAN_POINT('Ctrl Pts',(0.789839907090891,5.07566286150554,7.59354140897947));
#11169=CARTESIAN_POINT('Ctrl Pts',(0.936867672825632,5.05278340713744,7.58547446493266));
#11170=CARTESIAN_POINT('Ctrl Pts',(1.08290876344197,5.02350992062861,7.57740752088585));
#11171=CARTESIAN_POINT('Ctrl Pts',(1.22740274936792,4.98795379422706,7.56934057683904));
#11172=CARTESIAN_POINT('Ctrl Pts',(1.3718879946571,4.95239981866371,7.56127412077259));
#11173=CARTESIAN_POINT('Ctrl Pts',(1.51482600124082,4.91056404341939,7.55320766470614));
#11174=CARTESIAN_POINT('Ctrl Pts',(1.65566895138303,4.86260844464431,7.54514120863969));
#11175=CARTESIAN_POINT('Ctrl Pts',(1.79654705040012,4.81464087803316,7.53707273950227));
#11176=CARTESIAN_POINT('Ctrl Pts',(1.9353287345135,4.76055054223209,7.52900427036485));
#11177=CARTESIAN_POINT('Ctrl Pts',(2.07148305120219,4.70054874786785,7.52093580122742));
#11178=CARTESIAN_POINT('Ctrl Pts',(2.17236134866681,4.65609272908348,7.51495777974765));
#11179=CARTESIAN_POINT('Ctrl Pts',(2.27179768844976,4.60839264641327,7.50897975826787));
#11180=CARTESIAN_POINT('Ctrl Pts',(2.36958373807782,4.55755125815795,7.5030017367881));
#11181=CARTESIAN_POINT('Ctrl Pts',(2.50156141385262,4.48893279692935,7.49493345523226));
#11182=CARTESIAN_POINT('Ctrl Pts',(2.63058090336597,4.41456507690165,7.48686517367642));
#11183=CARTESIAN_POINT('Ctrl Pts',(2.75614447658439,4.33472815603163,7.47879689212058));
#11184=CARTESIAN_POINT('Ctrl Pts',(2.88168270909485,4.25490734751047,7.47073023887112));
#11185=CARTESIAN_POINT('Ctrl Pts',(3.0037661375973,4.16961971769966,7.46266358562165));
#11186=CARTESIAN_POINT('Ctrl Pts',(3.12192459723588,4.07918954838747,7.45459693237219));
#11187=CARTESIAN_POINT('Ctrl Pts',(3.24008731640648,3.98875611912925,7.44652998832537));
#11188=CARTESIAN_POINT('Ctrl Pts',(3.35432451842213,3.89317997756405,7.43846304427855));
#11189=CARTESIAN_POINT('Ctrl Pts',(3.46419736875478,3.79282706603035,7.43039610023173));
#11190=CARTESIAN_POINT('Ctrl Pts',(3.57406357272995,3.69248022498015,7.42232964416527));
#11191=CARTESIAN_POINT('Ctrl Pts',(3.67956570932188,3.58735741589004,7.41426318809882));
#11192=CARTESIAN_POINT('Ctrl Pts',(3.78030021960309,3.47786296627237,7.40619673203236));
#11193=CARTESIAN_POINT('Ctrl Pts',(3.88105986926614,3.36834119113567,7.39812826289493));
#11194=CARTESIAN_POINT('Ctrl Pts',(3.97704929042786,3.25444583873924,7.3900597937575));
#11195=CARTESIAN_POINT('Ctrl Pts',(4.06790333700283,3.13661648967501,7.38199132462007));
#11196=CARTESIAN_POINT('Ctrl Pts',(4.13521814390037,3.04931537125343,7.37601330314035));
#11197=CARTESIAN_POINT('Ctrl Pts',(4.1997146750762,2.95985543037342,7.37003528166063));
#11198=CARTESIAN_POINT('Ctrl Pts',(4.26125915092337,2.86842657412943,7.3640572601809));
#11199=CARTESIAN_POINT('Ctrl Pts',(4.34432311464882,2.7450289321157,7.35598897862506));
#11200=CARTESIAN_POINT('Ctrl Pts',(4.42203880424172,2.6179979986879,7.34792069706922));
#11201=CARTESIAN_POINT('Ctrl Pts',(4.49410313788345,2.48781782865349,7.33985241551337));
#11202=CARTESIAN_POINT('Ctrl Pts',(4.56615292780693,2.35766393102898,7.3317857622639));
#11203=CARTESIAN_POINT('Ctrl Pts',(4.63255347695501,2.22436235419458,7.32371910901443));
#11204=CARTESIAN_POINT('Ctrl Pts',(4.6930470671855,2.08842279907149,7.31565245576496));
#11205=CARTESIAN_POINT('Ctrl Pts',(4.75354283816872,1.95247834341999,7.30758551171813));
#11206=CARTESIAN_POINT('Ctrl Pts',(4.80813108609039,1.81389602005319,7.2995185676713));
#11207=CARTESIAN_POINT('Ctrl Pts',(4.85660153641266,1.67320712376387,7.29145162362447));
#11208=CARTESIAN_POINT('Ctrl Pts',(4.90506905469177,1.53252673793637,7.28338516755801));
#11209=CARTESIAN_POINT('Ctrl Pts',(4.94741940868861,1.38974034736346,7.27531871149155));
#11210=CARTESIAN_POINT('Ctrl Pts',(4.9834916648809,1.24539607698216,7.26725225542509));
#11211=CARTESIAN_POINT('Ctrl Pts',(5.01957292329318,1.10101578393377,7.25918378628765));
#11212=CARTESIAN_POINT('Ctrl Pts',(5.04937287226009,0.955077155346015,7.25111531715021));
#11213=CARTESIAN_POINT('Ctrl Pts',(5.07278117568299,0.808140894978314,7.24304684801278));
#11214=CARTESIAN_POINT('Ctrl Pts',(5.09012465661863,0.699274131573728,7.23706882653309));
#11215=CARTESIAN_POINT('Ctrl Pts',(5.10396049227048,0.589859995340661,7.23109080505341));
#11216=CARTESIAN_POINT('Ctrl Pts',(5.11426206438136,0.480129252732794,7.22511278357372));
#11217=CARTESIAN_POINT('Ctrl Pts',(5.12816565849535,0.3320303324295,7.21704450201789));
#11218=CARTESIAN_POINT('Ctrl Pts',(5.13563452060422,0.183299694848691,7.20897622046205));
#11219=CARTESIAN_POINT('Ctrl Pts',(5.13663409262762,0.0345074043590885,
7.20090793890621));
#11220=CARTESIAN_POINT('Ctrl Pts',(5.13763346292164,-0.114254857501211,
7.19284128565676));
#11221=CARTESIAN_POINT('Ctrl Pts',(5.13216614562539,-0.263078416641545,
7.1847746324073));
#11222=CARTESIAN_POINT('Ctrl Pts',(5.12024968753788,-0.411392391480728,
7.17670797915785));
#11223=CARTESIAN_POINT('Ctrl Pts',(5.10833279987017,-0.559711712937808,
7.16864103511103));
#11224=CARTESIAN_POINT('Ctrl Pts',(5.08996632892319,-0.707521083093384,
7.16057409106421));
#11225=CARTESIAN_POINT('Ctrl Pts',(5.06521981410316,-0.854253356631802,
7.15250714701739));
#11226=CARTESIAN_POINT('Ctrl Pts',(5.04047479623331,-1.00097675413638,7.14444069095094));
#11227=CARTESIAN_POINT('Ctrl Pts',(5.00935056245525,-1.14662285909008,7.13637423488449));
#11228=CARTESIAN_POINT('Ctrl Pts',(4.97196803184221,-1.29063335337309,7.12830777881803));
#11229=CARTESIAN_POINT('Ctrl Pts',(4.93457617201611,-1.43467978702572,7.1202393096806));
#11230=CARTESIAN_POINT('Ctrl Pts',(4.89092297709436,-1.57708947365403,7.11217084054318));
#11231=CARTESIAN_POINT('Ctrl Pts',(4.84117981514528,-1.71731725663313,7.10410237140575));
#11232=CARTESIAN_POINT('Ctrl Pts',(4.80432453497542,-1.82121363207028,7.09812434992601));
#11233=CARTESIAN_POINT('Ctrl Pts',(4.76412722074456,-1.92391250978888,7.09214632844627));
#11234=CARTESIAN_POINT('Ctrl Pts',(4.72067490368666,-2.02519851278904,7.08616830696653));
#11235=CARTESIAN_POINT('Ctrl Pts',(4.66202915785498,-2.16189992690095,7.07810002541068));
#11236=CARTESIAN_POINT('Ctrl Pts',(4.59743067384917,-2.2960775044637,7.07003174385483));
#11237=CARTESIAN_POINT('Ctrl Pts',(4.52712184078284,-2.42721412347716,7.06196346229899));
#11238=CARTESIAN_POINT('Ctrl Pts',(4.45682719714717,-2.55832427705406,7.05389680904952));
#11239=CARTESIAN_POINT('Ctrl Pts',(4.38082465991316,-2.6863944049046,7.04583015580006));
#11240=CARTESIAN_POINT('Ctrl Pts',(4.29940276382755,-2.81093159591122,7.0377635025506));
#11241=CARTESIAN_POINT('Ctrl Pts',(4.21797793253794,-2.93547327639891,7.02969655850377));
#11242=CARTESIAN_POINT('Ctrl Pts',(4.13113352942016,-3.05648148607089,7.02162961445694));
#11243=CARTESIAN_POINT('Ctrl Pts',(4.03920195774788,-3.17349146950574,7.01356267041011));
#11244=CARTESIAN_POINT('Ctrl Pts',(3.94727594714088,-3.29049437484822,7.00549621434365));
#11245=CARTESIAN_POINT('Ctrl Pts',(3.85026358877736,-3.40349927802166,6.99742975827719));
#11246=CARTESIAN_POINT('Ctrl Pts',(3.74853818056925,-3.51207375653112,6.98936330221073));
#11247=CARTESIAN_POINT('Ctrl Pts',(3.64678738569001,-3.62067533097094,6.98129483307329));
#11248=CARTESIAN_POINT('Ctrl Pts',(3.54032141665499,-3.72484402929224,6.97322636393585));
#11249=CARTESIAN_POINT('Ctrl Pts',(3.42955157511154,-3.82418312272699,6.9651578947984));
#11250=CARTESIAN_POINT('Ctrl Pts',(3.34748092691687,-3.89778459832415,6.95917987331872));
#11251=CARTESIAN_POINT('Ctrl Pts',(3.2630484692996,-3.96873559307783,6.95320185183903));
#11252=CARTESIAN_POINT('Ctrl Pts',(3.17643366931386,-4.03688861710962,6.94722383035934));
#11253=CARTESIAN_POINT('Ctrl Pts',(3.05953335445872,-4.12887185749071,6.93915554880351));
#11254=CARTESIAN_POINT('Ctrl Pts',(2.93861326203309,-4.21579088707642,6.93108726724769));
#11255=CARTESIAN_POINT('Ctrl Pts',(2.81413364653386,-4.29730757357977,6.92301898569186));
#11256=CARTESIAN_POINT('Ctrl Pts',(2.68967915298276,-4.37880780873113,6.91495233244241));
#11257=CARTESIAN_POINT('Ctrl Pts',(2.56166684627373,-4.4549076947012,6.90688567919295));
#11258=CARTESIAN_POINT('Ctrl Pts',(2.43058591939444,-4.52531243683146,6.89881902594349));
#11259=CARTESIAN_POINT('Ctrl Pts',(2.29950026713706,-4.5957197170047,6.89075208189668));
#11260=CARTESIAN_POINT('Ctrl Pts',(2.16534606315687,-4.66043128254934,6.88268513784987));
#11261=CARTESIAN_POINT('Ctrl Pts',(2.02863755203179,-4.71919805104495,6.87461819380306));
#11262=CARTESIAN_POINT('Ctrl Pts',(1.8919373105896,-4.77796126465919,6.86655173773661));
#11263=CARTESIAN_POINT('Ctrl Pts',(1.75268337556592,-4.83078027067817,6.85848528167017));
#11264=CARTESIAN_POINT('Ctrl Pts',(1.61141043317042,-4.87745394425919,6.85041882560372));
#11265=CARTESIAN_POINT('Ctrl Pts',(1.47010223459086,-4.92413926575805,6.8423503564663));
#11266=CARTESIAN_POINT('Ctrl Pts',(1.32677433607392,-4.96467608580011,6.83428188732888));
#11267=CARTESIAN_POINT('Ctrl Pts',(1.1819777189786,-4.99891280523457,6.82621341819146));
#11268=CARTESIAN_POINT('Ctrl Pts',(1.07469624185444,-5.02427918399739,6.8202353967117));
#11269=CARTESIAN_POINT('Ctrl Pts',(0.966608865772434,-5.04618814763894,
6.81425737523193));
#11270=CARTESIAN_POINT('Ctrl Pts',(0.857943748909188,-5.06459604373415,
6.80827935375217));
#11271=CARTESIAN_POINT('Ctrl Pts',(0.711283058391623,-5.08944039885225,
6.80021107219632));
#11272=CARTESIAN_POINT('Ctrl Pts',(0.563515362805088,-5.10791455911667,
6.79214279064048));
#11273=CARTESIAN_POINT('Ctrl Pts',(0.415206596013435,-5.11994180095115,
6.78407450908464));
#11274=CARTESIAN_POINT('Ctrl Pts',(0.26692776026831,-5.13196661549868,6.77600785583518));
#11275=CARTESIAN_POINT('Ctrl Pts',(0.118108400899065,-5.13754708058652,
6.76794120258571));
#11276=CARTESIAN_POINT('Ctrl Pts',(-0.0306808705751501,-5.13665837356162,
6.75987454933624));
#11277=CARTESIAN_POINT('Ctrl Pts',(-0.179475505801333,-5.13576963449945,
6.75180760528942));
#11278=CARTESIAN_POINT('Ctrl Pts',(-0.328239719944949,-5.12841125484726,
6.74374066124259));
#11279=CARTESIAN_POINT('Ctrl Pts',(-0.476402773103094,-5.11461053847502,
6.73567371719577));
#11280=CARTESIAN_POINT('Ctrl Pts',(-0.62455686367748,-5.1008106569268,6.72760726112931));
#11281=CARTESIAN_POINT('Ctrl Pts',(-0.772109536492282,-5.08056924981998,
6.71954080506286));
#11282=CARTESIAN_POINT('Ctrl Pts',(-0.91849504562186,-5.05396551369992,
6.71147434899641));
#11283=CARTESIAN_POINT('Ctrl Pts',(-1.06491708683173,-5.02735513833101,
6.70340587985897));
#11284=CARTESIAN_POINT('Ctrl Pts',(-1.21017105636499,-4.99437931980706,
6.69533741072153));
#11285=CARTESIAN_POINT('Ctrl Pts',(-1.35370059363943,-4.95516854055241,
6.6872689415841));
#11286=CARTESIAN_POINT('Ctrl Pts',(-1.46004327676605,-4.92611682372389,
6.68129092010439));
#11287=CARTESIAN_POINT('Ctrl Pts',(-1.565439512296,-4.89364349479034,6.67531289862468));
#11288=CARTESIAN_POINT('Ctrl Pts',(-1.66966806398151,-4.85781937896215,
6.66933487714497));
#11289=CARTESIAN_POINT('Ctrl Pts',(-1.81034091101133,-4.80946909217047,
6.66126659558913));
#11290=CARTESIAN_POINT('Ctrl Pts',(-1.94893816056983,-4.75499534738238,
6.65319831403329));
#11291=CARTESIAN_POINT('Ctrl Pts',(-2.08492614455465,-4.69460153093449,
6.64513003247745));
#11292=CARTESIAN_POINT('Ctrl Pts',(-2.22088668402104,-4.63421990291061,
6.63706337922799));
#11293=CARTESIAN_POINT('Ctrl Pts',(-2.35423870613906,-4.56792072108554,
6.62899672597853));
#11294=CARTESIAN_POINT('Ctrl Pts',(-2.48446926615469,-4.49595518527851,
6.62093007272907));
#11295=CARTESIAN_POINT('Ctrl Pts',(-2.61470452089347,-4.42398705516285,
6.61286312868224));
#11296=CARTESIAN_POINT('Ctrl Pts',(-2.74181779681594,-4.34635231908976,
6.60479618463541));
#11297=CARTESIAN_POINT('Ctrl Pts',(-2.86532097528403,-4.26334801196165,
6.59672924058859));
#11298=CARTESIAN_POINT('Ctrl Pts',(-2.98881668287759,-4.1803487258765,6.58866278452213));
#11299=CARTESIAN_POINT('Ctrl Pts',(-3.10870245562007,-4.09198070388662,
6.58059632845568));
#11300=CARTESIAN_POINT('Ctrl Pts',(-3.22451938718877,-3.99858415994258,
6.57252987238922));
#11301=CARTESIAN_POINT('Ctrl Pts',(-3.34036522212005,-3.90516430788517,
6.56446140325178));
#11302=CARTESIAN_POINT('Ctrl Pts',(-3.4521399286501,-3.80671363367402,6.55639293411435));
#11303=CARTESIAN_POINT('Ctrl Pts',(-3.5594173786357,-3.70361289650608,6.54832446497691));
#11304=CARTESIAN_POINT('Ctrl Pts',(-3.6389004738026,-3.62722437585056,6.5423464434972));
#11305=CARTESIAN_POINT('Ctrl Pts',(-3.71591546932809,-3.548284056494,6.53636842201749));
#11306=CARTESIAN_POINT('Ctrl Pts',(-3.79030197673961,-3.46695997779378,
6.53039040053778));
#11307=CARTESIAN_POINT('Ctrl Pts',(-3.89069828474704,-3.35720032462925,
6.52232211898194));
#11308=CARTESIAN_POINT('Ctrl Pts',(-3.98634231503882,-3.24305652967757,
6.5142538374261));
#11309=CARTESIAN_POINT('Ctrl Pts',(-4.07686274569445,-3.12496251421817,
6.50618555587026));
#11310=CARTESIAN_POINT('Ctrl Pts',(-4.16736490790042,-3.00689233199244,
6.4981189026208));
#11311=CARTESIAN_POINT('Ctrl Pts',(-4.25274533212363,-2.88487378228349,
6.49005224937135));
#11312=CARTESIAN_POINT('Ctrl Pts',(-4.33267376952517,-2.75937285798214,
6.4819855961219));
#11313=CARTESIAN_POINT('Ctrl Pts',(-4.41260508829257,-2.63386740945775,
6.47391865207507));
#11314=CARTESIAN_POINT('Ctrl Pts',(-4.48708384594589,-2.50487961228577,
6.46585170802825));
#11315=CARTESIAN_POINT('Ctrl Pts',(-4.55582352295105,-2.37290383080013,
6.45778476398143));
#11316=CARTESIAN_POINT('Ctrl Pts',(-4.62455904179996,-2.2409360327084,6.44971830791498));
#11317=CARTESIAN_POINT('Ctrl Pts',(-4.68755602234724,-2.10598090587611,
6.44165185184854));
#11318=CARTESIAN_POINT('Ctrl Pts',(-4.74457425527497,-1.96855675526055,
6.4335853957821));
#11319=CARTESIAN_POINT('Ctrl Pts',(-4.80160671771683,-1.83109830896811,
6.42551692664467));
#11320=CARTESIAN_POINT('Ctrl Pts',(-4.85265732358227,-1.69116991330361,
6.41744845750724));
#11321=CARTESIAN_POINT('Ctrl Pts',(-4.89753404496007,-1.54930979502393,
6.40937998836981));
#11322=CARTESIAN_POINT('Ctrl Pts',(-4.9307837234018,-1.44420400360935,6.40340196689007));
#11323=CARTESIAN_POINT('Ctrl Pts',(-4.96064524398971,-1.33803822219086,
6.39742394541034));
#11324=CARTESIAN_POINT('Ctrl Pts',(-4.98705816036214,-1.23103674505086,
6.3914459239306));
#11325=CARTESIAN_POINT('Ctrl Pts',(-5.02320823666945,-1.0845890181484,6.38326409616073));
#11326=CARTESIAN_POINT('Ctrl Pts',(-5.05290817629628,-0.936528220354522,
6.37508226839086));
#11327=CARTESIAN_POINT('Ctrl Pts',(-5.07603746558229,-0.787428860599461,
6.36690044062098));
#11328=CARTESIAN_POINT('Ctrl Pts',(-5.09916160595338,-0.638362692522116,
6.35872043424451));
#11329=CARTESIAN_POINT('Ctrl Pts',(-5.11571796687674,-0.488258730911634,
6.35054042786805));
#11330=CARTESIAN_POINT('Ctrl Pts',(-5.12563745358772,-0.33769995096059,
6.34236042149158));
#11331=CARTESIAN_POINT('Ctrl Pts',(-5.13304226630334,-0.225309098418272,
6.33625411609542));
#11332=CARTESIAN_POINT('Ctrl Pts',(-5.13674974008113,-0.112665007672855,
6.33014781069927));
#11333=CARTESIAN_POINT('Ctrl Pts',(-5.13674999998633,-1.18511375680025E-5,
6.32404150530312));
#11334=CARTESIAN_POINT('Ctrl Pts',(-5.13674999993655,-2.55313104141619E-5,
6.32378934850487));
#11335=CARTESIAN_POINT('Ctrl Pts',(-5.13675175881838,0.353851183330079,
6.30459076071832));
#11336=CARTESIAN_POINT('Ctrl Pts',(-5.10018553184707,0.706781009868396,
6.28575565506401));
#11337=CARTESIAN_POINT('Ctrl Pts',(-5.01097029336203,1.13268802209302,6.26235343972258));
#11338=CARTESIAN_POINT('Ctrl Pts',(-4.99242291290921,1.21182448726008,6.25797201038631));
#11339=CARTESIAN_POINT('Ctrl Pts',(-4.90528205000358,1.54756212131146,6.23917043738623));
#11340=CARTESIAN_POINT('Ctrl Pts',(-4.81872142881228,1.7990722902529,6.22455421264983));
#11341=CARTESIAN_POINT('Ctrl Pts',(-4.65257091141745,2.18241944463084,6.20168245279317));
#11342=CARTESIAN_POINT('Ctrl Pts',(-4.58585904589532,2.31932507128563,6.1933810177971));
#11343=CARTESIAN_POINT('Ctrl Pts',(-4.44454904821096,2.57930788189307,6.17732565126477));
#11344=CARTESIAN_POINT('Ctrl Pts',(-4.37070278764835,2.7025468175416,6.16957809495441));
#11345=CARTESIAN_POINT('Ctrl Pts',(-4.29183649439967,2.8224705610226,6.16186016520308));
#11346=CARTESIAN_POINT('Origin',(0.,0.,0.));
#11347=CARTESIAN_POINT('',(-4.29183634723918,2.82247078479419,4.41198748894216));
#11348=CARTESIAN_POINT('',(-4.29183618112783,2.82247103738233,4.88896334675683));
#11349=CARTESIAN_POINT('',(-4.29183622825304,2.82247096572397,0.));
#11350=CARTESIAN_POINT('Ctrl Pts',(-4.29183618112783,2.82247103738234,4.88896334675683));
#11351=CARTESIAN_POINT('Ctrl Pts',(-4.35076667494944,2.73286160571572,4.89484305890014));
#11352=CARTESIAN_POINT('Ctrl Pts',(-4.40688922721175,2.64140882838337,4.90071687591498));
#11353=CARTESIAN_POINT('Ctrl Pts',(-4.49902899138872,2.4801393544412,4.91085775786024));
#11354=CARTESIAN_POINT('Ctrl Pts',(-4.53637581793597,2.41115070099564,4.91513024842132));
#11355=CARTESIAN_POINT('Ctrl Pts',(-4.65490048988083,2.17969711237887,4.92925757696788));
#11356=CARTESIAN_POINT('Ctrl Pts',(-4.72904407135895,2.01378308427835,4.93904982177472));
#11357=CARTESIAN_POINT('Ctrl Pts',(-4.86203773616973,1.66806482258989,4.95895017141693));
#11358=CARTESIAN_POINT('Ctrl Pts',(-4.92006091600445,1.48823766118503,4.96904016528542));
#11359=CARTESIAN_POINT('Ctrl Pts',(-4.98148356785063,1.25451763246555,4.98203334701867));
#11360=CARTESIAN_POINT('Ctrl Pts',(-4.99412551682467,1.20320541802812,4.98487908351888));
#11361=CARTESIAN_POINT('Ctrl Pts',(-5.02848941190195,1.05384047643724,4.99315588135523));
#11362=CARTESIAN_POINT('Ctrl Pts',(-5.04812996977751,0.955336836620863,
4.9986127844951));
#11363=CARTESIAN_POINT('Ctrl Pts',(-5.09815841771197,0.659434726490387,
5.01499992341947));
#11364=CARTESIAN_POINT('Ctrl Pts',(-5.11993756290548,0.460773957801797,
5.02597188807525));
#11365=CARTESIAN_POINT('Ctrl Pts',(-5.13453025535386,0.174331876064929,
5.04167125775976));
#11366=CARTESIAN_POINT('Ctrl Pts',(-5.13674863816779,0.0872134508755163,
5.04643134595567));
#11367=CARTESIAN_POINT('Ctrl Pts',(-5.13675261505373,-0.167352117693572,
5.06030159264728));
#11368=CARTESIAN_POINT('Ctrl Pts',(-5.12856906637668,-0.334686869971494,
5.06936667163545));
#11369=CARTESIAN_POINT('Ctrl Pts',(-5.09454248799109,-0.681670387724374,
5.08815307217164));
#11370=CARTESIAN_POINT('Ctrl Pts',(-5.06732638629499,-0.860953938580389,
5.09785328912853));
#11371=CARTESIAN_POINT('Ctrl Pts',(-4.99886041106813,-1.1926403364,5.11601577130758));
#11372=CARTESIAN_POINT('Ctrl Pts',(-4.9599536683695,-1.34530826903399,5.12446531774806));
#11373=CARTESIAN_POINT('Ctrl Pts',(-4.82548190008043,-1.78704071595509,
5.14951732576378));
#11374=CARTESIAN_POINT('Ctrl Pts',(-4.71117701145238,-2.06968627579925,
5.16628477743318));
#11375=CARTESIAN_POINT('Ctrl Pts',(-4.4940214701316,-2.49392446646106,5.19231923691255));
#11376=CARTESIAN_POINT('Ctrl Pts',(-4.40784445491978,-2.64325508881694,
5.20167777347038));
#11377=CARTESIAN_POINT('Ctrl Pts',(-4.2703745437973,-2.8559865329779,5.21535912339026));
#11378=CARTESIAN_POINT('Ctrl Pts',(-4.22482191454289,-2.92295018554061,
5.21972072900632));
#11379=CARTESIAN_POINT('Ctrl Pts',(-4.11009496461746,-3.08331349243077,
5.23032162209334));
#11380=CARTESIAN_POINT('Ctrl Pts',(-4.03929751456115,-3.17549657449616,
5.23654896067303));
#11381=CARTESIAN_POINT('Ctrl Pts',(-3.85270804337653,-3.40210090516477,
5.25228662469231));
#11382=CARTESIAN_POINT('Ctrl Pts',(-3.7329695374097,-3.5330703291436,5.26178746264883));
#11383=CARTESIAN_POINT('Ctrl Pts',(-3.48367786934961,-3.7788940600989,5.28077396470312));
#11384=CARTESIAN_POINT('Ctrl Pts',(-3.35461436601722,-3.89391993255668,
5.29024323451936));
#11385=CARTESIAN_POINT('Ctrl Pts',(-3.02579250576841,-4.15847485742709,
5.31338563258738));
#11386=CARTESIAN_POINT('Ctrl Pts',(-2.82046177660664,-4.30038760683045,
5.32702240745528));
#11387=CARTESIAN_POINT('Ctrl Pts',(-2.41269658561049,-4.54039858685244,
5.35268131936462));
#11388=CARTESIAN_POINT('Ctrl Pts',(-2.2125347411642,-4.64123012568271,5.36470256018284));
#11389=CARTESIAN_POINT('Ctrl Pts',(-1.81818606140417,-4.80855655972018,
5.38767251058753));
#11390=CARTESIAN_POINT('Ctrl Pts',(-1.62534268444444,-4.87711747043902,
5.39860607350409));
#11391=CARTESIAN_POINT('Ctrl Pts',(-1.28883363923448,-4.97457354426541,
5.41759486411576));
#11392=CARTESIAN_POINT('Ctrl Pts',(-1.14707417045461,-5.00916093916427,
5.42557468777306));
#11393=CARTESIAN_POINT('Ctrl Pts',(-0.712504788672453,-5.09577329946574,
5.44986341754238));
#11394=CARTESIAN_POINT('Ctrl Pts',(-0.416469418077995,-5.12846270969461,
5.4661413171253));
#11395=CARTESIAN_POINT('Ctrl Pts',(0.101206793825572,-5.14048571251202,
5.49418906878275));
#11396=CARTESIAN_POINT('Ctrl Pts',(0.32178524065613,-5.13140262919381,5.50601932938985));
#11397=CARTESIAN_POINT('Ctrl Pts',(0.727947503460507,-5.08837864068416,
5.52791716391643));
#11398=CARTESIAN_POINT('Ctrl Pts',(0.913566335216109,-5.05834941959818,
5.53797288310535));
#11399=CARTESIAN_POINT('Ctrl Pts',(1.22824756609194,-4.98955160405469,5.55542530478754));
#11400=CARTESIAN_POINT('Ctrl Pts',(1.35819995898229,-4.95575510375443,5.56276205078095));
#11401=CARTESIAN_POINT('Ctrl Pts',(1.79047535739138,-4.82505233274795,5.58750611267025));
#11402=CARTESIAN_POINT('Ctrl Pts',(2.08511671918455,-4.70523430195556,5.60489516509617));
#11403=CARTESIAN_POINT('Ctrl Pts',(2.56115582484357,-4.45809705594016,5.63393677711287));
#11404=CARTESIAN_POINT('Ctrl Pts',(2.74884884910895,-4.34487984782121,5.64568003104302));
#11405=CARTESIAN_POINT('Ctrl Pts',(3.07900775626645,-4.11574606299812,5.66722605964057));
#11406=CARTESIAN_POINT('Ctrl Pts',(3.22359050743026,-4.0035130040499,5.67701737438513));
#11407=CARTESIAN_POINT('Ctrl Pts',(3.46097767781925,-3.79802763496036,5.6940262473911));
#11408=CARTESIAN_POINT('Ctrl Pts',(3.55675720378763,-3.70848447643342,5.70118848483755));
#11409=CARTESIAN_POINT('Ctrl Pts',(3.87672233774735,-3.38554336959448,5.72609369491122));
#11410=CARTESIAN_POINT('Ctrl Pts',(4.08222306912352,-3.13470012865412,5.74382306491193));
#11411=CARTESIAN_POINT('Ctrl Pts',(4.38607728400062,-2.68279145605713,5.77330449563059));
#11412=CARTESIAN_POINT('Ctrl Pts',(4.49742990286746,-2.4916200684532,5.78515406010949));
#11413=CARTESIAN_POINT('Ctrl Pts',(4.68108485635258,-2.12363886161213,5.80720310961879));
#11414=CARTESIAN_POINT('Ctrl Pts',(4.75652051110564,-1.94882207014414,5.81738869919237));
#11415=CARTESIAN_POINT('Ctrl Pts',(4.88407969953336,-1.60135214897491,5.83747048028227));
#11416=CARTESIAN_POINT('Ctrl Pts',(4.93714988064486,-1.42933474119038,5.84733204546999));
#11417=CARTESIAN_POINT('Ctrl Pts',(5.03972250490122,-1.02224261884155,5.87035297090975));
#11418=CARTESIAN_POINT('Ctrl Pts',(5.08201819096381,-0.785489198455414,
5.88349119731374));
#11419=CARTESIAN_POINT('Ctrl Pts',(5.1321025676287,-0.31752263634635,5.90901139921348));
#11420=CARTESIAN_POINT('Ctrl Pts',(5.14117978245887,-0.0870107790218277,
5.92137820564444));
#11421=CARTESIAN_POINT('Ctrl Pts',(5.1293031738,0.338454165328436,5.94419891307366));
#11422=CARTESIAN_POINT('Ctrl Pts',(5.11273914575662,0.533102216108032,5.95464119155864));
#11423=CARTESIAN_POINT('Ctrl Pts',(5.0654556216585,0.864140570948428,5.97276249389672));
#11424=CARTESIAN_POINT('Ctrl Pts',(5.04017813134208,1.00109061540283,5.98037479488938));
#11425=CARTESIAN_POINT('Ctrl Pts',(4.94113634553711,1.43750759598957,6.00489954169758));
#11426=CARTESIAN_POINT('Ctrl Pts',(4.84596944145801,1.73142872882405,6.02178748625493));
#11427=CARTESIAN_POINT('Ctrl Pts',(4.63611254522064,2.22351698621223,6.0507585970176));
#11428=CARTESIAN_POINT('Ctrl Pts',(4.53350467082986,2.42588236888161,6.06290992577457));
#11429=CARTESIAN_POINT('Ctrl Pts',(4.32150440810181,2.78324843096805,6.08518690693516));
#11430=CARTESIAN_POINT('Ctrl Pts',(4.21625801619962,2.94024453447699,6.09529909828665));
#11431=CARTESIAN_POINT('Ctrl Pts',(4.0008265096165,3.22617363943583,6.11472131811095));
#11432=CARTESIAN_POINT('Ctrl Pts',(3.89243590534358,3.35615110775703,6.12399112259118));
#11433=CARTESIAN_POINT('Ctrl Pts',(3.60845866095431,3.66438429088189,6.14697293205562));
#11434=CARTESIAN_POINT('Ctrl Pts',(3.42588686792987,3.83562121634691,6.16064877382191));
#11435=CARTESIAN_POINT('Ctrl Pts',(3.0575908520117,4.1336951366118,6.18634277346802));
#11436=CARTESIAN_POINT('Ctrl Pts',(2.87459021028,4.26298385421086,6.19836084857391));
#11437=CARTESIAN_POINT('Ctrl Pts',(2.50930445417532,4.48680764122961,6.2213321813699));
#11438=CARTESIAN_POINT('Ctrl Pts',(2.3286441985642,4.58317191110622,6.23227025220367));
#11439=CARTESIAN_POINT('Ctrl Pts',(2.01011045436244,4.72937073494544,6.25126694722387));
#11440=CARTESIAN_POINT('Ctrl Pts',(1.87496621935885,4.78455762145455,6.25925008577663));
#11441=CARTESIAN_POINT('Ctrl Pts',(1.45800616493269,4.93444325976642,6.28353694626568));
#11442=CARTESIAN_POINT('Ctrl Pts',(1.17014907750794,5.01051607499201,6.29980961136405));
#11443=CARTESIAN_POINT('Ctrl Pts',(0.660080505383652,5.0989321998958,6.32784977733062));
#11444=CARTESIAN_POINT('Ctrl Pts',(0.440630106783252,5.12256414988613,6.33967761486079));
#11445=CARTESIAN_POINT('Ctrl Pts',(0.0325309836741374,5.14008550698156,
6.3615776261939));
#11446=CARTESIAN_POINT('Ctrl Pts',(-0.155574449815248,5.13783333831406,
6.37163792855709));
#11447=CARTESIAN_POINT('Ctrl Pts',(-0.477111820295809,5.11630695044312,
6.38909814649617));
#11448=CARTESIAN_POINT('Ctrl Pts',(-0.610688937314607,5.10208682847716,
6.39643802524681));
#11449=CARTESIAN_POINT('Ctrl Pts',(-1.05748535164622,5.03672399017357,6.42117936172845));
#11450=CARTESIAN_POINT('Ctrl Pts',(-1.36649822918216,4.96180974567678,6.43856247765311));
#11451=CARTESIAN_POINT('Ctrl Pts',(-1.8727932559441,4.78814713298114,6.46754369058711));
#11452=CARTESIAN_POINT('Ctrl Pts',(-2.07425500578036,4.70437839353973,6.47923352004727));
#11453=CARTESIAN_POINT('Ctrl Pts',(-2.43505842376461,4.52665798603239,6.5007967269021));
#11454=CARTESIAN_POINT('Ctrl Pts',(-2.59582700116256,4.43641994168349,6.51065843586246));
#11455=CARTESIAN_POINT('Ctrl Pts',(-2.8627716029435,4.26709903664984,6.52778417868107));
#11456=CARTESIAN_POINT('Ctrl Pts',(-2.9713817741071,4.19219325645766,6.53499165756809));
#11457=CARTESIAN_POINT('Ctrl Pts',(-3.33219938525618,3.92227378166827,6.55967855836324));
#11458=CARTESIAN_POINT('Ctrl Pts',(-3.56909740785504,3.70800992819532,6.57714451091868));
#11459=CARTESIAN_POINT('Ctrl Pts',(-3.93920150163499,3.3047190286957,6.60678579541625));
#11460=CARTESIAN_POINT('Ctrl Pts',(-4.08237593636468,3.12612949197814,6.6190420456666));
#11461=CARTESIAN_POINT('Ctrl Pts',(-4.23992760663097,2.90024154009261,6.63380724808002));
#11462=CARTESIAN_POINT('Ctrl Pts',(-4.26614956753193,2.86152998221862,6.63631380382691));
#11463=CARTESIAN_POINT('Ctrl Pts',(-4.29183621579633,2.82247098466558,6.63882185511496));
#11464=CARTESIAN_POINT('Ctrl Pts',(-4.29183649439966,2.8224705610226,6.16186016520308));
#11465=CARTESIAN_POINT('Ctrl Pts',(-4.19725390933125,2.96629242968514,6.15260422432914));
#11466=CARTESIAN_POINT('Ctrl Pts',(-4.09545108415786,3.10534617699547,6.14339199955404));
#11467=CARTESIAN_POINT('Ctrl Pts',(-3.90218522766283,3.34322503928577,6.12694209094475));
#11468=CARTESIAN_POINT('Ctrl Pts',(-3.81353312405755,3.4440045650993,6.11972652822776));
#11469=CARTESIAN_POINT('Ctrl Pts',(-3.5915626956095,3.67724782599031,6.10224279270102));
#11470=CARTESIAN_POINT('Ctrl Pts',(-3.45472490639275,3.80609358067502,6.09193707841706));
#11471=CARTESIAN_POINT('Ctrl Pts',(-3.14250599113566,4.06933786739302,6.06954496239244));
#11472=CARTESIAN_POINT('Ctrl Pts',(-2.96488438196448,4.20051409112443,6.05748849496811));
#11473=CARTESIAN_POINT('Ctrl Pts',(-2.52930807527318,4.48076149686582,6.02939343924952));
#11474=CARTESIAN_POINT('Ctrl Pts',(-2.26573715376429,4.61963872422158,6.01349904927813));
#11475=CARTESIAN_POINT('Ctrl Pts',(-1.85723845235867,4.79146358774224,5.98972503912635));
#11476=CARTESIAN_POINT('Ctrl Pts',(-1.72050094412173,4.84224465263094,5.98189300166352));
#11477=CARTESIAN_POINT('Ctrl Pts',(-1.38731964776934,4.9500833824721,5.96288438992435));
#11478=CARTESIAN_POINT('Ctrl Pts',(-1.18926746821426,5.00136204605316,5.95166118322735));
#11479=CARTESIAN_POINT('Ctrl Pts',(-0.768935238839542,5.08380658744256,
5.92817911252273));
#11480=CARTESIAN_POINT('Ctrl Pts',(-0.546592339084737,5.11249366174593,
5.91595152211607));
#11481=CARTESIAN_POINT('Ctrl Pts',(-0.0759509131320661,5.14215418998918,
5.89040169538602));
#11482=CARTESIAN_POINT('Ctrl Pts',(0.171987736413737,5.13983866357537,5.87713661866262));
#11483=CARTESIAN_POINT('Ctrl Pts',(0.591263223056248,5.10554142019864,5.85458192794348));
#11484=CARTESIAN_POINT('Ctrl Pts',(0.762906708664317,5.08272727259404,5.84530766423137));
#11485=CARTESIAN_POINT('Ctrl Pts',(1.11226441971272,5.01819446413918,5.82603773727903));
#11486=CARTESIAN_POINT('Ctrl Pts',(1.28957095845087,4.97558272649148,5.81604448562454));
#11487=CARTESIAN_POINT('Ctrl Pts',(1.70149904446022,4.85307871146888,5.79247841485924));
#11488=CARTESIAN_POINT('Ctrl Pts',(1.93333421223393,4.76546796703958,5.7789475584529));
#11489=CARTESIAN_POINT('Ctrl Pts',(2.33117697936211,4.58129370685745,5.75518820385545));
#11490=CARTESIAN_POINT('Ctrl Pts',(2.49979930575679,4.49150793975523,5.74492616201104));
#11491=CARTESIAN_POINT('Ctrl Pts',(2.84107775545857,4.2846036322245,5.72351690090885));
#11492=CARTESIAN_POINT('Ctrl Pts',(3.01239072911943,4.16593935513081,5.71239424761735));
#11493=CARTESIAN_POINT('Ctrl Pts',(3.25970275563985,3.97138181260307,5.69538040988315));
#11494=CARTESIAN_POINT('Ctrl Pts',(3.34131024906505,3.90297070011646,5.68958316397548));
#11495=CARTESIAN_POINT('Ctrl Pts',(3.65899377046751,3.61938805472154,5.66630084388965));
#11496=CARTESIAN_POINT('Ctrl Pts',(3.87690797328752,3.38493682553852,5.64874946335737));
#11497=CARTESIAN_POINT('Ctrl Pts',(4.18533277008768,2.98395166433981,5.62127715473111));
#11498=CARTESIAN_POINT('Ctrl Pts',(4.29089743734252,2.83004934223808,5.6112282659875));
#11499=CARTESIAN_POINT('Ctrl Pts',(4.51526997353433,2.46141991961872,5.58805398293149));
#11500=CARTESIAN_POINT('Ctrl Pts',(4.62753520096295,2.24324883224769,5.57498893735118));
#11501=CARTESIAN_POINT('Ctrl Pts',(4.76659109010211,1.91772694692146,5.5558434368822));
#11502=CARTESIAN_POINT('Ctrl Pts',(4.80618591328844,1.81621669319552,5.54990852336167));
#11503=CARTESIAN_POINT('Ctrl Pts',(4.9073630203892,1.53028454583526,5.53332027145507));
#11504=CARTESIAN_POINT('Ctrl Pts',(4.96175024495561,1.34350938206039,5.52264265023909));
#11505=CARTESIAN_POINT('Ctrl Pts',(5.02416708917492,1.07280310674512,5.50744749504817));
#11506=CARTESIAN_POINT('Ctrl Pts',(5.04092883804701,0.991059076741259,5.50289366739454));
#11507=CARTESIAN_POINT('Ctrl Pts',(5.08561676379312,0.742497274432245,5.48914553749949));
#11508=CARTESIAN_POINT('Ctrl Pts',(5.10730382298176,0.574673438170269,5.47999985348081));
#11509=CARTESIAN_POINT('Ctrl Pts',(5.14612836540326,0.0850996471055538,
5.4535602820455));
#11510=CARTESIAN_POINT('Ctrl Pts',(5.14134576107469,-0.237559152087237,
5.43646659019121));
#11511=CARTESIAN_POINT('Ctrl Pts',(5.08679226888453,-0.737118438938526,
5.40920716678854));
#11512=CARTESIAN_POINT('Ctrl Pts',(5.05774296952375,-0.915441678129262,
5.39930679155705));
#11513=CARTESIAN_POINT('Ctrl Pts',(4.97043138119144,-1.31681923342578,5.37678220263966));
#11514=CARTESIAN_POINT('Ctrl Pts',(4.90642772221416,-1.53823657711337,5.36418932725019));
#11515=CARTESIAN_POINT('Ctrl Pts',(4.71934063016897,-2.05300270962597,5.33446833855216));
#11516=CARTESIAN_POINT('Ctrl Pts',(4.58346448588307,-2.3406950393242,5.31751698212112));
#11517=CARTESIAN_POINT('Ctrl Pts',(4.35362020290054,-2.72950449897037,5.29327550687882));
#11518=CARTESIAN_POINT('Ctrl Pts',(4.28084272351437,-2.84228576605228,5.28605985193424));
#11519=CARTESIAN_POINT('Ctrl Pts',(4.09579651057626,-3.10578912897284,5.26857587871268));
#11520=CARTESIAN_POINT('Ctrl Pts',(3.97951192525345,-3.25345329763332,5.25827001740642));
#11521=CARTESIAN_POINT('Ctrl Pts',(3.70964632072762,-3.55996883882456,5.23587783364701));
#11522=CARTESIAN_POINT('Ctrl Pts',(3.55337336087219,-3.71596490313294,5.22382144489708));
#11523=CARTESIAN_POINT('Ctrl Pts',(3.16402459396092,-4.05753244874945,5.19572662495801));
#11524=CARTESIAN_POINT('Ctrl Pts',(2.92388723522484,-4.23385267815995,5.17983238770126));
#11525=CARTESIAN_POINT('Ctrl Pts',(2.54528540766308,-4.46418869564088,5.15605843637834));
#11526=CARTESIAN_POINT('Ctrl Pts',(2.41755766957114,-4.53463032937321,5.14822630160392));
#11527=CARTESIAN_POINT('Ctrl Pts',(2.10397938392896,-4.69054934057154,5.12921744965009));
#11528=CARTESIAN_POINT('Ctrl Pts',(1.91568358977597,-4.77054890723372,5.11799409864902));
#11529=CARTESIAN_POINT('Ctrl Pts',(1.51216057300273,-4.91423650237626,5.09451198629455));
#11530=CARTESIAN_POINT('Ctrl Pts',(1.29650486924802,-4.97548278363567,5.08228449711849));
#11531=CARTESIAN_POINT('Ctrl Pts',(0.83651342401759,-5.07417114992291,5.05679515098435));
#11532=CARTESIAN_POINT('Ctrl Pts',(0.592076705526503,-5.10846510642551,
5.04358885557984));
#11533=CARTESIAN_POINT('Ctrl Pts',(0.173335422487548,-5.1367447373362,5.02108693358169));
#11534=CARTESIAN_POINT('Ctrl Pts',(7.31257870932242E-5,-5.13966822455429,
5.01180611869767));
#11535=CARTESIAN_POINT('Ctrl Pts',(-0.403813977630477,-5.12605790564199,
4.9898895015897));
#11536=CARTESIAN_POINT('Ctrl Pts',(-0.633836265327348,-5.10272325256985,
4.97719683718441));
#11537=CARTESIAN_POINT('Ctrl Pts',(-1.01563570440475,-5.03777024302909,
4.95597468649871));
#11538=CARTESIAN_POINT('Ctrl Pts',(-1.16849236970092,-5.00452512410979,
4.94743231178558));
#11539=CARTESIAN_POINT('Ctrl Pts',(-1.49044311109576,-4.91894612871971,
4.92932428038163));
#11540=CARTESIAN_POINT('Ctrl Pts',(-1.65883428994811,-4.86474279428754,
4.91978387849841));
#11541=CARTESIAN_POINT('Ctrl Pts',(-2.04932212205834,-4.7164101820224,4.8973300927706));
#11542=CARTESIAN_POINT('Ctrl Pts',(-2.26824587812907,-4.61511697808785,
4.88448311157));
#11543=CARTESIAN_POINT('Ctrl Pts',(-2.51600913742638,-4.47857793172112,
4.86922614022122));
#11544=CARTESIAN_POINT('Ctrl Pts',(-2.55251948563139,-4.45787017510926,
4.86695819402372));
#11545=CARTESIAN_POINT('Ctrl Pts',(-2.6955856090148,-4.37439279926031,4.8579837487011));
#11546=CARTESIAN_POINT('Ctrl Pts',(-2.80011183965857,-4.30823241737501,
4.85122853323049));
#11547=CARTESIAN_POINT('Ctrl Pts',(-3.06787887433788,-4.1248836774479,4.83345404965342));
#11548=CARTESIAN_POINT('Ctrl Pts',(-3.22681415472045,-4.00177681714965,
4.82242681106416));
#11549=CARTESIAN_POINT('Ctrl Pts',(-3.43719081487231,-3.81812334439494,
4.80717991422066));
#11550=CARTESIAN_POINT('Ctrl Pts',(-3.49506181699057,-3.76522106227782,
4.80290980517107));
#11551=CARTESIAN_POINT('Ctrl Pts',(-3.68310624358796,-3.58524943597255,
4.78876912574235));
#11552=CARTESIAN_POINT('Ctrl Pts',(-3.80774178924914,-3.45259173071376,
4.77896144642471));
#11553=CARTESIAN_POINT('Ctrl Pts',(-4.07586696421642,-3.13498779893074,
4.75663172151737));
#11554=CARTESIAN_POINT('Ctrl Pts',(-4.2142848997596,-2.94629267526063,4.74416361301676));
#11555=CARTESIAN_POINT('Ctrl Pts',(-4.36111019268017,-2.7145108210406,4.7293575864247));
#11556=CARTESIAN_POINT('Ctrl Pts',(-4.38244282748342,-2.67993394120567,
4.7271609838702));
#11557=CARTESIAN_POINT('Ctrl Pts',(-4.52411871659907,-2.44408331484917,
4.71224489691283));
#11558=CARTESIAN_POINT('Ctrl Pts',(-4.63096519517049,-2.23502836797372,
4.6993555257995));
#11559=CARTESIAN_POINT('Ctrl Pts',(-4.78454635710325,-1.87582081026763,
4.67794880073465));
#11560=CARTESIAN_POINT('Ctrl Pts',(-4.83935972053827,-1.72950463456054,
4.66941687705839));
#11561=CARTESIAN_POINT('Ctrl Pts',(-4.94194684680734,-1.41235545454078,
4.65129897979436));
#11562=CARTESIAN_POINT('Ctrl Pts',(-4.98771496044528,-1.24108340528471,
4.64173870813363));
#11563=CARTESIAN_POINT('Ctrl Pts',(-5.07794139622615,-0.816516849869994,
4.61840797605637));
#11564=CARTESIAN_POINT('Ctrl Pts',(-5.11241548553482,-0.561598795219459,
4.6047210912281));
#11565=CARTESIAN_POINT('Ctrl Pts',(-5.1337232019056,-0.203580757021962,
4.5853456424715));
#11566=CARTESIAN_POINT('Ctrl Pts',(-5.13674886148609,-0.101829509366764,
4.57981171115969));
#11567=CARTESIAN_POINT('Ctrl Pts',(-5.13675161298497,0.144194971788234,
4.56637234854805));
#11568=CARTESIAN_POINT('Ctrl Pts',(-5.13067679167021,0.288382805314253,
4.55845572529731));
#11569=CARTESIAN_POINT('Ctrl Pts',(-5.1010468084383,0.639353262164002,4.53914770184875));
#11570=CARTESIAN_POINT('Ctrl Pts',(-5.07098266694131,0.845333617713159,
4.52778891312207));
#11571=CARTESIAN_POINT('Ctrl Pts',(-4.98278422769968,1.2681536796937,4.50436622563596));
#11572=CARTESIAN_POINT('Ctrl Pts',(-4.92276642765659,1.48415835872673,4.49234165092297));
#11573=CARTESIAN_POINT('Ctrl Pts',(-4.78137394854056,1.88850291919869,4.46937314064419));
#11574=CARTESIAN_POINT('Ctrl Pts',(-4.70244963657659,2.0772444369788,4.45844430968834));
#11575=CARTESIAN_POINT('Ctrl Pts',(-4.54832674288316,2.3916897379459,4.43946377574975));
#11576=CARTESIAN_POINT('Ctrl Pts',(-4.47861778415142,2.51980893655661,4.43148739053182));
#11577=CARTESIAN_POINT('Ctrl Pts',(-4.36751796376614,2.70478953924705,4.41965977358021));
#11578=CARTESIAN_POINT('Ctrl Pts',(-4.33026961532294,2.76402933066338,4.41582199283889));
#11579=CARTESIAN_POINT('Ctrl Pts',(-4.29183634723918,2.82247078479419,4.41198748894216));
#11580=CARTESIAN_POINT('Origin',(0.,0.,0.));
#11581=CARTESIAN_POINT('',(-4.29199677360937,2.82257643420045,2.66202500160396));
#11582=CARTESIAN_POINT('',(-4.29183621895492,2.82247097986264,3.13909688836532));
#11583=CARTESIAN_POINT('',(-4.29183622825304,2.82247096572397,0.));
#11584=CARTESIAN_POINT('',(-5.13675004007553,-0.000129368701075719,3.30088737635801));
#11585=CARTESIAN_POINT('Ctrl Pts',(-4.29183621895492,2.82247097986264,3.13909688836532));
#11586=CARTESIAN_POINT('Ctrl Pts',(-4.31434163625608,2.78824934719221,3.14129950131095));
#11587=CARTESIAN_POINT('Ctrl Pts',(-4.33643920649416,2.75375631830031,3.14350002919566));
#11588=CARTESIAN_POINT('Ctrl Pts',(-4.47026145774089,2.53926049515073,3.15707221045047));
#11589=CARTESIAN_POINT('Ctrl Pts',(-4.57117114657727,2.352758786316,3.16838340061208));
#11590=CARTESIAN_POINT('Ctrl Pts',(-4.69788620924262,2.07943778774776,3.18463611438416));
#11591=CARTESIAN_POINT('Ctrl Pts',(-4.73337101716958,1.99734691669373,3.18948360463754));
#11592=CARTESIAN_POINT('Ctrl Pts',(-4.89764401713157,1.58831497354132,3.21350853176904));
#11593=CARTESIAN_POINT('Ctrl Pts',(-4.99479460385032,1.24967860481255,3.23285629740859));
#11594=CARTESIAN_POINT('Ctrl Pts',(-5.07504813350195,0.800661998792021,
3.25763833275876));
#11595=CARTESIAN_POINT('Ctrl Pts',(-5.0903199759671,0.697005156173732,3.26330725016343));
#11596=CARTESIAN_POINT('Ctrl Pts',(-5.12528966797252,0.396087887183829,
3.27965022342625));
#11597=CARTESIAN_POINT('Ctrl Pts',(-5.13675498680471,0.198063051843214,
3.29025921997661));
#11598=CARTESIAN_POINT('Ctrl Pts',(-5.13674999837291,-0.00012929019744156,
3.3008872998628));
#11599=CARTESIAN_POINT('Ctrl Pts',(-5.13674999837083,-0.000129372565223704,
3.30088730427978));
#11600=CARTESIAN_POINT('Ctrl Pts',(-5.13674612579616,-0.153890318034086,
3.3091327470438));
#11601=CARTESIAN_POINT('Ctrl Pts',(-5.12983834509799,-0.307571136377627,
3.31738214574149));
#11602=CARTESIAN_POINT('Ctrl Pts',(-5.10272874859786,-0.608616870674754,
3.3337678624906));
#11603=CARTESIAN_POINT('Ctrl Pts',(-5.08300150008219,-0.755876525193646,
3.34189484704342));
#11604=CARTESIAN_POINT('Ctrl Pts',(-5.00935481136442,-1.16873260684651,
3.36488401408925));
#11605=CARTESIAN_POINT('Ctrl Pts',(-4.94076786556144,-1.43121980420412,
3.37972203588897));
#11606=CARTESIAN_POINT('Ctrl Pts',(-4.78716696880529,-1.87295550571598,
3.40509359150357));
#11607=CARTESIAN_POINT('Ctrl Pts',(-4.71190277537752,-2.05497067164751,
3.41568078862056));
#11608=CARTESIAN_POINT('Ctrl Pts',(-4.55526944016961,-2.37960048042415,
3.43502067681698));
#11609=CARTESIAN_POINT('Ctrl Pts',(-4.47715742144368,-2.52349736779438,
3.44377263470832));
#11610=CARTESIAN_POINT('Ctrl Pts',(-4.35145585254996,-2.7307949740682,3.45681705808139));
#11611=CARTESIAN_POINT('Ctrl Pts',(-4.30905599440955,-2.79722100846318,
3.4610678026599));
#11612=CARTESIAN_POINT('Ctrl Pts',(-4.16534636182157,-3.01133857811476,
3.47505487145739));
#11613=CARTESIAN_POINT('Ctrl Pts',(-4.05784101596219,-3.15470994959003,
3.48487359093311));
#11614=CARTESIAN_POINT('Ctrl Pts',(-3.86868100961065,-3.38126898125076,
3.50105814060987));
#11615=CARTESIAN_POINT('Ctrl Pts',(-3.79129258578506,-3.46781970266228,
3.50741994673028));
#11616=CARTESIAN_POINT('Ctrl Pts',(-3.65506526521694,-3.61015954435536,
3.51818893400671));
#11617=CARTESIAN_POINT('Ctrl Pts',(-3.59771693372384,-3.66731333308679,
3.5226038915113));
#11618=CARTESIAN_POINT('Ctrl Pts',(-3.41412528901304,-3.84182932458607,
3.53638211105508));
#11619=CARTESIAN_POINT('Ctrl Pts',(-3.28331062935476,-3.95421006601779,
3.54569255021215));
#11620=CARTESIAN_POINT('Ctrl Pts',(-2.90644726189053,-4.24634830595016,
3.57134267597798));
#11621=CARTESIAN_POINT('Ctrl Pts',(-2.64969765551798,-4.41112280617052,
3.58752328436325));
#11622=CARTESIAN_POINT('Ctrl Pts',(-2.21216641867224,-4.63986366384214,
3.61429693512724));
#11623=CARTESIAN_POINT('Ctrl Pts',(-2.03974086582732,-4.7182062431308,3.62467758210589));
#11624=CARTESIAN_POINT('Ctrl Pts',(-1.65695218080982,-4.8672152455183,3.6472018832576));
#11625=CARTESIAN_POINT('Ctrl Pts',(-1.44552884790294,-4.93413867833424,
3.65931690279207));
#11626=CARTESIAN_POINT('Ctrl Pts',(-0.915591744015469,-5.06488482932643,
3.68894017476201));
#11627=CARTESIAN_POINT('Ctrl Pts',(-0.594089770907524,-5.11257544983285,
3.70624874556336));
#11628=CARTESIAN_POINT('Ctrl Pts',(-0.139719207230433,-5.13651263367917,
3.73067366122826));
#11629=CARTESIAN_POINT('Ctrl Pts',(-0.00898646934228279,-5.13840461067615,
3.73770509894011));
#11630=CARTESIAN_POINT('Ctrl Pts',(0.303919311190788,-5.1309906513171,3.7547031982634));
#11631=CARTESIAN_POINT('Ctrl Pts',(0.485801915032334,-5.11697439419366,
3.76470410231091));
#11632=CARTESIAN_POINT('Ctrl Pts',(0.884280653854546,-5.06482637645206,
3.78674019785601));
#11633=CARTESIAN_POINT('Ctrl Pts',(1.099962664156,-5.0224002196701,3.79874631966172));
#11634=CARTESIAN_POINT('Ctrl Pts',(1.61867843600075,-4.88533747872523,3.82785970059415));
#11635=CARTESIAN_POINT('Ctrl Pts',(1.9169385478368,-4.77619017812944,3.84478178084446));
#11636=CARTESIAN_POINT('Ctrl Pts',(2.32470922134776,-4.58257676006919,3.86900875663399));
#11637=CARTESIAN_POINT('Ctrl Pts',(2.44386770315813,-4.52015403342131,3.87624001468175));
#11638=CARTESIAN_POINT('Ctrl Pts',(2.72364881707301,-4.35928680110357,3.89376417740104));
#11639=CARTESIAN_POINT('Ctrl Pts',(2.88157436339059,-4.25654458778638,3.90409488791843));
#11640=CARTESIAN_POINT('Ctrl Pts',(3.21131227268516,-4.01524865699555,3.92649850801113));
#11641=CARTESIAN_POINT('Ctrl Pts',(3.38057046033108,-3.87382176793148,3.93854158899194));
#11642=CARTESIAN_POINT('Ctrl Pts',(3.75532550756194,-3.51736530069845,3.96659644484515));
#11643=CARTESIAN_POINT('Ctrl Pts',(3.9522858323587,-3.29450586352294,3.98246477019735));
#11644=CARTESIAN_POINT('Ctrl Pts',(4.21581890141645,-2.93843845624901,4.00622876913822));
#11645=CARTESIAN_POINT('Ctrl Pts',(4.29769016924388,-2.81734051255778,4.0140774425482));
#11646=CARTESIAN_POINT('Ctrl Pts',(4.4816796101353,-2.51847425437161,4.03312725249025));
#11647=CARTESIAN_POINT('Ctrl Pts',(4.57853956172384,-2.33776352584395,4.04437526366578));
#11648=CARTESIAN_POINT('Ctrl Pts',(4.75802507450122,-1.94869372409275,4.06786448074228));
#11649=CARTESIAN_POINT('Ctrl Pts',(4.83834280068921,-1.73972773045446,4.08007465942468));
#11650=CARTESIAN_POINT('Ctrl Pts',(4.97947792775408,-1.28615536694663,4.10581117586804));
#11651=CARTESIAN_POINT('Ctrl Pts',(5.03644746675353,-1.04095918568242,4.11927458788016));
#11652=CARTESIAN_POINT('Ctrl Pts',(5.10135403330102,-0.625332205992982,
4.1418294226555));
#11653=CARTESIAN_POINT('Ctrl Pts',(5.11918857432193,-0.456902156318874,
4.15090378545258));
#11654=CARTESIAN_POINT('Ctrl Pts',(5.13890002952896,-0.105764388778069,
4.16997982012417));
#11655=CARTESIAN_POINT('Ctrl Pts',(5.13941451232527,0.0767872595261164,
4.17998369442522));
#11656=CARTESIAN_POINT('Ctrl Pts',(5.11883901954797,0.484380370928735,4.20236278399278));
#11657=CARTESIAN_POINT('Ctrl Pts',(5.09261737623013,0.708794066694097,4.21470836249437));
#11658=CARTESIAN_POINT('Ctrl Pts',(4.99242249082055,1.2526056342636,4.24472100931902));
#11659=CARTESIAN_POINT('Ctrl Pts',(4.90250149117385,1.56805169444472,4.26218541645775));
#11660=CARTESIAN_POINT('Ctrl Pts',(4.73605830076253,1.99315295393288,4.2866941209861));
#11661=CARTESIAN_POINT('Ctrl Pts',(4.68440939389031,2.11168529819525,4.29364875186226));
#11662=CARTESIAN_POINT('Ctrl Pts',(4.55033203215963,2.39019358739317,4.31043659600053));
#11663=CARTESIAN_POINT('Ctrl Pts',(4.46386291414731,2.54803323190023,4.32030254736569));
#11664=CARTESIAN_POINT('Ctrl Pts',(4.2529073903596,2.88928594904022,4.34230145153023));
#11665=CARTESIAN_POINT('Ctrl Pts',(4.1244693497047,3.06984536201229,4.35440475484275));
#11666=CARTESIAN_POINT('Ctrl Pts',(3.7844839417774,3.48778272489964,4.38364002470495));
#11667=CARTESIAN_POINT('Ctrl Pts',(3.56179286452425,3.71491352300689,4.40058732566539));
#11668=CARTESIAN_POINT('Ctrl Pts',(3.21713929916307,4.00677292704103,4.42482678011335));
#11669=CARTESIAN_POINT('Ctrl Pts',(3.11135622352853,4.0894591484327,4.43204458430779));
#11670=CARTESIAN_POINT('Ctrl Pts',(2.85001470505729,4.27772310499848,4.4495341424321));
#11671=CARTESIAN_POINT('Ctrl Pts',(2.69166398992563,4.37909146968617,4.45984347662887));
#11672=CARTESIAN_POINT('Ctrl Pts',(2.33613725497451,4.58009845287954,4.48223724998594));
#11673=CARTESIAN_POINT('Ctrl Pts',(2.13736082214875,4.67616630069395,4.49429177003673));
#11674=CARTESIAN_POINT('Ctrl Pts',(1.6575879654358,4.87103511302511,4.52238105932679));
#11675=CARTESIAN_POINT('Ctrl Pts',(1.37295873461636,4.95878706027175,4.53827173640728));
#11676=CARTESIAN_POINT('Ctrl Pts',(0.939768756184492,5.05215851226198,4.56204430790658));
#11677=CARTESIAN_POINT('Ctrl Pts',(0.795957974736394,5.07680220634383,4.56987870270247));
#11678=CARTESIAN_POINT('Ctrl Pts',(0.448477893813733,5.12121813481024,4.58889319764682));
#11679=CARTESIAN_POINT('Ctrl Pts',(0.24429572456553,5.13500976941002,4.60011996561718));
#11680=CARTESIAN_POINT('Ctrl Pts',(-0.184051653057268,5.13833197426969,
4.62360305296982));
#11681=CARTESIAN_POINT('Ctrl Pts',(-0.407820268856465,5.12542846225274,
4.63582813403276));
#11682=CARTESIAN_POINT('Ctrl Pts',(-0.877026503496012,5.06744131284838,
4.66144299802282));
#11683=CARTESIAN_POINT('Ctrl Pts',(-1.12147490047326,5.01900727455947,4.67477377875648));
#11684=CARTESIAN_POINT('Ctrl Pts',(-1.52637072166629,4.90771296889318,4.69728779832826));
#11685=CARTESIAN_POINT('Ctrl Pts',(-1.68892084205195,4.85417329852926,4.70645525547616));
#11686=CARTESIAN_POINT('Ctrl Pts',(-2.06368333503849,4.70962916299031,4.72823993300734));
#11687=CARTESIAN_POINT('Ctrl Pts',(-2.27303626942172,4.61223368350821,4.74091588948176));
#11688=CARTESIAN_POINT('Ctrl Pts',(-2.61214544964475,4.42575936469761,4.76212237131582));
#11689=CARTESIAN_POINT('Ctrl Pts',(-2.74564892399965,4.34419877776501,4.77066563807934));
#11690=CARTESIAN_POINT('Ctrl Pts',(-3.02169087439151,4.15774272360441,4.78877284425884));
#11691=CARTESIAN_POINT('Ctrl Pts',(-3.16295473596736,4.0513157868866,4.79831156670103));
#11692=CARTESIAN_POINT('Ctrl Pts',(-3.48314291991241,3.78311500025063,4.82076344299472));
#11693=CARTESIAN_POINT('Ctrl Pts',(-3.65671817672521,3.6156125077955,4.83361016214211));
#11694=CARTESIAN_POINT('Ctrl Pts',(-3.84598987714552,3.40533786809132,4.84886791552904));
#11695=CARTESIAN_POINT('Ctrl Pts',(-3.87370096498165,3.37378199019494,4.85113703712899));
#11696=CARTESIAN_POINT('Ctrl Pts',(-3.98090387010537,3.24864296469522,4.86006480280909));
#11697=CARTESIAN_POINT('Ctrl Pts',(-4.05741527366864,3.15256352653649,4.86677141894919));
#11698=CARTESIAN_POINT('Ctrl Pts',(-4.18633789524806,2.97819171682413,4.87864837273494));
#11699=CARTESIAN_POINT('Ctrl Pts',(-4.24016636135774,2.90103992224406,4.8838080587719));
#11700=CARTESIAN_POINT('Ctrl Pts',(-4.29183618112783,2.82247103738233,4.88896334675683));
#11701=CARTESIAN_POINT('',(-5.13651484023392,0.000115948992882031,2.82404150530312));
#11702=CARTESIAN_POINT('Ctrl Pts',(-4.29183634723918,2.82247078479419,4.41198748894216));
#11703=CARTESIAN_POINT('Ctrl Pts',(-4.16698587373161,3.01231785178831,4.39953110282041));
#11704=CARTESIAN_POINT('Ctrl Pts',(-4.02963071635437,3.19374075290447,4.38712197081976));
#11705=CARTESIAN_POINT('Ctrl Pts',(-3.73612956550945,3.53216556002768,4.36285766398529));
#11706=CARTESIAN_POINT('Ctrl Pts',(-3.58102114042954,3.68932890567501,4.35102484059281));
#11707=CARTESIAN_POINT('Ctrl Pts',(-3.27604092772345,3.9609375593332,4.32912928924372));
#11708=CARTESIAN_POINT('Ctrl Pts',(-3.12905114971264,4.07805185788519,4.31907839854511));
#11709=CARTESIAN_POINT('Ctrl Pts',(-2.86662554369391,4.26458197742617,4.30163415571333));
#11710=CARTESIAN_POINT('Ctrl Pts',(-2.75426752523295,4.33799611961743,4.29430067500792));
#11711=CARTESIAN_POINT('Ctrl Pts',(-2.36678203900346,4.57004881472384,4.26955374984683));
#11712=CARTESIAN_POINT('Ctrl Pts',(-2.0798511784439,4.70757177577128,4.25215848700385));
#11713=CARTESIAN_POINT('Ctrl Pts',(-1.70962682491867,4.84451661825589,4.230785323076));
#11714=CARTESIAN_POINT('Ctrl Pts',(-1.63659713314603,4.86967300144542,4.22661547558092));
#11715=CARTESIAN_POINT('Ctrl Pts',(-1.38834792646372,4.94897130409852,4.21257524180766));
#11716=CARTESIAN_POINT('Ctrl Pts',(-1.21080523780386,4.99537568940815,4.20276111010223));
#11717=CARTESIAN_POINT('Ctrl Pts',(-0.879696229489418,5.06322427581663,
4.18463390673299));
#11718=CARTESIAN_POINT('Ctrl Pts',(-0.726909371012189,5.08740668869004,
4.17633464143379));
#11719=CARTESIAN_POINT('Ctrl Pts',(-0.413174559980931,5.12263998239836,
4.15920153610614));
#11720=CARTESIAN_POINT('Ctrl Pts',(-0.252326397011973,5.13307739963098,
4.1503748936816));
#11721=CARTESIAN_POINT('Ctrl Pts',(0.159466251844732,5.1403942378555,4.12779133029774));
#11722=CARTESIAN_POINT('Ctrl Pts',(0.410184079607603,5.12648380152769,4.11406728356203));
#11723=CARTESIAN_POINT('Ctrl Pts',(0.865980866247116,5.0675323422528,4.08913561064054));
#11724=CARTESIAN_POINT('Ctrl Pts',(1.07125366947234,5.02814330520748,4.07790960016148));
#11725=CARTESIAN_POINT('Ctrl Pts',(1.49674222504323,4.91925150846555,4.0543512741899));
#11726=CARTESIAN_POINT('Ctrl Pts',(1.71582365701268,4.84718657241992,4.04205190831842));
#11727=CARTESIAN_POINT('Ctrl Pts',(1.96623131618516,4.74570553105891,4.02739561684172));
#11728=CARTESIAN_POINT('Ctrl Pts',(2.0029648951508,4.7303190338737,4.02522967903795));
#11729=CARTESIAN_POINT('Ctrl Pts',(2.25290352949564,4.62219452969925,4.01038947628906));
#11730=CARTESIAN_POINT('Ctrl Pts',(2.45977724820779,4.51550131852102,3.99760448772146));
#11731=CARTESIAN_POINT('Ctrl Pts',(2.81626101730516,4.29985809873201,3.97480838910817));
#11732=CARTESIAN_POINT('Ctrl Pts',(2.96857560114251,4.19614907219953,3.96478664594098));
#11733=CARTESIAN_POINT('Ctrl Pts',(3.25390099252848,3.97854826481852,3.94537614251492));
#11734=CARTESIAN_POINT('Ctrl Pts',(3.38731432460225,3.86559452496691,3.93599324912956));
#11735=CARTESIAN_POINT('Ctrl Pts',(3.67449138419474,3.59615281646616,3.91487387141684));
#11736=CARTESIAN_POINT('Ctrl Pts',(3.82451057584409,3.43617770224084,3.90316984683769));
#11737=CARTESIAN_POINT('Ctrl Pts',(4.0637518660067,3.14591651354651,3.88277721021179));
#11738=CARTESIAN_POINT('Ctrl Pts',(4.15803636699966,3.02019896117357,3.87417745955817));
#11739=CARTESIAN_POINT('Ctrl Pts',(4.3997437315395,2.66509164186776,3.8506260579924));
#11740=CARTESIAN_POINT('Ctrl Pts',(4.53491116777309,2.42797140819965,3.83570852024841));
#11741=CARTESIAN_POINT('Ctrl Pts',(4.75000089237087,1.96937922115244,3.80824994901112));
#11742=CARTESIAN_POINT('Ctrl Pts',(4.83477841364186,1.75096650678446,3.79569685530856));
#11743=CARTESIAN_POINT('Ctrl Pts',(4.95958572779056,1.35025425526063,3.77319528924216));
#11744=CARTESIAN_POINT('Ctrl Pts',(5.00514791860923,1.17011498450273,3.76325692924003));
#11745=CARTESIAN_POINT('Ctrl Pts',(5.06639688980398,0.857588889998009,3.74600288246298));
#11746=CARTESIAN_POINT('Ctrl Pts',(5.08687320653975,0.726330247355653,3.73874509430522));
#11747=CARTESIAN_POINT('Ctrl Pts',(5.13928545762581,0.276453311367826,3.71393041820706));
#11748=CARTESIAN_POINT('Ctrl Pts',(5.14652589683625,-0.0442993161981663,
3.69638975855686));
#11749=CARTESIAN_POINT('Ctrl Pts',(5.108016425025,-0.58691963264991,3.66693741023549));
#11750=CARTESIAN_POINT('Ctrl Pts',(5.07759223039183,-0.808928934359862,
3.65493683317251));
#11751=CARTESIAN_POINT('Ctrl Pts',(4.99516043005286,-1.21239359879457,3.63285918260659));
#11752=CARTESIAN_POINT('Ctrl Pts',(4.94745981875735,-1.39433307262257,3.62279567306552));
#11753=CARTESIAN_POINT('Ctrl Pts',(4.83782946207367,-1.73508183596097,3.60337688120331));
#11754=CARTESIAN_POINT('Ctrl Pts',(4.77775958408615,-1.89423194031333,3.59405930115639));
#11755=CARTESIAN_POINT('Ctrl Pts',(4.61039790601261,-2.27872810951186,3.57106458514552));
#11756=CARTESIAN_POINT('Ctrl Pts',(4.49436913243882,-2.49980429798838,3.5574236828366));
#11757=CARTESIAN_POINT('Ctrl Pts',(4.2445622392266,-2.90172598993572,3.53176094077151));
#11758=CARTESIAN_POINT('Ctrl Pts',(4.11407563818438,-3.0839433985168,3.51973991424205));
#11759=CARTESIAN_POINT('Ctrl Pts',(3.8424509966675,-3.41519978376224,3.49676985460789));
#11760=CARTESIAN_POINT('Ctrl Pts',(3.70346093812589,-3.56544432361029,3.48583597099365));
#11761=CARTESIAN_POINT('Ctrl Pts',(3.45062776303413,-3.80797106325528,3.4668465739468));
#11762=CARTESIAN_POINT('Ctrl Pts',(3.34111544225883,-3.90441052517542,3.4588664696661));
#11763=CARTESIAN_POINT('Ctrl Pts',(2.99640171948637,-4.18283883486137,3.43457788345979));
#11764=CARTESIAN_POINT('Ctrl Pts',(2.74936951454945,-4.34919983472328,3.41830041235499));
#11765=CARTESIAN_POINT('Ctrl Pts',(2.29643071437254,-4.60013486452377,3.39025324662284));
#11766=CARTESIAN_POINT('Ctrl Pts',(2.09684128391969,-4.69447483070205,3.37842315012932));
#11767=CARTESIAN_POINT('Ctrl Pts',(1.71711198229436,-4.84489768070246,3.35652514904728));
#11768=CARTESIAN_POINT('Ctrl Pts',(1.53875640268628,-4.90446055851283,3.34646910037956));
#11769=CARTESIAN_POINT('Ctrl Pts',(1.22808443090893,-4.98959188421171,3.32901608696968));
#11770=CARTESIAN_POINT('Ctrl Pts',(1.09728773392296,-5.01997775425295,3.32167908404949));
#11771=CARTESIAN_POINT('Ctrl Pts',(0.653736807702905,-5.10485600200475,
3.29693522931891));
#11772=CARTESIAN_POINT('Ctrl Pts',(0.337151974305867,-5.13549069809148,
3.27954664739659));
#11773=CARTESIAN_POINT('Ctrl Pts',(-0.199632914229041,-5.13755619757714,
3.25048221337806));
#11774=CARTESIAN_POINT('Ctrl Pts',(-0.418862162275425,-5.12434326013654,
3.23871619197176));
#11775=CARTESIAN_POINT('Ctrl Pts',(-0.817528766906801,-5.07455433896842,
3.2171764094075));
#11776=CARTESIAN_POINT('Ctrl Pts',(-0.997146294888052,-5.04233596897738,
3.20741403073825));
#11777=CARTESIAN_POINT('Ctrl Pts',(-1.30194277429408,-4.97073825333411,
3.19045290852861));
#11778=CARTESIAN_POINT('Ctrl Pts',(-1.42802884969813,-4.93599289859468,
3.18330897824713));
#11779=CARTESIAN_POINT('Ctrl Pts',(-1.86169327647025,-4.79848000757839,
3.15838573140533));
#11780=CARTESIAN_POINT('Ctrl Pts',(-2.16077584673093,-4.67144197549698,
3.14061949307602));
#11781=CARTESIAN_POINT('Ctrl Pts',(-2.64063244514378,-4.41161041848959,
3.11107762533365));
#11782=CARTESIAN_POINT('Ctrl Pts',(-2.82835650920064,-4.29367535017223,
3.09920402644515));
#11783=CARTESIAN_POINT('Ctrl Pts',(-3.16139176043437,-4.05310536390033,
3.07717800486347));
#11784=CARTESIAN_POINT('Ctrl Pts',(-3.30864704724423,-3.93381660329622,
3.06703937154162));
#11785=CARTESIAN_POINT('Ctrl Pts',(-3.57475728552765,-3.6927116017888,3.04755782221915));
#11786=CARTESIAN_POINT('Ctrl Pts',(-3.69481074735828,-3.57258737928862,
3.03825541100929));
#11787=CARTESIAN_POINT('Ctrl Pts',(-3.98081182979747,-3.2565525159005,3.01488278264972));
#11788=CARTESIAN_POINT('Ctrl Pts',(-4.13844413358835,-3.05373256130016,
3.00085247389584));
#11789=CARTESIAN_POINT('Ctrl Pts',(-4.36438680493656,-2.71320434173564,
2.97870184272605));
#11790=CARTESIAN_POINT('Ctrl Pts',(-4.44283307788045,-2.58274764502386,
2.97050522314688));
#11791=CARTESIAN_POINT('Ctrl Pts',(-4.64062278389246,-2.21807044518969,
2.94822104182528));
#11792=CARTESIAN_POINT('Ctrl Pts',(-4.74796938175079,-1.97787719972954,
2.93422696338568));
#11793=CARTESIAN_POINT('Ctrl Pts',(-4.8654627302989,-1.64950862658489,2.91533902401815));
#11794=CARTESIAN_POINT('Ctrl Pts',(-4.89241326820209,-1.56776852310285,
2.91065129160068));
#11795=CARTESIAN_POINT('Ctrl Pts',(-5.01082735890465,-1.17576598720495,
2.88827250409072));
#11796=CARTESIAN_POINT('Ctrl Pts',(-5.07490678563656,-0.857988966175358,
2.87049172435325));
#11797=CARTESIAN_POINT('Ctrl Pts',(-5.12738307900252,-0.358112429451637,
2.84319159551417));
#11798=CARTESIAN_POINT('Ctrl Pts',(-5.13675378971372,-0.179064674554883,
2.83353163990953));
#11799=CARTESIAN_POINT('Ctrl Pts',(-5.13674999885029,0.000108680878606257,
2.82390612103021));
#11800=CARTESIAN_POINT('Ctrl Pts',(-5.13651484023392,0.000115948992882031,
2.82404150530312));
#11801=CARTESIAN_POINT('Ctrl Pts',(-5.13674462019434,0.2777253544017,2.80899084758333));
#11802=CARTESIAN_POINT('Ctrl Pts',(-5.05737420441865,1.27372684428605,2.75498534635027));
#11803=CARTESIAN_POINT('Ctrl Pts',(-4.68610612556516,2.22198890685184,2.70097984511722));
#11804=CARTESIAN_POINT('Ctrl Pts',(-4.29199677360937,2.82257643420045,2.66202500160396));
#11805=CARTESIAN_POINT('Origin',(0.,0.,0.));
#11806=CARTESIAN_POINT('',(-4.29183622825303,2.82247096572397,0.912017191992546));
#11807=CARTESIAN_POINT('',(-4.29183622715607,2.82247096739201,1.38870419915418));
#11808=CARTESIAN_POINT('',(-4.29183622825304,2.82247096572397,0.));
#11809=CARTESIAN_POINT('',(3.87994761181451,-3.36633437021263,0.));
#11810=CARTESIAN_POINT('Ctrl Pts',(-4.29183622825303,2.82247096572397,0.912017191992546));
#11811=CARTESIAN_POINT('Ctrl Pts',(-4.21008100390854,2.94678757976597,0.903950966471187));
#11812=CARTESIAN_POINT('Ctrl Pts',(-4.12291891447378,3.06755243451359,0.895884740949828));
#11813=CARTESIAN_POINT('Ctrl Pts',(-4.03068457529414,3.18430250086042,0.887818515428468));
#11814=CARTESIAN_POINT('Ctrl Pts',(-3.93845155802828,3.30105089393108,0.879752405513235));
#11815=CARTESIAN_POINT('Ctrl Pts',(-3.84114664385558,3.41378435569289,0.871686295598001));
#11816=CARTESIAN_POINT('Ctrl Pts',(-3.73914516075628,3.52207240545859,0.863620185682768));
#11817=CARTESIAN_POINT('Ctrl Pts',(-3.63712168518292,3.63038380314095,0.855552336638772));
#11818=CARTESIAN_POINT('Ctrl Pts',(-3.53039984594936,3.73424763421122,0.847484487594775));
#11819=CARTESIAN_POINT('Ctrl Pts',(-3.41939267200455,3.83326940315204,0.839416638550779));
#11820=CARTESIAN_POINT('Ctrl Pts',(-3.39302187999351,3.85679295014912,0.837500045581558));
#11821=CARTESIAN_POINT('Ctrl Pts',(-3.36640940475421,3.88004340779256,0.835583452612338));
#11822=CARTESIAN_POINT('Ctrl Pts',(-3.33956107133174,3.90301581003019,0.833666859643117));
#11823=CARTESIAN_POINT('Ctrl Pts',(-3.22653862334114,3.99972189216443,0.825598648265736));
#11824=CARTESIAN_POINT('Ctrl Pts',(-3.10929183836299,4.09153327460306,0.817530436888356));
#11825=CARTESIAN_POINT('Ctrl Pts',(-2.9882666781965,4.17809320413995,0.809462225510975));
#11826=CARTESIAN_POINT('Ctrl Pts',(-2.86726598957703,4.2646356310734,0.801395645543243));
#11827=CARTESIAN_POINT('Ctrl Pts',(-2.74248871904446,4.34592853107688,0.793329065575511));
#11828=CARTESIAN_POINT('Ctrl Pts',(-2.61441152346859,4.42165726266234,0.785262485607779));
#11829=CARTESIAN_POINT('Ctrl Pts',(-2.4863297736047,4.49738868708047,0.777195618801096));
#11830=CARTESIAN_POINT('Ctrl Pts',(-2.35494814688641,4.56755537541207,0.769128751994412));
#11831=CARTESIAN_POINT('Ctrl Pts',(-2.22077020889626,4.63188733042794,0.761061885187729));
#11832=CARTESIAN_POINT('Ctrl Pts',(-2.08660042131369,4.69621537771008,0.752995508388966));
#11833=CARTESIAN_POINT('Ctrl Pts',(-1.94963496112967,4.75470925833884,0.744929131590202));
#11834=CARTESIAN_POINT('Ctrl Pts',(-1.81039978902733,4.8071460521176,0.736862754791439));
#11835=CARTESIAN_POINT('Ctrl Pts',(-1.6711299114841,4.85959591617177,0.728794367386024));
#11836=CARTESIAN_POINT('Ctrl Pts',(-1.52958950126482,4.90598555920214,0.720725979980609));
#11837=CARTESIAN_POINT('Ctrl Pts',(-1.38632283533957,4.9461408753407,0.712657592575194));
#11838=CARTESIAN_POINT('Ctrl Pts',(-1.2801670636738,4.9758946114498,0.706679189395441));
#11839=CARTESIAN_POINT('Ctrl Pts',(-1.17306391967465,5.00222651706419,0.700700786215688));
#11840=CARTESIAN_POINT('Ctrl Pts',(-1.06523962154578,5.02508359245784,0.694722383035935));
#11841=CARTESIAN_POINT('Ctrl Pts',(-0.919691791466988,5.0559374703242,0.686652368899518));
#11842=CARTESIAN_POINT('Ctrl Pts',(-0.772775968558962,5.0804692105179,0.678582354763101));
#11843=CARTESIAN_POINT('Ctrl Pts',(-0.625054704343801,5.0985789372214,0.670512340626684));
#11844=CARTESIAN_POINT('Ctrl Pts',(-0.477363046062251,5.11668503441787,
0.662443943862715));
#11845=CARTESIAN_POINT('Ctrl Pts',(-0.328866596591976,5.12837164570133,
0.654375547098746));
#11846=CARTESIAN_POINT('Ctrl Pts',(-0.180134706237769,5.13359056120652,
0.646307150334778));
#11847=CARTESIAN_POINT('Ctrl Pts',(-0.0313974666155599,5.1388096644144,
0.638238463384108));
#11848=CARTESIAN_POINT('Ctrl Pts',(0.11757490046023,5.13756059100852,0.630169776433437));
#11849=CARTESIAN_POINT('Ctrl Pts',(0.266210780156402,5.12984720854613,0.622101089482767));
#11850=CARTESIAN_POINT('Ctrl Pts',(0.414837591449361,5.12213429668385,0.614032894809647));
#11851=CARTESIAN_POINT('Ctrl Pts',(0.563127626181557,5.10795788272256,0.605964700136526));
#11852=CARTESIAN_POINT('Ctrl Pts',(0.710512129098562,5.08737388805893,0.597896505463406));
#11853=CARTESIAN_POINT('Ctrl Pts',(0.857932985422962,5.0667848162106,0.589826320714246));
#11854=CARTESIAN_POINT('Ctrl Pts',(1.0044475358245,5.0397850506676,0.581756135965086));
#11855=CARTESIAN_POINT('Ctrl Pts',(1.14949429669496,5.00648214062187,0.573685951215926));
#11856=CARTESIAN_POINT('Ctrl Pts',(1.25678237706487,4.98184866884977,0.567716602953532));
#11857=CARTESIAN_POINT('Ctrl Pts',(1.36326752836467,4.95376766217731,0.561747254691139));
#11858=CARTESIAN_POINT('Ctrl Pts',(1.46872680677471,4.92230049159551,0.555777906428746));
#11859=CARTESIAN_POINT('Ctrl Pts',(1.61116648069071,4.87979902956858,0.54771534396098));
#11860=CARTESIAN_POINT('Ctrl Pts',(1.751787269433,4.83110249295492,0.539652781493215));
#11861=CARTESIAN_POINT('Ctrl Pts',(1.89004827637476,4.77639174225406,0.531590219025449));
#11862=CARTESIAN_POINT('Ctrl Pts',(2.0282809272638,4.72169221222174,0.523529310114616));
#11863=CARTESIAN_POINT('Ctrl Pts',(2.16415445337024,4.66098105087857,0.515468401203782));
#11864=CARTESIAN_POINT('Ctrl Pts',(2.29714668271859,4.59448774952932,0.507407492292949));
#11865=CARTESIAN_POINT('Ctrl Pts',(2.43014400301256,4.52799190281495,0.499346274810335));
#11866=CARTESIAN_POINT('Ctrl Pts',(2.56025950722101,4.45571361820597,0.491285057327722));
#11867=CARTESIAN_POINT('Ctrl Pts',(2.68699393420941,4.37792920911495,0.483223839845109));
#11868=CARTESIAN_POINT('Ctrl Pts',(2.81372104560421,4.30014929003614,0.475163087686658));
#11869=CARTESIAN_POINT('Ctrl Pts',(2.93706718779034,4.21686405679972,0.467102335528207));
#11870=CARTESIAN_POINT('Ctrl Pts',(3.05656051392089,4.1283941656823,0.459041583369756));
#11871=CARTESIAN_POINT('Ctrl Pts',(3.17608499704292,4.03990120670215,0.450978729430441));
#11872=CARTESIAN_POINT('Ctrl Pts',(3.29175438943587,3.94622108570467,0.442915875491126));
#11873=CARTESIAN_POINT('Ctrl Pts',(3.40312793024007,3.84771631658571,0.434853021551811));
#11874=CARTESIAN_POINT('Ctrl Pts',(3.48609713485625,3.77433387506786,0.428846490975061));
#11875=CARTESIAN_POINT('Ctrl Pts',(3.56668289912837,3.69827477537264,0.42283996039831));
#11876=CARTESIAN_POINT('Ctrl Pts',(3.6447156174895,3.61970283726829,0.41683342982156));
#11877=CARTESIAN_POINT('Ctrl Pts',(3.74970717869758,3.51398576599388,0.408751755417004));
#11878=CARTESIAN_POINT('Ctrl Pts',(3.85011415322258,3.40367942648003,0.400670081012447));
#11879=CARTESIAN_POINT('Ctrl Pts',(3.94554677348586,3.28920373658053,0.392588406607891));
#11880=CARTESIAN_POINT('Ctrl Pts',(4.04096069636049,3.17475047503371,0.384508315584434));
#11881=CARTESIAN_POINT('Ctrl Pts',(4.13140199903371,3.0561297452835,0.376428224560978));
#11882=CARTESIAN_POINT('Ctrl Pts',(4.2165206596561,2.93379516824084,0.368348133537521));
#11883=CARTESIAN_POINT('Ctrl Pts',(4.30164168937171,2.81145718628068,0.360267817622264));
#11884=CARTESIAN_POINT('Ctrl Pts',(4.38143958971418,2.68540541788936,0.352187501707008));
#11885=CARTESIAN_POINT('Ctrl Pts',(4.45560688104378,2.55612360501118,0.344107185791751));
#11886=CARTESIAN_POINT('Ctrl Pts',(4.52976906939097,2.42685068719719,0.336027425831946));
#11887=CARTESIAN_POINT('Ctrl Pts',(4.59830126053746,2.29434845491385,0.327947665872142));
#11888=CARTESIAN_POINT('Ctrl Pts',(4.6609412589197,2.15912647693462,0.319867905912338));
#11889=CARTESIAN_POINT('Ctrl Pts',(4.7235950620254,2.02387469847547,0.311786365319474));
#11890=CARTESIAN_POINT('Ctrl Pts',(4.78035393865719,1.88590227475489,0.30370482472661));
#11891=CARTESIAN_POINT('Ctrl Pts',(4.83100301207731,1.74574066224051,0.295623284133747));
#11892=CARTESIAN_POINT('Ctrl Pts',(4.86805153512688,1.64321596867247,0.289711840493955));
#11893=CARTESIAN_POINT('Ctrl Pts',(4.90183195686734,1.53952040512254,0.283800396854164));
#11894=CARTESIAN_POINT('Ctrl Pts',(4.9322768395638,1.43486784771369,0.277888953214373));
#11895=CARTESIAN_POINT('Ctrl Pts',(4.97370082733191,1.29247523936544,0.269845710891254));
#11896=CARTESIAN_POINT('Ctrl Pts',(5.00896290811795,1.14825843281626,0.261802468568135));
#11897=CARTESIAN_POINT('Ctrl Pts',(5.03792200991058,1.0027673631299,0.253759226245016));
#11898=CARTESIAN_POINT('Ctrl Pts',(5.06687513239429,0.857306333603579,0.245717644644352));
#11899=CARTESIAN_POINT('Ctrl Pts',(5.08952780654059,0.71057189423708,0.237676063043689));
#11900=CARTESIAN_POINT('Ctrl Pts',(5.10578996746797,0.563124649259317,0.229634481443026));
#11901=CARTESIAN_POINT('Ctrl Pts',(5.12205310316367,0.415668566163129,0.221592417822841));
#11902=CARTESIAN_POINT('Ctrl Pts',(5.13192491885463,0.267499924669364,0.213550354202656));
#11903=CARTESIAN_POINT('Ctrl Pts',(5.13536711260807,0.119185490909914,0.205508290582471));
#11904=CARTESIAN_POINT('Ctrl Pts',(5.13880916577307,-0.0291228852895836,
0.197466555421771));
#11905=CARTESIAN_POINT('Ctrl Pts',(5.13582211635772,-0.177576706738936,
0.189424820261071));
#11906=CARTESIAN_POINT('Ctrl Pts',(5.12641978813453,-0.325608228278663,
0.181383085100371));
#11907=CARTESIAN_POINT('Ctrl Pts',(5.1170145447799,-0.473685646040024,0.17333885665138));
#11908=CARTESIAN_POINT('Ctrl Pts',(5.10119006912052,-0.621340167588099,
0.16529462820239));
#11909=CARTESIAN_POINT('Ctrl Pts',(5.07901221185679,-0.76800749625874,0.1572503997534));
#11910=CARTESIAN_POINT('Ctrl Pts',(5.06218912960214,-0.879262452269773,
0.151148425371328));
#11911=CARTESIAN_POINT('Ctrl Pts',(5.04171136380057,-0.989949420781112,
0.145046450989256));
#11912=CARTESIAN_POINT('Ctrl Pts',(5.01762739212586,-1.0998254026382,0.138944476607185));
#11913=CARTESIAN_POINT('Ctrl Pts',(4.98558682514019,-1.24600099212803,0.130826599640121));
#11914=CARTESIAN_POINT('Ctrl Pts',(4.94714925029851,-1.3907987628262,0.122708722673057));
#11915=CARTESIAN_POINT('Ctrl Pts',(4.902457660558,-1.53365884372509,0.114590845705993));
#11916=CARTESIAN_POINT('Ctrl Pts',(4.85777553300864,-1.67648867800708,0.106474687471783));
#11917=CARTESIAN_POINT('Ctrl Pts',(4.80684212893725,-1.81738133333755,0.0983585292375734));
#11918=CARTESIAN_POINT('Ctrl Pts',(4.74985030595653,-1.95579207317768,0.0902423710033638));
#11919=CARTESIAN_POINT('Ctrl Pts',(4.6928610457974,-2.09419658893137,0.0821265777384509));
#11920=CARTESIAN_POINT('Ctrl Pts',(4.62981402997828,-2.23011911229002,0.074010784473538));
#11921=CARTESIAN_POINT('Ctrl Pts',(4.56095048152956,-2.36303433481937,0.0658949912086251));
#11922=CARTESIAN_POINT('Ctrl Pts',(4.49209525369898,-2.49593349751974,0.0577801785556347));
#11923=CARTESIAN_POINT('Ctrl Pts',(4.41742504594519,-2.62582579900045,0.0496653659026443));
#11924=CARTESIAN_POINT('Ctrl Pts',(4.33722738088866,-2.75220987734761,0.0415505532496539));
#11925=CARTESIAN_POINT('Ctrl Pts',(4.2570221515381,-2.87860587632023,0.0334349752024494));
#11926=CARTESIAN_POINT('Ctrl Pts',(4.17128859463849,-3.0014927176085,0.025319397155245));
#11927=CARTESIAN_POINT('Ctrl Pts',(4.08035831595364,-3.12039686192766,0.0172038191080405));
#11928=CARTESIAN_POINT('Ctrl Pts',(4.01610542450468,-3.20441656568607,0.0114692127386931));
#11929=CARTESIAN_POINT('Ctrl Pts',(3.94925869462562,-3.28644825652029,0.00573460636934572));
#11930=CARTESIAN_POINT('Ctrl Pts',(3.87994761181449,-3.36633437021265,-1.66533453693773E-15));
#11931=CARTESIAN_POINT('',(-3.87712761685009,-3.36958187393604,0.));
#11932=CARTESIAN_POINT('Origin',(0.,0.,0.));
#11933=CARTESIAN_POINT('Ctrl Pts',(-3.87712761685009,-3.36958187393604,
4.49727061146987E-15));
#11934=CARTESIAN_POINT('Ctrl Pts',(-3.67794676588939,-3.59876448676431,
0.0165613539089372));
#11935=CARTESIAN_POINT('Ctrl Pts',(-3.45883402269643,-3.80983897824898,
0.0332733431119535));
#11936=CARTESIAN_POINT('Ctrl Pts',(-3.09258329567885,-4.10486285593889,
0.0588935811804499));
#11937=CARTESIAN_POINT('Ctrl Pts',(-2.95779534839617,-4.2030249769505,0.0679145294576286));
#11938=CARTESIAN_POINT('Ctrl Pts',(-2.60936178549079,-4.43170327237994,
0.0903703299745524));
#11939=CARTESIAN_POINT('Ctrl Pts',(-2.39050720159611,-4.55348631775,0.103712854959601));
#11940=CARTESIAN_POINT('Ctrl Pts',(-2.09063362584706,-4.69275331719403,
0.121499195248639));
#11941=CARTESIAN_POINT('Ctrl Pts',(-2.01682637619907,-4.72494377940485,
0.125841126992301));
#11942=CARTESIAN_POINT('Ctrl Pts',(-1.70233581227173,-4.85339458642629,
0.144261136625014));
#11943=CARTESIAN_POINT('Ctrl Pts',(-1.45530622128663,-4.93309916368872,
0.15852273649863));
#11944=CARTESIAN_POINT('Ctrl Pts',(-1.05527656046196,-5.02949121427313,
0.181051295485889));
#11945=CARTESIAN_POINT('Ctrl Pts',(-0.905716505943988,-5.05856396129082,
0.18935829443773));
#11946=CARTESIAN_POINT('Ctrl Pts',(-0.432678787318127,-5.12886250479386,
0.215312816039704));
#11947=CARTESIAN_POINT('Ctrl Pts',(-0.106443458305649,-5.14598048110269,
0.23270696890385));
#11948=CARTESIAN_POINT('Ctrl Pts',(0.34892233957708,-5.12652994874249,0.257173627398254));
#11949=CARTESIAN_POINT('Ctrl Pts',(0.478373500791217,-5.11607409352535,
0.264158391034179));
#11950=CARTESIAN_POINT('Ctrl Pts',(0.78908104089943,-5.07908146218344,0.281151389956572));
#11951=CARTESIAN_POINT('Ctrl Pts',(0.96958390305285,-5.04773442969581,0.291195520648721));
#11952=CARTESIAN_POINT('Ctrl Pts',(1.36146745708136,-4.95787856096829,0.3132413220559));
#11953=CARTESIAN_POINT('Ctrl Pts',(1.57156576091593,-4.89533837737919,0.32521413130658));
#11954=CARTESIAN_POINT('Ctrl Pts',(2.0737784553686,-4.7101669225529,0.35425942983852));
#11955=CARTESIAN_POINT('Ctrl Pts',(2.35978606958852,-4.57358099099414,0.371147635061239));
#11956=CARTESIAN_POINT('Ctrl Pts',(2.74718951566983,-4.34250195081651,0.39535775583837));
#11957=CARTESIAN_POINT('Ctrl Pts',(2.86019893378217,-4.26891491972748,0.402607010498784));
#11958=CARTESIAN_POINT('Ctrl Pts',(3.12348935838074,-4.08231830347208,0.420129907503093));
#11959=CARTESIAN_POINT('Ctrl Pts',(3.27071744966058,-3.9653391051075,0.430440616113486));
#11960=CARTESIAN_POINT('Ctrl Pts',(3.5761028785873,-3.69409428874524,0.452836388923162));
#11961=CARTESIAN_POINT('Ctrl Pts',(3.73140140671969,-3.53715866168108,0.464891535223208));
#11962=CARTESIAN_POINT('Ctrl Pts',(4.07122465605871,-3.1463822001139,0.492982350425229));
#11963=CARTESIAN_POINT('Ctrl Pts',(4.24647224751272,-2.90552378445464,0.508873916678694));
#11964=CARTESIAN_POINT('Ctrl Pts',(4.47517449491686,-2.52592336704837,0.532648208012569));
#11965=CARTESIAN_POINT('Ctrl Pts',(4.5450895460534,-2.3978397412183,0.540483436976261));
#11966=CARTESIAN_POINT('Ctrl Pts',(4.69981111166034,-2.08324053907106,0.559513082360392));
#11967=CARTESIAN_POINT('Ctrl Pts',(4.7790983621461,-1.89428947067627,0.570754490415751));
#11968=CARTESIAN_POINT('Ctrl Pts',(4.92097365448571,-1.49005160546221,0.594240358157978));
#11969=CARTESIAN_POINT('Ctrl Pts',(4.98118627467262,-1.27437144825174,0.60645373847293));
#11970=CARTESIAN_POINT('Ctrl Pts',(5.07824358872919,-0.812084167476704,
0.632046342522596));
#11971=CARTESIAN_POINT('Ctrl Pts',(5.11159934270931,-0.565326300837397,
0.645366656085126));
#11972=CARTESIAN_POINT('Ctrl Pts',(5.13765208327986,-0.144128238859615,
0.667992630281884));
#11973=CARTESIAN_POINT('Ctrl Pts',(5.13958963906823,0.0292932019941339,
0.677282382789924));
#11974=CARTESIAN_POINT('Ctrl Pts',(5.12576156181907,0.37983320139103,0.696314066716988));
#11975=CARTESIAN_POINT('Ctrl Pts',(5.10957748483041,0.556705551840665,0.706045732276116));
#11976=CARTESIAN_POINT('Ctrl Pts',(5.06771091843579,0.84734760871232,0.722147861276686));
#11977=CARTESIAN_POINT('Ctrl Pts',(5.04725554703136,0.961719111476853,0.728514237713954));
#11978=CARTESIAN_POINT('Ctrl Pts',(5.00598998697943,1.15447891712609,0.739288911459822));
#11979=CARTESIAN_POINT('Ctrl Pts',(4.98716938784524,1.2332473419332,0.743704999132241));
#11980=CARTESIAN_POINT('Ctrl Pts',(4.92248900032307,1.47817709710584,0.757484618818292));
#11981=CARTESIAN_POINT('Ctrl Pts',(4.87012408715872,1.64249771726079,0.766795339539799));
#11982=CARTESIAN_POINT('Ctrl Pts',(4.70270011315783,2.08889280222995,0.792441569914432));
#11983=CARTESIAN_POINT('Ctrl Pts',(4.57068198165357,2.36383590570105,0.808618117485238));
#11984=CARTESIAN_POINT('Ctrl Pts',(4.31814811777889,2.78850886561886,0.835411388137797));
#11985=CARTESIAN_POINT('Ctrl Pts',(4.21223646506265,2.94605612110679,0.845816787543465));
#11986=CARTESIAN_POINT('Ctrl Pts',(3.96318555833698,3.27555214221487,0.868465063416418));
#11987=CARTESIAN_POINT('Ctrl Pts',(3.81703550485156,3.44475326201248,0.880678412879389));
#11988=CARTESIAN_POINT('Ctrl Pts',(3.43755738543845,3.83017319014098,0.910028833770194));
#11989=CARTESIAN_POINT('Ctrl Pts',(3.19427763230978,4.03529697831146,0.926982737569991));
#11990=CARTESIAN_POINT('Ctrl Pts',(2.82350049240882,4.29325522727336,0.951225207217467));
#11991=CARTESIAN_POINT('Ctrl Pts',(2.71042732998981,4.36552153642016,0.958439225669647));
#11992=CARTESIAN_POINT('Ctrl Pts',(2.43253339794523,4.52816395244855,0.975923313940613));
#11993=CARTESIAN_POINT('Ctrl Pts',(2.26532985933429,4.61408349444963,0.986230991954779));
#11994=CARTESIAN_POINT('Ctrl Pts',(1.89239357250138,4.78055372433496,1.00862415092931));
#11995=CARTESIAN_POINT('Ctrl Pts',(1.68540303190607,4.85739306715182,1.02067970430198));
#11996=CARTESIAN_POINT('Ctrl Pts',(1.18934426571286,5.00599954024447,1.04876913223415));
#11997=CARTESIAN_POINT('Ctrl Pts',(0.89770629447462,5.06642856938913,1.06465896497858));
#11998=CARTESIAN_POINT('Ctrl Pts',(0.457631110645011,5.11840288465141,1.08843129162848));
#11999=CARTESIAN_POINT('Ctrl Pts',(0.312122433197049,5.129332578545,1.09626630778173));
#12000=CARTESIAN_POINT('Ctrl Pts',(-0.0379702776302637,5.14067588196109,
1.1152791392755));
#12001=CARTESIAN_POINT('Ctrl Pts',(-0.242499004021474,5.13509324416503,
1.12650355857268));
#12002=CARTESIAN_POINT('Ctrl Pts',(-0.6692274883726,5.09788958232329,1.14998594167575));
#12003=CARTESIAN_POINT('Ctrl Pts',(-0.890801469099042,5.06387402817349,
1.16221264436448));
#12004=CARTESIAN_POINT('Ctrl Pts',(-1.35077562034394,4.96212585850705,1.18773635945147));
#12005=CARTESIAN_POINT('Ctrl Pts',(-1.58793497065248,4.89139584885384,1.20097686756525));
#12006=CARTESIAN_POINT('Ctrl Pts',(-1.98173820068383,4.74227423996327,1.22355376393861));
#12007=CARTESIAN_POINT('Ctrl Pts',(-2.14115816562501,4.67246088888614,1.23287493450321));
#12008=CARTESIAN_POINT('Ctrl Pts',(-2.45881379811487,4.51367612881655,1.25213847658075));
#12009=CARTESIAN_POINT('Ctrl Pts',(-2.61649813803016,4.42413476899977,1.26207510876547));
#12010=CARTESIAN_POINT('Ctrl Pts',(-2.97860362880383,4.19237199858659,1.28565029941015));
#12011=CARTESIAN_POINT('Ctrl Pts',(-3.17808721282558,4.04324546800822,1.29924846941561));
#12012=CARTESIAN_POINT('Ctrl Pts',(-3.51169963555394,3.75384835361944,1.32318227012894));
#12013=CARTESIAN_POINT('Ctrl Pts',(-3.65018170213261,3.61933521208265,1.33355114534632));
#12014=CARTESIAN_POINT('Ctrl Pts',(-3.92026463845979,3.32568584159246,1.35495200457925));
#12015=CARTESIAN_POINT('Ctrl Pts',(-4.05050341498609,3.16576701487549,1.36596134553038));
#12016=CARTESIAN_POINT('Ctrl Pts',(-4.21235227040537,2.94063944829266,1.38095379298858));
#12017=CARTESIAN_POINT('Ctrl Pts',(-4.25271201107483,2.88196306841854,1.38482184364391));
#12018=CARTESIAN_POINT('Ctrl Pts',(-4.29183622715607,2.82247096739201,1.38870419915418));
#12019=CARTESIAN_POINT('Origin',(0.,0.,0.));
#12020=CARTESIAN_POINT('Ctrl Pts',(-4.29183622715607,2.82247096739201,1.38870419915418));
#12021=CARTESIAN_POINT('Ctrl Pts',(-4.31141166714452,2.79270464438086,1.39064669985879));
#12022=CARTESIAN_POINT('Ctrl Pts',(-4.33067781498162,2.7627340977274,1.39259244493516));
#12023=CARTESIAN_POINT('Ctrl Pts',(-4.51934871643038,2.46241218084559,1.41198450141167));
#12024=CARTESIAN_POINT('Ctrl Pts',(-4.66353332528833,2.17702800889423,1.42951622892346));
#12025=CARTESIAN_POINT('Ctrl Pts',(-4.84874005285254,1.70612859728417,1.45699470652792));
#12026=CARTESIAN_POINT('Ctrl Pts',(-4.90762112400106,1.52853261964258,1.46706850157614));
#12027=CARTESIAN_POINT('Ctrl Pts',(-5.01939924697197,1.11755322245494,1.4899392981333));
#12028=CARTESIAN_POINT('Ctrl Pts',(-5.06594377540955,0.882895526417692,
1.50268213900738));
#12029=CARTESIAN_POINT('Ctrl Pts',(-5.10916066820828,0.541902040532461,
1.52126208035794));
#12030=CARTESIAN_POINT('Ctrl Pts',(-5.11915130749457,0.437572172905712,
1.52696533204475));
#12031=CARTESIAN_POINT('Ctrl Pts',(-5.14036681225492,0.111008979525595,
1.54485261825289));
#12032=CARTESIAN_POINT('Ctrl Pts',(-5.14035198390431,-0.111696981736819,
1.55707921641052));
#12033=CARTESIAN_POINT('Ctrl Pts',(-5.12068037764657,-0.413868710161159,
1.57362677475726));
#12034=CARTESIAN_POINT('Ctrl Pts',(-5.113581257039,-0.493904600531326,1.57800711312869));
#12035=CARTESIAN_POINT('Ctrl Pts',(-5.08520518934513,-0.746367912630681,
1.59182285114144));
#12036=CARTESIAN_POINT('Ctrl Pts',(-5.05705804447842,-0.917901261478106,
1.60120387894329));
#12037=CARTESIAN_POINT('Ctrl Pts',(-4.96805251722242,-1.32871300747945,
1.62380954986378));
#12038=CARTESIAN_POINT('Ctrl Pts',(-4.89854093047065,-1.56566882709781,
1.63695767537244));
#12039=CARTESIAN_POINT('Ctrl Pts',(-4.77768946535749,-1.8893552738304,1.65558489834132));
#12040=CARTESIAN_POINT('Ctrl Pts',(-4.74043272869375,-1.98097878584997,
1.66094358692037));
#12041=CARTESIAN_POINT('Ctrl Pts',(-4.60508239316641,-2.28811419298573,
1.67924125183664));
#12042=CARTESIAN_POINT('Ctrl Pts',(-4.49474713708642,-2.49789882629554,
1.69226091047833));
#12043=CARTESIAN_POINT('Ctrl Pts',(-4.27545647508133,-2.85294114281389,
1.71508529103285));
#12044=CARTESIAN_POINT('Ctrl Pts',(-4.17254040925077,-3.00145131639488,
1.7249075314345));
#12045=CARTESIAN_POINT('Ctrl Pts',(-4.01390746121736,-3.20638813345496,
1.73892180881287));
#12046=CARTESIAN_POINT('Ctrl Pts',(-3.96437763307514,-3.26742836552705,
1.74315998107736));
#12047=CARTESIAN_POINT('Ctrl Pts',(-3.78178821157069,-3.48218379783606,
1.75832959751573));
#12048=CARTESIAN_POINT('Ctrl Pts',(-3.64103255844747,-3.62910568764466,
1.76919264782912));
#12049=CARTESIAN_POINT('Ctrl Pts',(-3.43642165873281,-3.81876125601511,
1.78417592482309));
#12050=CARTESIAN_POINT('Ctrl Pts',(-3.37977137045612,-3.86898909760957,
1.78824820687431));
#12051=CARTESIAN_POINT('Ctrl Pts',(-3.24490383790619,-3.98334347723956,
1.79779907114967));
#12052=CARTESIAN_POINT('Ctrl Pts',(-3.16586326002202,-4.0464472197234,1.80329583339986));
#12053=CARTESIAN_POINT('Ctrl Pts',(-2.97262834866866,-4.19159129141606,
1.81649532033844));
#12054=CARTESIAN_POINT('Ctrl Pts',(-2.85682665152495,-4.27135786086577,
1.82420808002789));
#12055=CARTESIAN_POINT('Ctrl Pts',(-2.55720146267498,-4.46010432807095,
1.843622205695));
#12056=CARTESIAN_POINT('Ctrl Pts',(-2.36957635092301,-4.5625564177526,1.85528941963915));
#12057=CARTESIAN_POINT('Ctrl Pts',(-1.97469236155925,-4.74723460680782,
1.8789303816139));
#12058=CARTESIAN_POINT('Ctrl Pts',(-1.76736133874764,-4.82825880858382,
1.89087141787454));
#12059=CARTESIAN_POINT('Ctrl Pts',(-1.35848056167132,-4.95816861655219,
1.91387638233383));
#12060=CARTESIAN_POINT('Ctrl Pts',(-1.15793765458368,-5.0088005241963,1.92492410092325));
#12061=CARTESIAN_POINT('Ctrl Pts',(-0.810115838898992,-5.07460583021643,
1.94411172691831));
#12062=CARTESIAN_POINT('Ctrl Pts',(-0.664227260001339,-5.09575436093513,
1.95217413987132));
#12063=CARTESIAN_POINT('Ctrl Pts',(-0.224205717253499,-5.14032258787291,
1.97641757494));
#12064=CARTESIAN_POINT('Ctrl Pts',(0.0712459142612628,-5.14471732046345,
1.99256637832505));
#12065=CARTESIAN_POINT('Ctrl Pts',(0.584314172565213,-5.10812354573329,
2.02042862672598));
#12066=CARTESIAN_POINT('Ctrl Pts',(0.801963171469988,-5.07850438433339,
2.0322006848874));
#12067=CARTESIAN_POINT('Ctrl Pts',(1.2032638579666,-4.99744394827057,2.05415079295371));
#12068=CARTESIAN_POINT('Ctrl Pts',(1.38724179637618,-4.94953003756478,2.06431655169254));
#12069=CARTESIAN_POINT('Ctrl Pts',(1.69726933951955,-4.85014079745769,2.08195713025871));
#12070=CARTESIAN_POINT('Ctrl Pts',(1.82470738519257,-4.80364761347787,2.08937006591804));
#12071=CARTESIAN_POINT('Ctrl Pts',(2.24138331453824,-4.63265576006546,2.11404942497428));
#12072=CARTESIAN_POINT('Ctrl Pts',(2.52101923036853,-4.48662121468314,2.13129573017535));
#12073=CARTESIAN_POINT('Ctrl Pts',(2.97281583180695,-4.19502751127474,2.1604123509012));
#12074=CARTESIAN_POINT('Ctrl Pts',(3.15204066944918,-4.06208466874455,2.17236480419372));
#12075=CARTESIAN_POINT('Ctrl Pts',(3.46799012604106,-3.79418624669297,2.19457327312554));
#12076=CARTESIAN_POINT('Ctrl Pts',(3.6068868057623,-3.66239945016972,2.20481540706834));
#12077=CARTESIAN_POINT('Ctrl Pts',(3.85823291506199,-3.39572008051004,2.22469796506014));
#12078=CARTESIAN_POINT('Ctrl Pts',(3.97176141901386,-3.26220564490393,2.23430001569753));
#12079=CARTESIAN_POINT('Ctrl Pts',(4.2262139065245,-2.92993919161391,2.25724918189883));
#12080=CARTESIAN_POINT('Ctrl Pts',(4.36026584482773,-2.72644712183987,2.27056003177417));
#12081=CARTESIAN_POINT('Ctrl Pts',(4.58891772585733,-2.31907561490368,2.29589345796691));
#12082=CARTESIAN_POINT('Ctrl Pts',(4.68558031649715,-2.11698314038772,2.30790920922863));
#12083=CARTESIAN_POINT('Ctrl Pts',(4.84481696450797,-1.71925154252139,2.33088155637874));
#12084=CARTESIAN_POINT('Ctrl Pts',(4.90945504653299,-1.52490174988738,2.34182293582193));
#12085=CARTESIAN_POINT('Ctrl Pts',(5.00003926780489,-1.18621740950124,2.36082543105876));
#12086=CARTESIAN_POINT('Ctrl Pts',(5.03172400004837,-1.04367446005091,2.3688110013006));
#12087=CARTESIAN_POINT('Ctrl Pts',(5.10934922604341,-0.607471373211402,
2.39309649364469));
#12088=CARTESIAN_POINT('Ctrl Pts',(5.13592870127669,-0.310990825811056,
2.40936532209319));
#12089=CARTESIAN_POINT('Ctrl Pts',(5.1373267443539,0.206579087863292,2.43739993271944));
#12090=CARTESIAN_POINT('Ctrl Pts',(5.1237297641605,0.426845181964274,2.44922599880147));
#12091=CARTESIAN_POINT('Ctrl Pts',(5.07239118242162,0.832111030281952,2.47112760193419));
#12092=CARTESIAN_POINT('Ctrl Pts',(5.03853323482339,1.01722241977832,2.48119125524799));
#12093=CARTESIAN_POINT('Ctrl Pts',(4.96322250420805,1.33066374794971,2.49865717613434));
#12094=CARTESIAN_POINT('Ctrl Pts',(4.92673108004532,1.45998732328115,2.50599934816381));
#12095=CARTESIAN_POINT('Ctrl Pts',(4.78717135690065,1.8893925886892,2.53073869295086));
#12096=CARTESIAN_POINT('Ctrl Pts',(4.66139430778449,2.18133596579021,2.54811746667217));
#12097=CARTESIAN_POINT('Ctrl Pts',(4.40405758253498,2.65310297354305,2.57721447167864));
#12098=CARTESIAN_POINT('Ctrl Pts',(4.28630290147522,2.83941691267552,2.58902167958839));
#12099=CARTESIAN_POINT('Ctrl Pts',(4.05037228469111,3.16442773986515,2.61055349693758));
#12100=CARTESIAN_POINT('Ctrl Pts',(3.936086367198,3.30550154142237,2.62026684610574));
#12101=CARTESIAN_POINT('Ctrl Pts',(3.72739054895614,3.53690662520179,2.63714733539855));
#12102=CARTESIAN_POINT('Ctrl Pts',(3.63655980579654,3.63023140921971,2.6442605209355));
#12103=CARTESIAN_POINT('Ctrl Pts',(3.30667633459527,3.94435512283217,2.66921451597319));
#12104=CARTESIAN_POINT('Ctrl Pts',(3.0502789600889,4.14582371024468,2.68704314377013));
#12105=CARTESIAN_POINT('Ctrl Pts',(2.5892076168806,4.44204776925775,2.71671100842295));
#12106=CARTESIAN_POINT('Ctrl Pts',(2.39423586960612,4.55010125589898,2.72864847294603));
#12107=CARTESIAN_POINT('Ctrl Pts',(2.0235080441058,4.72511270438161,2.75062757006997));
#12108=CARTESIAN_POINT('Ctrl Pts',(1.84990692018692,4.79573943034203,2.7606556209678));
#12109=CARTESIAN_POINT('Ctrl Pts',(1.50756783501789,4.9136540143316,2.78029786142779));
#12110=CARTESIAN_POINT('Ctrl Pts',(1.33949838561722,4.96210630219023,2.78988054898158));
#12111=CARTESIAN_POINT('Ctrl Pts',(0.931010247072214,5.05759826221133,2.8128842813617));
#12112=CARTESIAN_POINT('Ctrl Pts',(0.689050509106018,5.09620390254759,2.82626898240154));
#12113=CARTESIAN_POINT('Ctrl Pts',(0.222224703879941,5.13682174297132,2.85168019626704));
#12114=CARTESIAN_POINT('Ctrl Pts',(-0.00184217065915739,5.14162629554737,
2.86370111824652));
#12115=CARTESIAN_POINT('Ctrl Pts',(-0.429811238103686,5.12281978570965,
2.88667120785942));
#12116=CARTESIAN_POINT('Ctrl Pts',(-0.633390554240987,5.10165008435015,
2.89760522478219));
#12117=CARTESIAN_POINT('Ctrl Pts',(-0.979080582536843,5.04468800522704,
2.91659481129789));
#12118=CARTESIAN_POINT('Ctrl Pts',(-1.12192229200466,5.01485439448364,2.92457496863274));
#12119=CARTESIAN_POINT('Ctrl Pts',(-1.55142586968957,4.9058781773376,2.94886351004635));
#12120=CARTESIAN_POINT('Ctrl Pts',(-1.83267253594294,4.80789790270234,2.96514088252546));
#12121=CARTESIAN_POINT('Ctrl Pts',(-2.30505156043652,4.59582108344528,2.99318787011608));
#12122=CARTESIAN_POINT('Ctrl Pts',(-2.50021299084452,4.4926352663032,3.00501788652547));
#12123=CARTESIAN_POINT('Ctrl Pts',(-2.84825957756841,4.2788930127771,3.02691594043159));
#12124=CARTESIAN_POINT('Ctrl Pts',(-3.00286004790986,4.17185056170326,3.03697212151953));
#12125=CARTESIAN_POINT('Ctrl Pts',(-3.25725051026099,3.97423425812866,3.05442532884527));
#12126=CARTESIAN_POINT('Ctrl Pts',(-3.35998524110482,3.88776497340196,3.06176239048907));
#12127=CARTESIAN_POINT('Ctrl Pts',(-3.69383167968171,3.58364795508103,3.0865061775217));
#12128=CARTESIAN_POINT('Ctrl Pts',(-3.90814534258248,3.34863176145679,3.10389463153942));
#12129=CARTESIAN_POINT('Ctrl Pts',(-4.16649034429435,3.00648554434302,3.12710801500211));
#12130=CARTESIAN_POINT('Ctrl Pts',(-4.23066960584482,2.91548064671473,3.13311049086494));
#12131=CARTESIAN_POINT('Ctrl Pts',(-4.29183621895492,2.82247097986264,3.13909688836532));
#12132=CARTESIAN_POINT('',(-5.13674999831709,-0.000131489181014188,1.07404150530312));
#12133=CARTESIAN_POINT('Ctrl Pts',(-4.29199677360937,2.82257643420045,2.66202500160396));
#12134=CARTESIAN_POINT('Ctrl Pts',(-4.21753523086708,2.93604918894789,2.65466501958149));
#12135=CARTESIAN_POINT('Ctrl Pts',(-3.64162075244998,3.74186919945967,2.60099021202329));
#12136=CARTESIAN_POINT('Ctrl Pts',(-2.13912211940093,4.90889399862105,2.50100057892936));
#12137=CARTESIAN_POINT('Ctrl Pts',(0.470139480393059,5.33404654130231,2.36205610232219));
#12138=CARTESIAN_POINT('Ctrl Pts',(2.96480561398902,4.45903705461135,2.22311162571499));
#12139=CARTESIAN_POINT('Ctrl Pts',(4.73680694601427,2.49714709212602,2.0841671491078));
#12140=CARTESIAN_POINT('Ctrl Pts',(5.35422202774455,-0.0734168574314198,
1.94522267250061));
#12141=CARTESIAN_POINT('Ctrl Pts',(4.66655737753191,-2.6260858009926,1.80627819589344));
#12142=CARTESIAN_POINT('Ctrl Pts',(2.84142957722535,-4.53865176071962,1.66733371928624));
#12143=CARTESIAN_POINT('Ctrl Pts',(0.323709801564174,-5.34493211998566,
1.52838924267905));
#12144=CARTESIAN_POINT('Ctrl Pts',(-2.27291392243804,-4.84839564767857,
1.38944476607187));
#12145=CARTESIAN_POINT('Ctrl Pts',(-4.31551911731205,-3.17007628077776,
1.25050028946468));
#12146=CARTESIAN_POINT('Ctrl Pts',(-5.06515352982256,-1.31547226615614,
1.14536587063201));
#12147=CARTESIAN_POINT('Ctrl Pts',(-5.13687131111266,-0.230764757637239,
1.08654627733508));
#12148=CARTESIAN_POINT('Ctrl Pts',(-5.13664618448387,-0.00013156529178269,
1.07404150957387));
#12149=CARTESIAN_POINT('Ctrl Pts',(-5.13674999831709,-0.000131489181014244,
1.07404150530312));
#12150=CARTESIAN_POINT('Ctrl Pts',(-5.13675398895607,0.15576662052808,1.06558899121539));
#12151=CARTESIAN_POINT('Ctrl Pts',(-5.12965553311713,0.311682248976567,
1.05713647712765));
#12152=CARTESIAN_POINT('Ctrl Pts',(-5.11548157266034,0.466957002594934,
1.04868396303992));
#12153=CARTESIAN_POINT('Ctrl Pts',(-5.10198818049961,0.614776177738121,
1.0406372997465));
#12154=CARTESIAN_POINT('Ctrl Pts',(-5.08208291523897,0.762014223800285,
1.03259063645309));
#12155=CARTESIAN_POINT('Ctrl Pts',(-5.0558422630955,0.908107688106076,1.02454397315967));
#12156=CARTESIAN_POINT('Ctrl Pts',(-5.029601885012,1.05419962659724,1.01649739390641));
#12157=CARTESIAN_POINT('Ctrl Pts',(-4.99702631447217,1.19914667878811,1.00845081465314));
#12158=CARTESIAN_POINT('Ctrl Pts',(-4.95824328173864,1.34239492013103,1.00040423539987));
#12159=CARTESIAN_POINT('Ctrl Pts',(-4.91945171273043,1.48567469088904,0.992355885067712));
#12160=CARTESIAN_POINT('Ctrl Pts',(-4.87445004172093,1.62725458178626,0.98430753473555));
#12161=CARTESIAN_POINT('Ctrl Pts',(-4.82341619095162,1.76659469357456,0.976259184403386));
#12162=CARTESIAN_POINT('Ctrl Pts',(-4.81570596750665,1.7876462775828,0.975043235019029));
#12163=CARTESIAN_POINT('Ctrl Pts',(-4.80785814898297,1.80864676985546,0.973827285634671));
#12164=CARTESIAN_POINT('Ctrl Pts',(-4.79987344606763,1.82959434417437,0.972611336250314));
#12165=CARTESIAN_POINT('Ctrl Pts',(-4.7468948658969,1.96858170002269,0.96454350046158));
#12166=CARTESIAN_POINT('Ctrl Pts',(-4.68786554548279,2.10529213254811,0.956475664672847));
#12167=CARTESIAN_POINT('Ctrl Pts',(-4.62300639714695,2.2391990564571,0.948407828884113));
#12168=CARTESIAN_POINT('Ctrl Pts',(-4.5581579010614,2.37308398793935,0.940341318129831));
#12169=CARTESIAN_POINT('Ctrl Pts',(-4.48748163017484,2.50416603095612,0.932274807375549));
#12170=CARTESIAN_POINT('Ctrl Pts',(-4.41124562792507,2.63194083759721,0.924208296621267));
#12171=CARTESIAN_POINT('Ctrl Pts',(-4.37283988231778,2.69631051300072,0.92014459507836));
#12172=CARTESIAN_POINT('Ctrl Pts',(-4.33302387301076,2.75984122459489,0.916080893535454));
#12173=CARTESIAN_POINT('Ctrl Pts',(-4.29183622825303,2.82247096572397,0.912017191992546));
#12174=CARTESIAN_POINT('Origin',(0.,0.,-3.86474103256053));
#12175=CARTESIAN_POINT('',(-6.11324999844244,0.000137998184040776,2.26025896739919));
#12176=CARTESIAN_POINT('Ctrl Pts',(3.72292453512039,-4.84888218750453,1.13013653271955));
#12177=CARTESIAN_POINT('Ctrl Pts',(3.8573754093748,-4.74565211525817,1.13785962463316));
#12178=CARTESIAN_POINT('Ctrl Pts',(3.98754469999778,-4.63681523196678,1.14558271654677));
#12179=CARTESIAN_POINT('Ctrl Pts',(4.1129725893008,-4.52275160075813,1.15330580846038));
#12180=CARTESIAN_POINT('Ctrl Pts',(4.23840615502252,-4.40868280743656,1.16102924989358));
#12181=CARTESIAN_POINT('Ctrl Pts',(4.35909765329052,-4.28938700356551,1.16875269132677));
#12182=CARTESIAN_POINT('Ctrl Pts',(4.47462201540418,-4.16528310943689,1.17647613275996));
#12183=CARTESIAN_POINT('Ctrl Pts',(4.59014003349401,-4.04118603047735,1.18419915006014));
#12184=CARTESIAN_POINT('Ctrl Pts',(4.70049126774584,-3.91228162202903,1.19192216736031));
#12185=CARTESIAN_POINT('Ctrl Pts',(4.80528891848427,-3.77902420902437,1.19964518466048));
#12186=CARTESIAN_POINT('Ctrl Pts',(4.91011305231619,-3.64573312094682,1.20737015362072));
#12187=CARTESIAN_POINT('Ctrl Pts',(5.00938060121277,-3.50808707864231,1.21509512258095));
#12188=CARTESIAN_POINT('Ctrl Pts',(5.10274576734098,-3.36657261861135,1.22282009154118));
#12189=CARTESIAN_POINT('Ctrl Pts',(5.18201307759727,-3.24642641126009,1.22937861370404));
#12190=CARTESIAN_POINT('Ctrl Pts',(5.25702655387851,-3.12349244938812,1.2359371358669));
#12191=CARTESIAN_POINT('Ctrl Pts',(5.32759941172684,-2.99808440019087,1.24249565802976));
#12192=CARTESIAN_POINT('Ctrl Pts',(5.41072151689508,-2.85037632413816,1.25022041490642));
#12193=CARTESIAN_POINT('Ctrl Pts',(5.48771173147153,-2.69918311039753,1.25794517178308));
#12194=CARTESIAN_POINT('Ctrl Pts',(5.55829382787376,-2.54503345469572,1.26566992865974));
#12195=CARTESIAN_POINT('Ctrl Pts',(5.62886215520052,-2.39091387033428,1.27339317859957));
#12196=CARTESIAN_POINT('Ctrl Pts',(5.69302472686585,-2.23383928279505,1.2811164285394));
#12197=CARTESIAN_POINT('Ctrl Pts',(5.7505524945068,-2.07436052084049,1.28883967847924));
#12198=CARTESIAN_POINT('Ctrl Pts',(5.80808248480531,-1.91487559722365,1.29656322681653));
#12199=CARTESIAN_POINT('Ctrl Pts',(5.85897704685537,-1.75298661008816,1.30428677515382));
#12200=CARTESIAN_POINT('Ctrl Pts',(5.90305600247511,-1.58926253153549,1.31201032349112));
#12201=CARTESIAN_POINT('Ctrl Pts',(5.94713199739441,-1.42554945002085,1.31973335305221));
#12202=CARTESIAN_POINT('Ctrl Pts',(5.98439321960548,-1.26000182981357,1.32745638261331));
#12203=CARTESIAN_POINT('Ctrl Pts',(6.01470986616232,-1.09320208030794,1.33517941217441));
#12204=CARTESIAN_POINT('Ctrl Pts',(6.0450345695927,-0.926358002532552,1.34290449418785));
#12205=CARTESIAN_POINT('Ctrl Pts',(6.0684109506079,-0.758261442167187,1.3506295762013));
#12206=CARTESIAN_POINT('Ctrl Pts',(6.08476050236919,-0.589504191085879,
1.35835465821474));
#12207=CARTESIAN_POINT('Ctrl Pts',(6.10104672392827,-0.421400623420052,
1.36604981702215));
#12208=CARTESIAN_POINT('Ctrl Pts',(6.11036045856332,-0.252641788184692,
1.37374497582955));
#12209=CARTESIAN_POINT('Ctrl Pts',(6.1126753807856,-0.0838167742016235,
1.38144013463695));
#12210=CARTESIAN_POINT('Ctrl Pts',(6.11499920959529,0.085657788491336,1.38916490031574));
#12211=CARTESIAN_POINT('Ctrl Pts',(6.11027105680977,0.25525906309682,1.39688966599452));
#12212=CARTESIAN_POINT('Ctrl Pts',(6.09850130396609,0.424390631404504,1.40461443167331));
#12213=CARTESIAN_POINT('Ctrl Pts',(6.08673384695857,0.593489208503662,1.41233769054082));
#12214=CARTESIAN_POINT('Ctrl Pts',(6.06792755260796,0.762117946154579,1.42006094940833));
#12215=CARTESIAN_POINT('Ctrl Pts',(6.04214482084422,0.929683562533715,1.42778420827583));
#12216=CARTESIAN_POINT('Ctrl Pts',(6.01636109256515,1.09725565540678,1.43550776565111));
#12217=CARTESIAN_POINT('Ctrl Pts',(5.98360043158213,1.26376423095059,1.44323132302639));
#12218=CARTESIAN_POINT('Ctrl Pts',(5.94397683230493,1.42862345617108,1.45095488040167));
#12219=CARTESIAN_POINT('Ctrl Pts',(5.90435589424919,1.59347160902775,1.45867791904324));
#12220=CARTESIAN_POINT('Ctrl Pts',(5.85787301437743,1.75667032506029,1.46640095768481));
#12221=CARTESIAN_POINT('Ctrl Pts',(5.80469285169398,1.91764607266118,1.47412399632638));
#12222=CARTESIAN_POINT('Ctrl Pts',(5.75149855611477,2.07866460037678,1.48184908740432));
#12223=CARTESIAN_POINT('Ctrl Pts',(5.69160351859424,2.23745867734327,1.48957417848227));
#12224=CARTESIAN_POINT('Ctrl Pts',(5.62522193143055,2.39347107453856,1.49729926956021));
#12225=CARTESIAN_POINT('Ctrl Pts',(5.55909793773548,2.54887806628547,1.50499438345485));
#12226=CARTESIAN_POINT('Ctrl Pts',(5.48653779880018,2.70152465381282,1.51268949734949));
#12227=CARTESIAN_POINT('Ctrl Pts',(5.40780022989844,2.85088095788134,1.52038461124413));
#12228=CARTESIAN_POINT('Ctrl Pts',(5.32875931489969,3.00081267534571,1.52810937150453));
#12229=CARTESIAN_POINT('Ctrl Pts',(5.24346525628034,3.14748179386505,1.53583413176492));
#12230=CARTESIAN_POINT('Ctrl Pts',(5.1522125135047,3.29036955039788,1.54355889202531));
#12231=CARTESIAN_POINT('Ctrl Pts',(5.06097757157155,3.43322943354991,1.55128214540233));
#12232=CARTESIAN_POINT('Ctrl Pts',(4.96378643530744,3.57230915962419,1.55900539877935));
#12233=CARTESIAN_POINT('Ctrl Pts',(4.8609777423659,3.70711760681036,1.56672865215637));
#12234=CARTESIAN_POINT('Ctrl Pts',(4.75816507661087,3.84193126336939,1.57445220398136));
#12235=CARTESIAN_POINT('Ctrl Pts',(4.64973460882364,3.97247305635589,1.58217575580634));
#12236=CARTESIAN_POINT('Ctrl Pts',(4.53606671939524,4.09828308925761,1.58989930763133));
#12237=CARTESIAN_POINT('Ctrl Pts',(4.4224064645163,4.22408467207792,1.59762234070085));
#12238=CARTESIAN_POINT('Ctrl Pts',(4.30350970444383,4.34515489562437,1.60534537377038));
#12239=CARTESIAN_POINT('Ctrl Pts',(4.17979542414352,4.46106890496089,1.6130684068399));
#12240=CARTESIAN_POINT('Ctrl Pts',(4.05604826585309,4.57701371930749,1.62079349236291));
#12241=CARTESIAN_POINT('Ctrl Pts',(3.92748125894714,4.68779936281262,1.62851857788591));
#12242=CARTESIAN_POINT('Ctrl Pts',(3.79454908524854,4.79303899443135,1.63624366340891));
#12243=CARTESIAN_POINT('Ctrl Pts',(3.66213218437205,4.89787069529506,1.64393880488972));
#12244=CARTESIAN_POINT('Ctrl Pts',(3.52538416193958,4.99719913435962,1.65163394637052));
#12245=CARTESIAN_POINT('Ctrl Pts',(3.38478571790181,5.09068278390904,1.65932908785133));
#12246=CARTESIAN_POINT('Ctrl Pts',(3.24364606032508,5.18452628535551,1.66705385067526));
#12247=CARTESIAN_POINT('Ctrl Pts',(3.09857627483836,5.27251312228381,1.67477861349919));
#12248=CARTESIAN_POINT('Ctrl Pts',(2.95008312582068,5.35432863328803,1.68250337632312));
#12249=CARTESIAN_POINT('Ctrl Pts',(2.80161894301487,5.43612818473155,1.6902266322956));
#12250=CARTESIAN_POINT('Ctrl Pts',(2.64973300656674,5.51175865946843,1.69794988826809));
#12251=CARTESIAN_POINT('Ctrl Pts',(2.4949576504884,5.58095080472579,1.70567314424057));
#12252=CARTESIAN_POINT('Ctrl Pts',(2.34017631296394,5.65014562398176,1.71339669868589));
#12253=CARTESIAN_POINT('Ctrl Pts',(2.182505620068,5.71290148290529,1.72112025313121));
#12254=CARTESIAN_POINT('Ctrl Pts',(2.02249962209345,5.76899651942449,1.72884380757653));
#12255=CARTESIAN_POINT('Ctrl Pts',(1.86250437080764,5.82508778836056,1.73656684327482));
#12256=CARTESIAN_POINT('Ctrl Pts',(1.70017442743467,5.87451902529616,1.74428987897312));
#12257=CARTESIAN_POINT('Ctrl Pts',(1.5360809770284,5.91711760864287,1.75201291467141));
#12258=CARTESIAN_POINT('Ctrl Pts',(1.37194391781922,5.95972751281451,1.75973800281202));
#12259=CARTESIAN_POINT('Ctrl Pts',(1.20604272150252,5.99550105315179,1.76746309095263));
#12260=CARTESIAN_POINT('Ctrl Pts',(1.03896173250995,6.02431606747852,1.77518817909324));
#12261=CARTESIAN_POINT('Ctrl Pts',(0.872528722387847,6.05301933048904,1.78288330754833));
#12262=CARTESIAN_POINT('Ctrl Pts',(0.704925367465891,6.07481792380217,1.79057843600341));
#12263=CARTESIAN_POINT('Ctrl Pts',(0.536737176574621,6.08964192426638,1.7982735644585));
#12264=CARTESIAN_POINT('Ctrl Pts',(0.367901302971622,6.10452301107397,1.80599832639521));
#12265=CARTESIAN_POINT('Ctrl Pts',(0.198416280939758,6.11238092141685,1.81372308833193));
#12266=CARTESIAN_POINT('Ctrl Pts',(0.0288776565905395,6.11318179375109,
1.82144785026864));
#12267=CARTESIAN_POINT('Ctrl Pts',(-0.140627896034936,6.11398250986,1.82917110534405));
#12268=CARTESIAN_POINT('Ctrl Pts',(-0.310186713383548,6.10772893329223,
1.83689436041945));
#12269=CARTESIAN_POINT('Ctrl Pts',(-0.479202520794083,6.09443931027003,
1.84461761549486));
#12270=CARTESIAN_POINT('Ctrl Pts',(-0.648224859840653,6.08114917366876,
1.85234116903638));
#12271=CARTESIAN_POINT('Ctrl Pts',(-0.816703830704214,6.06082246740018,
1.86006472257791));
#12272=CARTESIAN_POINT('Ctrl Pts',(-0.984046762183985,6.03352944240228,
1.86778827611943));
#12273=CARTESIAN_POINT('Ctrl Pts',(-1.15137845415264,6.00623825052787,1.87551131091203));
#12274=CARTESIAN_POINT('Ctrl Pts',(-1.31757394660641,5.97198172727477,1.88323434570462));
#12275=CARTESIAN_POINT('Ctrl Pts',(-1.48204907994823,5.93088156070618,1.89095738049722));
#12276=CARTESIAN_POINT('Ctrl Pts',(-1.64656792365069,5.88977047149496,1.89868246773768));
#12277=CARTESIAN_POINT('Ctrl Pts',(-1.8093651864335,5.84181217944948,1.90640755497814));
#12278=CARTESIAN_POINT('Ctrl Pts',(-1.96986929436292,5.78717897819189,1.9141326422186));
#12279=CARTESIAN_POINT('Ctrl Pts',(-2.12975104209433,5.73275761905093,1.92182777516763));
#12280=CARTESIAN_POINT('Ctrl Pts',(-2.28735710178446,5.67171315417662,1.92952290811666));
#12281=CARTESIAN_POINT('Ctrl Pts',(-2.44213986854364,5.60426430720123,1.93721804106569));
#12282=CARTESIAN_POINT('Ctrl Pts',(-2.59751860636432,5.53655575714796,1.94494280313073));
#12283=CARTESIAN_POINT('Ctrl Pts',(-2.75010728523121,5.46236940070029,1.95266756519576));
#12284=CARTESIAN_POINT('Ctrl Pts',(-2.8993667401887,5.38196042984223,1.9603923272608));
#12285=CARTESIAN_POINT('Ctrl Pts',(-3.04859707926959,5.30156714427307,1.96811558246505));
#12286=CARTESIAN_POINT('Ctrl Pts',(-3.19449921143748,5.21495381655532,1.97583883766931));
#12287=CARTESIAN_POINT('Ctrl Pts',(-3.33655826185793,5.12242174442202,1.98356209287356));
#12288=CARTESIAN_POINT('Ctrl Pts',(-3.47862280215923,5.02988609638103,1.9912856465435));
#12289=CARTESIAN_POINT('Ctrl Pts',(-3.61684369580897,4.93143141587311,1.99900920021343));
#12290=CARTESIAN_POINT('Ctrl Pts',(-3.75073411284258,4.82740294332874,2.00673275388336));
#12291=CARTESIAN_POINT('Ctrl Pts',(-3.8846155371794,4.72338145781549,2.01445578880387));
#12292=CARTESIAN_POINT('Ctrl Pts',(-4.01416681666281,4.61378712389629,2.02217882372439));
#12293=CARTESIAN_POINT('Ctrl Pts',(-4.13893320461471,4.49900627808384,2.0299018586449));
#12294=CARTESIAN_POINT('Ctrl Pts',(-4.26373275003021,4.38419492852932,2.03762694601121));
#12295=CARTESIAN_POINT('Ctrl Pts',(-4.38374462803762,4.26419452592647,2.04535203337753));
#12296=CARTESIAN_POINT('Ctrl Pts',(-4.49854935493777,4.13942982350094,2.05307712074384));
#12297=CARTESIAN_POINT('Ctrl Pts',(-4.61290891119671,4.01514891285017,2.06077225305352));
#12298=CARTESIAN_POINT('Ctrl Pts',(-4.72210143974045,3.88614083667116,2.0684673853632));
#12299=CARTESIAN_POINT('Ctrl Pts',(-4.82575071829774,3.75285965196526,2.07616251767288));
#12300=CARTESIAN_POINT('Ctrl Pts',(-4.9297990952227,3.61906527214603,2.08388727985347));
#12301=CARTESIAN_POINT('Ctrl Pts',(-5.02829827631538,3.48091740713,2.09161204203406));
#12302=CARTESIAN_POINT('Ctrl Pts',(-5.1208968980597,3.3388980999639,2.09933680421466));
#12303=CARTESIAN_POINT('Ctrl Pts',(-5.21347745671865,3.19690649630808,2.10706005953655));
#12304=CARTESIAN_POINT('Ctrl Pts',(-5.30015957972249,3.05104522270951,2.11478331485844));
#12305=CARTESIAN_POINT('Ctrl Pts',(-5.38063529168392,2.90182518777156,2.12250657018033));
#12306=CARTESIAN_POINT('Ctrl Pts',(-5.46111411365661,2.75259938617462,2.13023012397006));
#12307=CARTESIAN_POINT('Ctrl Pts',(-5.53538589071419,2.60001484055764,2.13795367775978));
#12308=CARTESIAN_POINT('Ctrl Pts',(-5.60318829787371,2.44460762926715,2.1456772315495));
#12309=CARTESIAN_POINT('Ctrl Pts',(-5.67098615111975,2.28921085582132,2.15340026659074));
#12310=CARTESIAN_POINT('Ctrl Pts',(-5.73231537725609,2.13099208660288,2.16112330163198));
#12311=CARTESIAN_POINT('Ctrl Pts',(-5.78696148603909,1.9705081379178,2.16884633667322));
#12312=CARTESIAN_POINT('Ctrl Pts',(-5.84162211737673,1.80998153959186,2.17657142416066));
#12313=CARTESIAN_POINT('Ctrl Pts',(-5.88959597802767,1.64718885840498,2.1842965116481));
#12314=CARTESIAN_POINT('Ctrl Pts',(-5.93071792276978,1.48270377454071,2.19202159913554));
#12315=CARTESIAN_POINT('Ctrl Pts',(-5.97168040787764,1.3188565187626,2.19971673085038));
#12316=CARTESIAN_POINT('Ctrl Pts',(-6.00584397787393,1.15333027300864,2.20741186256523));
#12317=CARTESIAN_POINT('Ctrl Pts',(-6.03309549633831,0.986703752178132,
2.21510699428008));
#12318=CARTESIAN_POINT('Ctrl Pts',(-6.06145111302405,0.81332633981401,2.22311389508957));
#12319=CARTESIAN_POINT('Ctrl Pts',(-6.08233074226667,0.63871365318621,2.23112079589906));
#12320=CARTESIAN_POINT('Ctrl Pts',(-6.09565353383094,0.463501410995017,
2.23912769670856));
#12321=CARTESIAN_POINT('Ctrl Pts',(-6.10737373709051,0.309365314056196,
2.24617145360543));
#12322=CARTESIAN_POINT('Ctrl Pts',(-6.1132465079406,0.154765470390503,2.25321521050231));
#12323=CARTESIAN_POINT('Ctrl Pts',(-6.11324999844244,0.000137998184036704,
2.26025896739919));
#12324=CARTESIAN_POINT('Ctrl Pts',(-6.11324999844246,0.000137997300213472,
2.26025896743945));
#12325=CARTESIAN_POINT('Ctrl Pts',(-6.11325387162186,-0.171442996720229,
2.26807500939343));
#12326=CARTESIAN_POINT('Ctrl Pts',(-6.1060295174546,-0.343034351920675,
2.27589105134742));
#12327=CARTESIAN_POINT('Ctrl Pts',(-6.09160170655671,-0.514017714845873,
2.2837070933014));
#12328=CARTESIAN_POINT('Ctrl Pts',(-6.07735174577439,-0.682893383743797,
2.2914267877239));
#12329=CARTESIAN_POINT('Ctrl Pts',(-6.05607496211486,-0.851175644165355,
2.2991464821464));
#12330=CARTESIAN_POINT('Ctrl Pts',(-6.02784749187544,-1.01827313486656,
2.30686617656889));
#12331=CARTESIAN_POINT('Ctrl Pts',(-5.99909157188228,-1.18849887712782,
2.31473039228862));
#12332=CARTESIAN_POINT('Ctrl Pts',(-5.96312217325259,-1.35749471095138,
2.32259460800834));
#12333=CARTESIAN_POINT('Ctrl Pts',(-5.92007454414292,-1.52464518963953,
2.33045882372807));
#12334=CARTESIAN_POINT('Ctrl Pts',(-5.87702691503326,-1.69179566832769,
2.3383230394478));
#12335=CARTESIAN_POINT('Ctrl Pts',(-5.82690115090709,-1.85710045725307,
2.34618725516752));
#12336=CARTESIAN_POINT('Ctrl Pts',(-5.76988658228266,-2.01995900703318,
2.35405147088725));
#12337=CARTESIAN_POINT('Ctrl Pts',(-5.71388303448856,-2.17992963903727,
2.36177623302347));
#12338=CARTESIAN_POINT('Ctrl Pts',(-5.65121266928852,-2.33759810852869,
2.36950099515969));
#12339=CARTESIAN_POINT('Ctrl Pts',(-5.58209000656017,-2.49240781598058,
2.37722575729591));
#12340=CARTESIAN_POINT('Ctrl Pts',(-5.51298082750083,-2.64718732490174,
2.3849490125727));
#12341=CARTESIAN_POINT('Ctrl Pts',(-5.4374219914878,-2.7991088952909,2.3926722678495));
#12342=CARTESIAN_POINT('Ctrl Pts',(-5.35567579798097,-2.94763673294741,
2.40039552312629));
#12343=CARTESIAN_POINT('Ctrl Pts',(-5.27392644537287,-3.09617031049787,
2.40811907687014));
#12344=CARTESIAN_POINT('Ctrl Pts',(-5.18598940613194,-3.2413096133189,2.41584263061399));
#12345=CARTESIAN_POINT('Ctrl Pts',(-5.09217288055155,-3.38254355730644,
2.42356618435784));
#12346=CARTESIAN_POINT('Ctrl Pts',(-4.99836265611334,-3.52376801538351,
2.43128921935289));
#12347=CARTESIAN_POINT('Ctrl Pts',(-4.89867391096325,-3.66108737552215,
2.43901225434793));
#12348=CARTESIAN_POINT('Ctrl Pts',(-4.79345820682571,-3.7940195020473,2.44673528934298));
#12349=CARTESIAN_POINT('Ctrl Pts',(-4.68821454093948,-3.92698695613828,
2.45446037678414));
#12350=CARTESIAN_POINT('Ctrl Pts',(-4.57744117611848,-4.05556459676049,
2.46218546422531));
#12351=CARTESIAN_POINT('Ctrl Pts',(-4.46153059924172,-4.17930260624064,
2.46991055166648));
#12352=CARTESIAN_POINT('Ctrl Pts',(-4.3460694877127,-4.30256079801168,2.47760568360913));
#12353=CARTESIAN_POINT('Ctrl Pts',(-4.22551117129597,-4.42101661930306,
2.48530081555179));
#12354=CARTESIAN_POINT('Ctrl Pts',(-4.10028056703834,-4.53426122252212,
2.49299594749444));
#12355=CARTESIAN_POINT('Ctrl Pts',(-3.97456776167407,-4.64794187468716,
2.5007207095835));
#12356=CARTESIAN_POINT('Ctrl Pts',(-3.84410207183109,-4.75641133750185,
2.50844547167256));
#12357=CARTESIAN_POINT('Ctrl Pts',(-3.70933816649836,-4.85928347897697,
2.51617023376162));
#12358=CARTESIAN_POINT('Ctrl Pts',(-3.57460054939822,-4.96213555330745,
2.52389348899064));
#12359=CARTESIAN_POINT('Ctrl Pts',(-3.43556664157642,-5.05939229277082,
2.53161674421967));
#12360=CARTESIAN_POINT('Ctrl Pts',(-3.29272311464412,-5.15070869422726,
2.5393399994487));
#12361=CARTESIAN_POINT('Ctrl Pts',(-3.14987406749818,-5.24202862462238,
2.54706355314431));
#12362=CARTESIAN_POINT('Ctrl Pts',(-3.00321537152376,-5.32740758360003,
2.55478710683992));
#12363=CARTESIAN_POINT('Ctrl Pts',(-2.85326218301945,-5.40654422690235,
2.56251066053553));
#12364=CARTESIAN_POINT('Ctrl Pts',(-2.70331906605275,-5.48567555502805,
2.57023369548217));
#12365=CARTESIAN_POINT('Ctrl Pts',(-2.55008217967926,-5.55856525856189,
2.57795673042881));
#12366=CARTESIAN_POINT('Ctrl Pts',(-2.39409090722725,-5.62495815899388,
2.58567976537545));
#12367=CARTESIAN_POINT('Ctrl Pts',(-2.2380581790894,-5.69136870376698,2.5934048527684));
#12368=CARTESIAN_POINT('Ctrl Pts',(-2.07926989313185,-5.75127886912873,
2.60112994016134));
#12369=CARTESIAN_POINT('Ctrl Pts',(-1.91828590825238,-5.80448143564094,
2.60885502755429));
#12370=CARTESIAN_POINT('Ctrl Pts',(-1.75792616345052,-5.85747770104641,
2.61655015973674));
#12371=CARTESIAN_POINT('Ctrl Pts',(-1.59538802431163,-5.90381822726308,
2.62424529191918));
#12372=CARTESIAN_POINT('Ctrl Pts',(-1.43124022628975,-5.94334728727424,
2.63194042410163));
#12373=CARTESIAN_POINT('Ctrl Pts',(-1.26646038104637,-5.98302855299787,
2.6396651862089));
#12374=CARTESIAN_POINT('Ctrl Pts',(-1.10000008925648,-6.01585981834215,
2.64738994831617));
#12375=CARTESIAN_POINT('Ctrl Pts',(-0.932443344467888,-6.04171953766952,
2.65511471042344));
#12376=CARTESIAN_POINT('Ctrl Pts',(-0.764919284766879,-6.06757421257333,
2.66283796567089));
#12377=CARTESIAN_POINT('Ctrl Pts',(-0.596299511869711,-6.08646000669851,
2.67056122091834));
#12378=CARTESIAN_POINT('Ctrl Pts',(-0.42717644441767,-6.09830680171428,
2.67828447616579));
#12379=CARTESIAN_POINT('Ctrl Pts',(-0.258046841170889,-6.11015405455181,
2.68600802987998));
#12380=CARTESIAN_POINT('Ctrl Pts',(-0.0884142203152118,-6.11496173784735,
2.69373158359417));
#12381=CARTESIAN_POINT('Ctrl Pts',(0.081124874046489,-6.11271169918155,
2.70145513730837));
#12382=CARTESIAN_POINT('Ctrl Pts',(0.250652581392769,-6.11046181163856,
2.70917817227362));
#12383=CARTESIAN_POINT('Ctrl Pts',(0.420086457886345,-6.10115515495588,
2.71690120723887));
#12384=CARTESIAN_POINT('Ctrl Pts',(0.588830772081147,-6.08482570698211,
2.72462424220413));
#12385=CARTESIAN_POINT('Ctrl Pts',(0.757619931163056,-6.06849191935248,
2.73234932961561));
#12386=CARTESIAN_POINT('Ctrl Pts',(0.925718845871653,-6.04513163938592,
2.74007441702709));
#12387=CARTESIAN_POINT('Ctrl Pts',(1.09253674965138,-6.01483075515523,2.74779950443857));
#12388=CARTESIAN_POINT('Ctrl Pts',(1.2587077890454,-5.9846473676825,2.75549463652866));
#12389=CARTESIAN_POINT('Ctrl Pts',(1.42360743311793,-5.94757719448578,2.76318976861874));
#12390=CARTESIAN_POINT('Ctrl Pts',(1.58666175608273,-5.90375558727531,2.77088490070882));
#12391=CARTESIAN_POINT('Ctrl Pts',(1.75034234718392,-5.85976566759215,2.77860958869135));
#12392=CARTESIAN_POINT('Ctrl Pts',(1.91222137634933,-5.80895673992962,2.78633427667389));
#12393=CARTESIAN_POINT('Ctrl Pts',(2.07172788897545,-5.75150146627307,2.79405896465642));
#12394=CARTESIAN_POINT('Ctrl Pts',(2.23121533170672,-5.69405306171553,2.80178272910935));
#12395=CARTESIAN_POINT('Ctrl Pts',(2.38833052483343,-5.62996000125963,2.80950649356227));
#12396=CARTESIAN_POINT('Ctrl Pts',(2.54251959434355,-5.55944418758558,2.81723025801519));
#12397=CARTESIAN_POINT('Ctrl Pts',(2.69668717969285,-5.48893819933616,2.82495294626603));
#12398=CARTESIAN_POINT('Ctrl Pts',(2.84792916754531,-5.41201137691455,2.83267563451688));
#12399=CARTESIAN_POINT('Ctrl Pts',(2.99571321128252,-5.32893309380474,2.84039832276772));
#12400=CARTESIAN_POINT('Ctrl Pts',(3.14351076533101,-5.24584721573789,2.84812171702118));
#12401=CARTESIAN_POINT('Ctrl Pts',(3.28784946631342,-5.1566089068414,2.85584511127464));
#12402=CARTESIAN_POINT('Ctrl Pts',(3.42822237126001,-5.06153306179979,2.8635685055281));
#12403=CARTESIAN_POINT('Ctrl Pts',(3.52853996042675,-4.99358704639039,2.86908803432881));
#12404=CARTESIAN_POINT('Ctrl Pts',(3.62683264091644,-4.92266060832901,2.87460756312952));
#12405=CARTESIAN_POINT('Ctrl Pts',(3.72292453512039,-4.84888218750453,2.88012709193022));
#12406=CARTESIAN_POINT('',(-6.11324999796762,0.0001576353973087,2.11474103256055));
#12407=CARTESIAN_POINT('Ctrl Pts',(-6.11324999796762,0.0001576353973087,
2.11474103256055));
#12408=CARTESIAN_POINT('Ctrl Pts',(-6.11325435310326,-0.168738649423157,
2.12243630998825));
#12409=CARTESIAN_POINT('Ctrl Pts',(-6.10625498998438,-0.337657948030418,
2.13013158741595));
#12410=CARTESIAN_POINT('Ctrl Pts',(-6.09227225641602,-0.506008217525845,
2.13782686484365));
#12411=CARTESIAN_POINT('Ctrl Pts',(-6.07828929035017,-0.674361286260356,
2.14552227022435));
#12412=CARTESIAN_POINT('Ctrl Pts',(-6.05732274391698,-0.84214498618751,
2.15321767560505));
#12413=CARTESIAN_POINT('Ctrl Pts',(-6.02944494908661,-1.00877111796181,
2.16091308098575));
#12414=CARTESIAN_POINT('Ctrl Pts',(-6.00156865647815,-1.17538827092607,
2.16860807169209));
#12415=CARTESIAN_POINT('Ctrl Pts',(-5.96678191434973,-1.3408476635067,2.17630306239844));
#12416=CARTESIAN_POINT('Ctrl Pts',(-5.92520844601766,-1.50456985007045,
2.18399805310479));
#12417=CARTESIAN_POINT('Ctrl Pts',(-5.88362467080505,-1.66833262658461,
2.19169495155069));
#12418=CARTESIAN_POINT('Ctrl Pts',(-5.83525088602938,-1.83035702456957,
2.19939184999659));
#12419=CARTESIAN_POINT('Ctrl Pts',(-5.78026131824623,-1.99007654508222,
2.20708874844249));
#12420=CARTESIAN_POINT('Ctrl Pts',(-5.74210347661473,-2.10090760658855,
2.21242970753332));
#12421=CARTESIAN_POINT('Ctrl Pts',(-5.7007611108435,-2.21062911917225,2.21777066662415));
#12422=CARTESIAN_POINT('Ctrl Pts',(-5.65630632717199,-2.31905676853632,
2.22311162571499));
#12423=CARTESIAN_POINT('Ctrl Pts',(-5.59201026082955,-2.47587839179245,
2.23083638853408));
#12424=CARTESIAN_POINT('Ctrl Pts',(-5.52117694864381,-2.6300522157125,2.23856115135317));
#12425=CARTESIAN_POINT('Ctrl Pts',(-5.44404973649907,-2.78103362601468,
2.24628591417226));
#12426=CARTESIAN_POINT('Ctrl Pts',(-5.36693756938016,-2.93198558472442,
2.25400917013984));
#12427=CARTESIAN_POINT('Ctrl Pts',(-5.28353409616438,-3.07974609033716,
2.26173242610742));
#12428=CARTESIAN_POINT('Ctrl Pts',(-5.19412928840774,-3.22379380510059,
2.269455682075));
#12429=CARTESIAN_POINT('Ctrl Pts',(-5.10472102551454,-3.36784708672936,
2.27717923651539));
#12430=CARTESIAN_POINT('Ctrl Pts',(-5.00931112773894,-3.5081870190292,2.28490279095577));
#12431=CARTESIAN_POINT('Ctrl Pts',(-4.90823411184662,-3.64431934190807,
2.29262634539616));
#12432=CARTESIAN_POINT('Ctrl Pts',(-4.80716388472028,-3.78044252155616,
2.3003493810895));
#12433=CARTESIAN_POINT('Ctrl Pts',(-4.70042749013053,-3.9123584028382,2.30807241678284));
#12434=CARTESIAN_POINT('Ctrl Pts',(-4.58840123239069,-4.03960390299539,
2.31579545247618));
#12435=CARTESIAN_POINT('Ctrl Pts',(-4.47634520301125,-4.16688321939573,
2.32352054061187));
#12436=CARTESIAN_POINT('Ctrl Pts',(-4.35899670926232,-4.28948943500712,
2.33124562874755));
#12437=CARTESIAN_POINT('Ctrl Pts',(-4.2367712337785,-4.40699388190261,2.33897071688324));
#12438=CARTESIAN_POINT('Ctrl Pts',(-4.11501977660236,-4.52404261971746,
2.34666584536288));
#12439=CARTESIAN_POINT('Ctrl Pts',(-3.98842934593239,-4.63602889699067,
2.35436097384253));
#12440=CARTESIAN_POINT('Ctrl Pts',(-3.85744566598918,-4.74256665703723,
2.36205610232218));
#12441=CARTESIAN_POINT('Ctrl Pts',(-3.72595757608652,-4.84951468733462,
2.36978086426033));
#12442=CARTESIAN_POINT('Ctrl Pts',(-3.58999574543703,-4.95101000774563,
2.37750562619848));
#12443=CARTESIAN_POINT('Ctrl Pts',(-3.45003442167379,-5.04669080207675,
2.38523038813663));
#12444=CARTESIAN_POINT('Ctrl Pts',(-3.31010040002098,-5.14235293205442,
2.39295364321347));
#12445=CARTESIAN_POINT('Ctrl Pts',(-3.16616870346133,-5.23220262040445,
2.40067689829031));
#12446=CARTESIAN_POINT('Ctrl Pts',(-3.01874338667934,-5.3159207977433,2.40840015336716));
#12447=CARTESIAN_POINT('Ctrl Pts',(-2.87131237262796,-5.39964221038134,
2.41612370691013));
#12448=CARTESIAN_POINT('Ctrl Pts',(-2.72038774181563,-5.47723147791105,
2.42384726045311));
#12449=CARTESIAN_POINT('Ctrl Pts',(-2.56649971049706,-5.54841462027835,
2.43157081399609));
#12450=CARTESIAN_POINT('Ctrl Pts',(-2.41262201499729,-5.61959298166265,
2.43929384879015));
#12451=CARTESIAN_POINT('Ctrl Pts',(-2.25578160496855,-5.68436594585324,
2.44701688358421));
#12452=CARTESIAN_POINT('Ctrl Pts',(-2.09653047525643,-5.74250690281005,
2.45473991837826));
#12453=CARTESIAN_POINT('Ctrl Pts',(-1.9372370234978,-5.80066331111272,2.46246500562017));
#12454=CARTESIAN_POINT('Ctrl Pts',(-1.77553186902071,-5.85218407946506,
2.47019009286207));
#12455=CARTESIAN_POINT('Ctrl Pts',(-1.61198494511743,-5.89689156244328,
2.47791518010397));
#12456=CARTESIAN_POINT('Ctrl Pts',(-1.44907218021927,-5.94142569056866,
2.48561031304577));
#12457=CARTESIAN_POINT('Ctrl Pts',(-1.28433221319907,-5.97919922568479,
2.49330544598756));
#12458=CARTESIAN_POINT('Ctrl Pts',(-1.11834114801678,-6.01008640862613,
2.50100057892936));
#12459=CARTESIAN_POINT('Ctrl Pts',(-0.951710955509462,-6.04109251870725,
2.50872534099443));
#12460=CARTESIAN_POINT('Ctrl Pts',(-0.783760990323875,-6.06517009324846,
2.51645010305951));
#12461=CARTESIAN_POINT('Ctrl Pts',(-0.615080805155099,-6.08222830594427,
2.52417486512458));
#12462=CARTESIAN_POINT('Ctrl Pts',(-0.446433524243184,-6.09928319111344,
2.53189812032887));
#12463=CARTESIAN_POINT('Ctrl Pts',(-0.27705662269999,-6.10932141473159,
2.53962137553317));
#12464=CARTESIAN_POINT('Ctrl Pts',(-0.107545376246114,-6.1123039481482,
2.54734463073746));
#12465=CARTESIAN_POINT('Ctrl Pts',(0.0619724209804701,-6.115286596825,2.55506818440743));
#12466=CARTESIAN_POINT('Ctrl Pts',(0.231624256707586,-6.11121300013985,
2.56279173807741));
#12467=CARTESIAN_POINT('Ctrl Pts',(0.400813454111122,-6.10009624001978,
2.57051529174738));
#12468=CARTESIAN_POINT('Ctrl Pts',(0.569991287989971,-6.08898022655246,
2.57823832666797));
#12469=CARTESIAN_POINT('Ctrl Pts',(0.738706229452274,-6.070822017091,2.58596136158855));
#12470=CARTESIAN_POINT('Ctrl Pts',(0.90636514052485,-6.04568670992315,2.59368439650914));
#12471=CARTESIAN_POINT('Ctrl Pts',(1.07406860802225,-6.02054472288712,2.6014094838755));
#12472=CARTESIAN_POINT('Ctrl Pts',(1.24071517036138,-5.98842197785238,2.60913457124187));
#12473=CARTESIAN_POINT('Ctrl Pts',(1.40571936345527,-5.94943515249195,2.61685965860824));
#12474=CARTESIAN_POINT('Ctrl Pts',(1.57008373077596,-5.91059950374839,2.62455479091768));
#12475=CARTESIAN_POINT('Ctrl Pts',(1.73281814681099,-5.86495301598595,2.63224992322712));
#12476=CARTESIAN_POINT('Ctrl Pts',(1.89335655291803,-5.81266088173242,2.63994505553656));
#12477=CARTESIAN_POINT('Ctrl Pts',(2.05793420996479,-5.75905304329604,2.64783380239074));
#12478=CARTESIAN_POINT('Ctrl Pts',(2.22026340992346,-5.69844132849409,2.65572254924493));
#12479=CARTESIAN_POINT('Ctrl Pts',(2.37974669582981,-5.6310417531916,2.66361129609911));
#12480=CARTESIAN_POINT('Ctrl Pts',(2.53588773868642,-5.56505465043022,2.67133472086832));
#12481=CARTESIAN_POINT('Ctrl Pts',(2.68930066551015,-5.49256150224778,2.67905814563753));
#12482=CARTESIAN_POINT('Ctrl Pts',(2.83944450143217,-5.4138138576965,2.68678157040674));
#12483=CARTESIAN_POINT('Ctrl Pts',(2.99440914407056,-5.33253778984085,2.69475297830341));
#12484=CARTESIAN_POINT('Ctrl Pts',(3.14589094439971,-5.2445990326299,2.70272438620009));
#12485=CARTESIAN_POINT('Ctrl Pts',(3.29332181854905,-5.15032590832549,2.71069579409676));
#12486=CARTESIAN_POINT('Ctrl Pts',(3.44075269269837,-5.05605278402109,2.71866720199343));
#12487=CARTESIAN_POINT('Ctrl Pts',(3.58413232802228,-4.95544549284129,2.7266386098901));
#12488=CARTESIAN_POINT('Ctrl Pts',(3.72292453512037,-4.84888218750454,2.73461001778677));
#12489=CARTESIAN_POINT('Ctrl Pts',(3.72318137141383,-4.84921626688776,0.984617815426764));
#12490=CARTESIAN_POINT('Ctrl Pts',(4.45925545347764,-4.2832330214638,1.02693048123701));
#12491=CARTESIAN_POINT('Ctrl Pts',(5.72853657905866,-2.74185888015094,1.11555797258299));
#12492=CARTESIAN_POINT('Ctrl Pts',(6.36790888585768,0.246115919908329,1.25050028946468));
#12493=CARTESIAN_POINT('Ctrl Pts',(5.47407798976948,3.26271229099702,1.38944476607187));
#12494=CARTESIAN_POINT('Ctrl Pts',(3.24595379495023,5.48403304914773,1.52838924267906));
#12495=CARTESIAN_POINT('Ctrl Pts',(0.22663497067087,6.36863119357982,1.66733371928624));
#12496=CARTESIAN_POINT('Ctrl Pts',(-2.84792533819912,5.70089041666575,1.80627819589343));
#12497=CARTESIAN_POINT('Ctrl Pts',(-5.22831028765922,3.64356976551659,1.94522267250062));
#12498=CARTESIAN_POINT('Ctrl Pts',(-6.04676335981403,1.4639066170294,2.04804361805632));
#12499=CARTESIAN_POINT('Ctrl Pts',(-6.11351535343457,0.223837879067313,
2.1045497380763));
#12500=CARTESIAN_POINT('Ctrl Pts',(-6.11328444993451,0.000157636285682099,
2.11474103256055));
#12501=CARTESIAN_POINT('Ctrl Pts',(3.87932907111019,-3.36622224230924,0.000294770375723887));
#12502=CARTESIAN_POINT('Ctrl Pts',(4.43916355178267,-2.72105483262093,0.0466153921027713));
#12503=CARTESIAN_POINT('Ctrl Pts',(5.23010367843801,-1.14675700997481,0.139250839365547));
#12504=CARTESIAN_POINT('Ctrl Pts',(5.1410027524235,1.49571158632152,0.278201112164053));
#12505=CARTESIAN_POINT('Ctrl Pts',(3.79898575529339,3.77284335683313,0.417145588771241));
#12506=CARTESIAN_POINT('Ctrl Pts',(1.53088506617911,5.13067232132384,0.556090065378428));
#12507=CARTESIAN_POINT('Ctrl Pts',(-1.11032056394027,5.23774955056566,0.695034541985614));
#12508=CARTESIAN_POINT('Ctrl Pts',(-3.48091084250257,4.06821920710838,0.833979018592801));
#12509=CARTESIAN_POINT('Ctrl Pts',(-5.0030251669043,1.90702749096064,0.972923495199987));
#12510=CARTESIAN_POINT('Ctrl Pts',(-5.30566909132792,-0.71897659277826,
1.11186797180717));
#12511=CARTESIAN_POINT('Ctrl Pts',(-4.31506488185325,-3.16974261036297,
1.25081244841436));
#12512=CARTESIAN_POINT('Ctrl Pts',(-2.27267468398946,-4.84788532362214,
1.38975692502155));
#12513=CARTESIAN_POINT('Ctrl Pts',(0.323675729076908,-5.3443695323507,1.52870140162873));
#12514=CARTESIAN_POINT('Ctrl Pts',(2.84113049893774,-4.53817403915035,1.66764587823592));
#12515=CARTESIAN_POINT('Ctrl Pts',(4.66606619309411,-2.62580938898832,1.80659035484311));
#12516=CARTESIAN_POINT('Ctrl Pts',(5.35365846228852,-0.073409129846628,
1.94553483145029));
#12517=CARTESIAN_POINT('Ctrl Pts',(4.73630836736869,2.49688425172971,2.08447930805749));
#12518=CARTESIAN_POINT('Ctrl Pts',(2.96449354959961,4.45856771298933,2.22342378466467));
#12519=CARTESIAN_POINT('Ctrl Pts',(0.470089995263518,5.33348509944276,2.36236826127186));
#12520=CARTESIAN_POINT('Ctrl Pts',(-2.13889696337894,4.90837730673373,2.50131273787904));
#12521=CARTESIAN_POINT('Ctrl Pts',(-4.22653251122924,3.28686338162061,2.64025721448623));
#12522=CARTESIAN_POINT('Ctrl Pts',(-5.28396010317908,0.864183778737327,
2.77920169109342));
#12523=CARTESIAN_POINT('Ctrl Pts',(-5.05343409817609,-1.76913871345001,
2.9181461677006));
#12524=CARTESIAN_POINT('Ctrl Pts',(-3.59114470180712,-3.97123755285457,
3.05709064430779));
#12525=CARTESIAN_POINT('Ctrl Pts',(-1.25352172162997,-5.20535601723436,
3.19603512091497));
#12526=CARTESIAN_POINT('Ctrl Pts',(1.38964440741605,-5.17068045735624,3.33497959752217));
#12527=CARTESIAN_POINT('Ctrl Pts',(3.69408778374435,-3.87566296496448,3.47392407412935));
#12528=CARTESIAN_POINT('Ctrl Pts',(5.09810542778582,-1.63596119111572,3.61286855073654));
#12529=CARTESIAN_POINT('Ctrl Pts',(5.25947114215003,1.0025025070482,3.75181302734373));
#12530=CARTESIAN_POINT('Ctrl Pts',(4.13885239060241,3.39660843497763,3.89075750395091));
#12531=CARTESIAN_POINT('Ctrl Pts',(2.00939751694447,4.96279856438097,4.0297019805581));
#12532=CARTESIAN_POINT('Ctrl Pts',(-0.609843560104704,5.31931751298505,
4.16864645716528));
#12533=CARTESIAN_POINT('Ctrl Pts',(-3.0804366173129,4.37926457506889,4.30759093377247));
#12534=CARTESIAN_POINT('Ctrl Pts',(-4.80018005773276,2.3717755764589,4.44653541037966));
#12535=CARTESIAN_POINT('Ctrl Pts',(-5.34989021890557,-0.213828476584512,
4.58547988698684));
#12536=CARTESIAN_POINT('Ctrl Pts',(-4.5955764640689,-2.74731231108447,4.72442436359404));
#12537=CARTESIAN_POINT('Ctrl Pts',(-2.72110110370615,-4.61114484213517,
4.86336884020122));
#12538=CARTESIAN_POINT('Ctrl Pts',(-0.183363363757842,-5.35102100991686,
5.00231331680841));
#12539=CARTESIAN_POINT('Ctrl Pts',(2.3990687908189,-4.78659763387935,5.14125779341559));
#12540=CARTESIAN_POINT('Ctrl Pts',(4.39673323028909,-3.0554516643881,5.28020227002279));
#12541=CARTESIAN_POINT('Ctrl Pts',(5.32270366296445,-0.579546105159232,
5.41914674662996));
#12542=CARTESIAN_POINT('Ctrl Pts',(4.95127684255042,2.03762253623294,5.55809122323716));
#12543=CARTESIAN_POINT('Ctrl Pts',(3.37298723555918,4.15812518817019,5.69703569984434));
#12544=CARTESIAN_POINT('Ctrl Pts',(0.97253944520539,5.26509401618431,5.83598017645153));
#12545=CARTESIAN_POINT('Ctrl Pts',(-1.66496268531579,5.08870781517731,5.97492465305872));
#12546=CARTESIAN_POINT('Ctrl Pts',(-3.89663384135399,3.67196033177855,6.1138691296659));
#12547=CARTESIAN_POINT('Ctrl Pts',(-5.17850911128188,1.36018063363326,6.2528136062731));
#12548=CARTESIAN_POINT('Ctrl Pts',(-5.19813423138016,-1.28314008755638,
6.39175808288028));
#12549=CARTESIAN_POINT('Ctrl Pts',(-3.95072562200224,-3.61369824852538,
6.53070255948746));
#12550=CARTESIAN_POINT('Ctrl Pts',(-1.74033637453994,-5.06342544876427,
6.66964703609465));
#12551=CARTESIAN_POINT('Ctrl Pts',(0.894256017555476,-5.27895388754308,
6.80859151270184));
#12552=CARTESIAN_POINT('Ctrl Pts',(3.31087548194349,-4.20774898429146,6.94753598930903));
#12553=CARTESIAN_POINT('Ctrl Pts',(4.92047636562735,-2.11091456649553,7.08648046591621));
#12554=CARTESIAN_POINT('Ctrl Pts',(5.33072201090579,0.500450611134641,7.2254249425234));
#12555=CARTESIAN_POINT('Ctrl Pts',(4.44161594850704,2.98983205844547,7.36436941913058));
#12556=CARTESIAN_POINT('Ctrl Pts',(2.46987581595201,4.75044854992828,7.50331389573778));
#12557=CARTESIAN_POINT('Ctrl Pts',(-0.103891087581167,5.35315370727028,
7.64225837234496));
#12558=CARTESIAN_POINT('Ctrl Pts',(-2.65233476814663,4.65103948052701,7.78120284895214));
#12559=CARTESIAN_POINT('Ctrl Pts',(-4.55427771142509,2.81524466058586,7.92014732555934));
#12560=CARTESIAN_POINT('Ctrl Pts',(-5.34612552885195,0.293240177154901,
8.05909180216652));
#12561=CARTESIAN_POINT('Ctrl Pts',(-4.83486706514864,-2.30024095130953,
8.19803627877371));
#12562=CARTESIAN_POINT('Ctrl Pts',(-3.14512044080958,-4.33304343210892,
8.33698075538089));
#12563=CARTESIAN_POINT('Ctrl Pts',(-0.688757660674787,-5.30967615364648,
8.47592523198808));
#12564=CARTESIAN_POINT('Ctrl Pts',(1.93548827689021,-4.99208704869627,8.61486970859527));
#12565=CARTESIAN_POINT('Ctrl Pts',(4.08796322496798,-3.45768775962346,8.75381418520246));
#12566=CARTESIAN_POINT('Ctrl Pts',(5.24400617257436,-1.08048472166078,8.89275866180964));
#12567=CARTESIAN_POINT('Ctrl Pts',(5.12183420642909,1.5600840790141,9.03170313841683));
#12568=CARTESIAN_POINT('Ctrl Pts',(3.75122647324369,3.82038583367911,9.17064761502402));
#12569=CARTESIAN_POINT('Ctrl Pts',(1.46626557853135,5.14947698557384,9.3095920916312));
#12570=CARTESIAN_POINT('Ctrl Pts',(-1.176094310065,5.22339450411064,9.4485365682384));
#12571=CARTESIAN_POINT('Ctrl Pts',(-3.53178381010122,4.02412115752588,9.58748104484557));
#12572=CARTESIAN_POINT('Ctrl Pts',(-5.02660881271791,1.84397717329882,9.72642552145276));
#12573=CARTESIAN_POINT('Ctrl Pts',(-5.29620902753513,-0.785632171181832,
9.86536999805996));
#12574=CARTESIAN_POINT('Ctrl Pts',(-4.27486999808783,-3.22374541041766,
10.0043144746671));
#12575=CARTESIAN_POINT('Ctrl Pts',(-2.21154085534078,-4.87607783130038,
10.1432589512744));
#12576=CARTESIAN_POINT('Ctrl Pts',(0.390846482732544,-5.33987705838589,
10.2822034278815));
#12577=CARTESIAN_POINT('Ctrl Pts',(2.89796585452676,-4.50209305520636,10.4211479044887));
#12578=CARTESIAN_POINT('Ctrl Pts',(4.69871245464655,-2.56693382078497,10.5600923810959));
#12579=CARTESIAN_POINT('Ctrl Pts',(5.3541582794983,-0.0060901412344418,
10.6990368577031));
#12580=CARTESIAN_POINT('Ctrl Pts',(4.70453985800457,2.55623799678097,10.8379813343103));
#12581=CARTESIAN_POINT('Ctrl Pts',(2.90820024455455,4.49548877312727,10.9769258109175));
#12582=CARTESIAN_POINT('Ctrl Pts',(0.402993249481863,5.33897409739104,11.1158702875246));
#12583=CARTESIAN_POINT('Ctrl Pts',(-2.20044245941706,4.88109628613643,11.2548147641319));
#12584=CARTESIAN_POINT('Ctrl Pts',(-4.26752518246539,3.23346204381065,11.393759240739));
#12585=CARTESIAN_POINT('Ctrl Pts',(-5.29440807478772,0.797678575218822,
11.5327037173462));
#12586=CARTESIAN_POINT('Ctrl Pts',(-5.03079070109704,-1.83253728297569,
11.6716481939534));
#12587=CARTESIAN_POINT('Ctrl Pts',(-3.54092921355771,-4.0160762288973,11.8105926705606));
#12588=CARTESIAN_POINT('Ctrl Pts',(-1.18797405672042,-5.22070547074815,
11.9495371471678));
#12589=CARTESIAN_POINT('Ctrl Pts',(1.4545471506665,-5.15279929341601,12.088481623775));
#12590=CARTESIAN_POINT('Ctrl Pts',(3.74252570506027,-3.8289096775327,12.2274261003821));
#12591=CARTESIAN_POINT('Ctrl Pts',(5.11827189094052,-1.57173179078,12.3663705769893));
#12592=CARTESIAN_POINT('Ctrl Pts',(5.24645061630721,1.06855224598058,12.5053150535965));
#12593=CARTESIAN_POINT('Ctrl Pts',(4.0958186001653,3.44837903460169,12.6442595302037));
#12594=CARTESIAN_POINT('Ctrl Pts',(1.94683985321038,4.98767105548193,12.7832040068109));
#12595=CARTESIAN_POINT('Ctrl Pts',(-0.676676804869458,5.31122928082493,
12.9221484834181));
#12596=CARTESIAN_POINT('Ctrl Pts',(-3.13525498741935,4.34018710836324,13.0610929600253));
#12597=CARTESIAN_POINT('Ctrl Pts',(-4.8296216966318,2.31123392134241,13.2000374366325));
#12598=CARTESIAN_POINT('Ctrl Pts',(-5.34677879219064,-0.281077425491243,
13.3389819132396));
#12599=CARTESIAN_POINT('Ctrl Pts',(-4.56067037512442,-2.80487677112613,
13.4779263898468));
#12600=CARTESIAN_POINT('Ctrl Pts',(-2.66290863455959,-4.64499360341092,
13.616870866454));
#12601=CARTESIAN_POINT('Ctrl Pts',(-0.116068800140973,-5.35290351168169,
13.7558153430612));
#12602=CARTESIAN_POINT('Ctrl Pts',(2.45906254776543,-4.75605502048891,13.8947598196684));
#12603=CARTESIAN_POINT('Ctrl Pts',(4.43480283491366,-2.99992863034811,14.0337042962756));
#12604=CARTESIAN_POINT('Ctrl Pts',(5.32956973328494,-0.51257626729447,14.1726487728828));
#12605=CARTESIAN_POINT('Ctrl Pts',(4.92526578910227,2.09971542796619,14.3115932494899));
#12606=CARTESIAN_POINT('Ctrl Pts',(3.3204391951282,4.20020612865568,14.4505377260972));
#12607=CARTESIAN_POINT('Ctrl Pts',(0.906262886499855,5.27690586919013,14.5894822027043));
#12608=CARTESIAN_POINT('Ctrl Pts',(-1.72881299760231,5.06737146764097,14.7284266793115));
#12609=CARTESIAN_POINT('Ctrl Pts',(-3.94249453472985,3.62267647125239,14.8673711559187));
#12610=CARTESIAN_POINT('Ctrl Pts',(-5.19520174310249,1.29496209218852,15.0063156325259));
#12611=CARTESIAN_POINT('Ctrl Pts',(-5.18159000953491,-1.34839643459491,
15.1452601091331));
#12612=CARTESIAN_POINT('Ctrl Pts',(-3.90497716399828,-3.663086310803,15.2842045857403));
#12613=CARTESIAN_POINT('Ctrl Pts',(-1.67653476589803,-5.08490699526312,
15.4231490623474));
#12614=CARTESIAN_POINT('Ctrl Pts',(0.960559275749421,-5.26729283878464,
15.5620935389546));
#12615=CARTESIAN_POINT('Ctrl Pts',(3.36351911705462,-4.16578769513627,15.7010380155618));
#12616=CARTESIAN_POINT('Ctrl Pts',(4.9466286079554,-2.04888100842811,15.839982492169));
#12617=CARTESIAN_POINT('Ctrl Pts',(5.3240083091875,0.567435895447707,15.9789269687762));
#12618=CARTESIAN_POINT('Ctrl Pts',(4.40367275269707,3.04544155401079,16.1178714453834));
#12619=CARTESIAN_POINT('Ctrl Pts',(2.40995169616313,4.78112756511432,16.2568159219906));
#12620=CARTESIAN_POINT('Ctrl Pts',(-0.171189759600305,5.35142429993724,
16.3957603985978));
#12621=CARTESIAN_POINT('Ctrl Pts',(-2.71060408984193,4.61732318988572,16.5347048752049));
#12622=CARTESIAN_POINT('Ctrl Pts',(-4.58931466442483,2.75775975796512,16.6736493518122));
#12623=CARTESIAN_POINT('Ctrl Pts',(-5.34938993330653,0.225998480494149,
16.8125938284193));
#12624=CARTESIAN_POINT('Ctrl Pts',(-4.8055632296837,-2.36084942704272,16.9515383050265));
#12625=CARTESIAN_POINT('Ctrl Pts',(-3.09039111055703,-4.37224550497758,
17.0904827816337));
#12626=CARTESIAN_POINT('Ctrl Pts',(-0.62194298890082,-5.31791640491889,
17.2294272582409));
#12627=CARTESIAN_POINT('Ctrl Pts',(1.99810236159196,-4.96735693557013,17.3683717348481));
#12628=CARTESIAN_POINT('Ctrl Pts',(4.13111467790414,-3.40601519205724,17.5073162114553));
#12629=CARTESIAN_POINT('Ctrl Pts',(5.25717692235762,-1.01446477468014,17.6462606880624));
#12630=CARTESIAN_POINT('Ctrl Pts',(5.10181391213023,1.62435919100904,17.7852051646696));
#12631=CARTESIAN_POINT('Ctrl Pts',(3.7028950369171,3.86724919076739,17.9241496412768));
#12632=CARTESIAN_POINT('Ctrl Pts',(1.4014036817988,5.16750575479613,18.063094117884));
#12633=CARTESIAN_POINT('Ctrl Pts',(-1.24167672489521,5.20819419957418,18.2020385944912));
#12634=CARTESIAN_POINT('Ctrl Pts',(-3.58210117112083,3.97939684585284,18.3409830710984));
#12635=CARTESIAN_POINT('Ctrl Pts',(-5.04939638077243,1.78063025560751,18.4799275477056));
#12636=CARTESIAN_POINT('Ctrl Pts',(-5.28591237076347,-0.852160923645241,
18.6188720243127));
#12637=CARTESIAN_POINT('Ctrl Pts',(-4.23399892837806,-3.27723995766688,
18.7578165009199));
#12638=CARTESIAN_POINT('Ctrl Pts',(-2.15005755740551,-4.90349861032466,
18.8967609775271));
#12639=CARTESIAN_POINT('Ctrl Pts',(0.457955496349907,-5.33454107110207,
19.0357054541343));
#12640=CARTESIAN_POINT('Ctrl Pts',(2.95434309566094,-4.4652994528204,19.1746499307415));
#12641=CARTESIAN_POINT('Ctrl Pts',(4.73061573122731,-2.50765387444491,19.3135944073487));
#12642=CARTESIAN_POINT('Ctrl Pts',(5.35381195296333,0.0612325072370531,
19.4525388839559));
#12643=CARTESIAN_POINT('Ctrl Pts',(4.67202694242282,2.61518238775666,19.591483360563));
#12644=CARTESIAN_POINT('Ctrl Pts',(2.85144844297689,4.53170934500242,19.7304278371702));
#12645=CARTESIAN_POINT('Ctrl Pts',(0.335830287665,5.34359898636174,19.8693723137774));
#12646=CARTESIAN_POINT('Ctrl Pts',(-2.261635153541,4.85308293633194,20.0083167903846));
#12647=CARTESIAN_POINT('Ctrl Pts',(-4.30785291211701,3.1794721341265,20.1472612669918));
#12648=CARTESIAN_POINT('Ctrl Pts',(-5.30399919630087,0.731201050000791,
20.286205743599));
#12649=CARTESIAN_POINT('Ctrl Pts',(-5.00739898838945,-1.89596936210377,
20.4251502202062));
#12650=CARTESIAN_POINT('Ctrl Pts',(-3.99577265594572,-3.33825103356245,
20.5177798712776));
#12651=CARTESIAN_POINT('Ctrl Pts',(-3.34807986563007,-3.89499774607468,
20.5640946968134));
#12652=CARTESIAN_POINT('Ctrl Pts',(4.12541174102849,-3.57975632042981,-0.187812896454475));
#12653=CARTESIAN_POINT('Ctrl Pts',(4.72075895114229,-2.89366314347346,-0.141492274727428));
#12654=CARTESIAN_POINT('Ctrl Pts',(5.56187184080512,-1.2195007812789,-0.0488568274646514));
#12655=CARTESIAN_POINT('Ctrl Pts',(5.46711885657024,1.59059106002505,0.0900934453338543));
#12656=CARTESIAN_POINT('Ctrl Pts',(4.03997190019308,4.01217117600349,0.229037921941041));
#12657=CARTESIAN_POINT('Ctrl Pts',(1.62799574627811,5.45613312141676,0.367982398548228));
#12658=CARTESIAN_POINT('Ctrl Pts',(-1.18075301342602,5.57000272376648,0.506926875155415));
#12659=CARTESIAN_POINT('Ctrl Pts',(-3.70172011600548,4.32628399768095,0.645871351762602));
#12660=CARTESIAN_POINT('Ctrl Pts',(-5.32038875431141,2.02799851661506,0.784815828369788));
#12661=CARTESIAN_POINT('Ctrl Pts',(-5.64223069560639,-0.76458439668364,
0.923760304976975));
#12662=CARTESIAN_POINT('Ctrl Pts',(-4.58878816429013,-3.37081313318115,
1.06270478158417));
#12663=CARTESIAN_POINT('Ctrl Pts',(-2.41684029712518,-5.15540771783689,
1.20164925819134));
#12664=CARTESIAN_POINT('Ctrl Pts',(0.344207884544761,-5.68338607346986,
1.34059373479854));
#12665=CARTESIAN_POINT('Ctrl Pts',(3.02135573014372,-4.82605010319058,1.47953821140572));
#12666=CARTESIAN_POINT('Ctrl Pts',(4.96205501120267,-2.79237586821557,1.61848268801291));
#12667=CARTESIAN_POINT('Ctrl Pts',(5.69326424052521,-0.0780657893714859,
1.75742716462009));
#12668=CARTESIAN_POINT('Ctrl Pts',(5.03675295127321,2.65527245027631,1.89637164122728));
#12669=CARTESIAN_POINT('Ctrl Pts',(3.15254423420737,4.74139400246158,2.03531611783446));
#12670=CARTESIAN_POINT('Ctrl Pts',(0.499909842720598,5.67181119377037,2.17426059444165));
#12671=CARTESIAN_POINT('Ctrl Pts',(-2.27457647542348,5.21973696982665,2.31320507104884));
#12672=CARTESIAN_POINT('Ctrl Pts',(-4.49463980138035,3.49536338298151,2.45214954765603));
#12673=CARTESIAN_POINT('Ctrl Pts',(-5.61914461217458,0.919002704297289,
2.59109402426322));
#12674=CARTESIAN_POINT('Ctrl Pts',(-5.37399534274702,-1.88136285584198,
2.7300385008704));
#12675=CARTESIAN_POINT('Ctrl Pts',(-3.81894658715497,-4.2231503764312,2.86898297747759));
#12676=CARTESIAN_POINT('Ctrl Pts',(-1.33303804169586,-5.53555432810611,
3.00792745408478));
#12677=CARTESIAN_POINT('Ctrl Pts',(1.47779557988571,-5.49867914705657,3.14687193069196));
#12678=CARTESIAN_POINT('Ctrl Pts',(3.92841979530433,-4.12151307786789,3.28581640729915));
#12679=CARTESIAN_POINT('Ctrl Pts',(5.42150036855981,-1.73973730559658,3.42476088390633));
#12680=CARTESIAN_POINT('Ctrl Pts',(5.59310221012439,1.06609558951481,3.56370536051352));
#12681=CARTESIAN_POINT('Ctrl Pts',(4.40139775038178,3.61207004110198,3.70264983712071));
#12682=CARTESIAN_POINT('Ctrl Pts',(2.1368623173862,5.27761040390352,3.8415943137279));
#12683=CARTESIAN_POINT('Ctrl Pts',(-0.64852858237328,5.65674489585048,3.98053879033508));
#12684=CARTESIAN_POINT('Ctrl Pts',(-3.27584207361916,4.65706032251836,4.11948326694227));
#12685=CARTESIAN_POINT('Ctrl Pts',(-5.10467630000627,2.52222758906297,4.25842774354946));
#12686=CARTESIAN_POINT('Ctrl Pts',(-5.6892569611194,-0.227392544354466,
4.39737222015664));
#12687=CARTESIAN_POINT('Ctrl Pts',(-4.88709381290986,-2.9215862476901,4.53631669676383));
#12688=CARTESIAN_POINT('Ctrl Pts',(-2.89371234973432,-4.90364976072612,
4.67526117337102));
#12689=CARTESIAN_POINT('Ctrl Pts',(-0.194994897276038,-5.69045948310944,
4.81420564997821));
#12690=CARTESIAN_POINT('Ctrl Pts',(2.55125213039659,-5.09023228409283,4.9531501265854));
#12691=CARTESIAN_POINT('Ctrl Pts',(4.67563709031104,-3.24927221675587,5.09209460319257));
#12692=CARTESIAN_POINT('Ctrl Pts',(5.66034584401081,-0.616309228442691,
5.23103907979977));
#12693=CARTESIAN_POINT('Ctrl Pts',(5.26535780928076,2.1668777720767,5.36998355640696));
#12694=CARTESIAN_POINT('Ctrl Pts',(3.58695044654535,4.42189310509675,5.50892803301416));
#12695=CARTESIAN_POINT('Ctrl Pts',(1.03423184069184,5.59908176744841,5.64787250962132));
#12696=CARTESIAN_POINT('Ctrl Pts',(-1.77057849037035,5.41150662462054,5.78681698622853));
#12697=CARTESIAN_POINT('Ctrl Pts',(-4.14381422790984,3.90488870308054,5.92576146283571));
#12698=CARTESIAN_POINT('Ctrl Pts',(-5.5070044064582,1.44646279113011,6.0647059394429));
#12699=CARTESIAN_POINT('Ctrl Pts',(-5.52787443305004,-1.36453522904529,
6.20365041605009));
#12700=CARTESIAN_POINT('Ctrl Pts',(-4.20133728483256,-3.8429308031696,6.34259489265727));
#12701=CARTESIAN_POINT('Ctrl Pts',(-1.85073345964212,-5.38462048804139,
6.48153936926446));
#12702=CARTESIAN_POINT('Ctrl Pts',(0.950982555664699,-5.61382083056589,
6.62048384587164));
#12703=CARTESIAN_POINT('Ctrl Pts',(3.52089867498252,-4.47466475385366,6.75942832247883));
#12704=CARTESIAN_POINT('Ctrl Pts',(5.23260352450663,-2.24481903372962,6.89837279908602));
#12705=CARTESIAN_POINT('Ctrl Pts',(5.66887283054235,0.532196364148326,7.0373172756932));
#12706=CARTESIAN_POINT('Ctrl Pts',(4.72336691402839,3.17949007457737,7.17626175230039));
#12707=CARTESIAN_POINT('Ctrl Pts',(2.6265507522657,5.05179010694687,7.31520622890758));
#12708=CARTESIAN_POINT('Ctrl Pts',(-0.110481349903347,5.69272746670676,
7.45415070551477));
#12709=CARTESIAN_POINT('Ctrl Pts',(-2.82058386723012,4.94607508907772,7.59309518212195));
#12710=CARTESIAN_POINT('Ctrl Pts',(-4.84317530124881,2.99382784078302,7.73203965872915));
#12711=CARTESIAN_POINT('Ctrl Pts',(-5.685253460446,0.311841673547404,7.87098413533632));
#12712=CARTESIAN_POINT('Ctrl Pts',(-5.14156365476053,-2.44615521235253,
8.00992861194351));
#12713=CARTESIAN_POINT('Ctrl Pts',(-3.34462907261211,-4.60790717197209,
8.1488730885507));
#12714=CARTESIAN_POINT('Ctrl Pts',(-0.732448546639514,-5.64649194326881,
8.28781756515788));
#12715=CARTESIAN_POINT('Ctrl Pts',(2.05826469364734,-5.30875678382038,8.42676204176508));
#12716=CARTESIAN_POINT('Ctrl Pts',(4.34728046423481,-3.67702389224715,8.56570651837225));
#12717=CARTESIAN_POINT('Ctrl Pts',(5.57665623044785,-1.14902455425511,8.70465099497944));
#12718=CARTESIAN_POINT('Ctrl Pts',(5.44673436655812,1.65904697915057,8.84359547158665));
#12719=CARTESIAN_POINT('Ctrl Pts',(3.98918303972281,4.06272947837557,8.98253994819381));
#12720=CARTESIAN_POINT('Ctrl Pts',(1.55927716423605,5.47613064708706,9.12148442480103));
#12721=CARTESIAN_POINT('Ctrl Pts',(-1.25069907356697,5.5547370744485,9.26042890140818));
#12722=CARTESIAN_POINT('Ctrl Pts',(-3.75582017660497,4.27938861753417,9.39937337801538));
#12723=CARTESIAN_POINT('Ctrl Pts',(-5.34546841307515,1.96094864381752,9.53831785462256));
#12724=CARTESIAN_POINT('Ctrl Pts',(-5.63217053893333,-0.835468227549896,
9.67726233122977));
#12725=CARTESIAN_POINT('Ctrl Pts',(-4.54604354469856,-3.4282415650853,9.81620680783694));
#12726=CARTESIAN_POINT('Ctrl Pts',(-2.35182848455184,-5.18538859856469,
9.95515128444412));
#12727=CARTESIAN_POINT('Ctrl Pts',(0.415639570463942,-5.67860862239497,
10.0940957610513));
#12728=CARTESIAN_POINT('Ctrl Pts',(3.0817963988662,-4.7876803459305,10.2330402376585));
#12729=CARTESIAN_POINT('Ctrl Pts',(4.99677216673147,-2.72976556734303,10.3719847142657));
#12730=CARTESIAN_POINT('Ctrl Pts',(5.69379576330861,-0.00647646530947798,
10.5109291908729));
#12731=CARTESIAN_POINT('Ctrl Pts',(5.00296922756137,2.71839126082836,10.6498736674801));
#12732=CARTESIAN_POINT('Ctrl Pts',(3.09268000064603,4.78065712559247,10.7888181440872));
#12733=CARTESIAN_POINT('Ctrl Pts',(0.428556859315862,5.67764838266755,10.9277626206944));
#12734=CARTESIAN_POINT('Ctrl Pts',(-2.34002606923442,5.19072539575898,11.0667070973016));
#12735=CARTESIAN_POINT('Ctrl Pts',(-4.53823281556239,3.43857456668117,11.2056515739088));
#12736=CARTESIAN_POINT('Ctrl Pts',(-5.63025534394137,0.848278787247312,
11.344596050516));
#12737=CARTESIAN_POINT('Ctrl Pts',(-5.34991557677349,-1.94878307162965,
11.4835405271232));
#12738=CARTESIAN_POINT('Ctrl Pts',(-3.76554571267171,-4.2708333641871,11.6224850037304));
#12739=CARTESIAN_POINT('Ctrl Pts',(-1.26333240408221,-5.55187746403591,
11.7614294803376));
#12740=CARTESIAN_POINT('Ctrl Pts',(1.546815385662,-5.47966370332645,11.9003739569447));
#12741=CARTESIAN_POINT('Ctrl Pts',(3.97993034407314,-4.07179402661772,12.0393184335519));
#12742=CARTESIAN_POINT('Ctrl Pts',(5.44294607794625,-1.67143355579679,12.1782629101591));
#12743=CARTESIAN_POINT('Ctrl Pts',(5.57925573584966,1.13633514988432,12.3172073867663));
#12744=CARTESIAN_POINT('Ctrl Pts',(4.35563413995431,3.66712467441981,12.4561518633735));
#12745=CARTESIAN_POINT('Ctrl Pts',(2.07033634969198,5.30406066500168,12.5950963399807));
#12746=CARTESIAN_POINT('Ctrl Pts',(-0.719601349748659,5.64814359204101,
12.7340408165879));
#12747=CARTESIAN_POINT('Ctrl Pts',(-3.33413781072106,4.61550400259756,12.872985293195));
#12748=CARTESIAN_POINT('Ctrl Pts',(-5.13598554976642,2.45784551415759,13.0119297698022));
#12749=CARTESIAN_POINT('Ctrl Pts',(-5.68594816311183,-0.298907385788696,
13.1508742464094));
#12750=CARTESIAN_POINT('Ctrl Pts',(-4.84997347933535,-2.98280227112322,
13.2898187230166));
#12751=CARTESIAN_POINT('Ctrl Pts',(-2.83182847985474,-4.93964569575163,
13.4287631996238));
#12752=CARTESIAN_POINT('Ctrl Pts',(-0.123431547592747,-5.69246140012673,
13.567707676231));
#12753=CARTESIAN_POINT('Ctrl Pts',(2.61505155157454,-5.05775222025373,13.7066521528382));
#12754=CARTESIAN_POINT('Ctrl Pts',(4.71612161508726,-3.19022711583059,13.8455966294454));
#12755=CARTESIAN_POINT('Ctrl Pts',(5.66764745895392,-0.54509120327449,13.9845411060525));
#12756=CARTESIAN_POINT('Ctrl Pts',(5.23769676188712,2.23290948526608,14.1234855826597));
#12757=CARTESIAN_POINT('Ctrl Pts',(3.53106905597799,4.46664342216709,14.2624300592669));
#12758=CARTESIAN_POINT('Ctrl Pts',(0.963751072387092,5.61164289752535,14.4013745358741));
#12759=CARTESIAN_POINT('Ctrl Pts',(-1.83847910492166,5.38881682001165,14.5403190124813));
#12760=CARTESIAN_POINT('Ctrl Pts',(-4.1925840639914,3.85247855350803,14.6792634890885));
#12761=CARTESIAN_POINT('Ctrl Pts',(-5.52475592432099,1.37710715471025,14.8182079656957));
#12762=CARTESIAN_POINT('Ctrl Pts',(-5.5102807394511,-1.43393106923174,14.9571524423028));
#12763=CARTESIAN_POINT('Ctrl Pts',(-4.15268680369936,-3.89545176446264,
15.0960969189101));
#12764=CARTESIAN_POINT('Ctrl Pts',(-1.78288463821885,-5.4074647022128,15.2350413955172));
#12765=CARTESIAN_POINT('Ctrl Pts',(1.02149171712221,-5.60142007090385,15.3739858721244));
#12766=CARTESIAN_POINT('Ctrl Pts',(3.57688172421524,-4.43004167811651,15.5129303487316));
#12767=CARTESIAN_POINT('Ctrl Pts',(5.26041471700324,-2.17885041799783,15.6518748253388));
#12768=CARTESIAN_POINT('Ctrl Pts',(5.66173324960281,0.603430815600041,15.790819301946));
#12769=CARTESIAN_POINT('Ctrl Pts',(4.68301681672617,3.23862712165757,15.9297637785531));
#12770=CARTESIAN_POINT('Ctrl Pts',(2.56282538563238,5.08441522513913,16.0687082551604));
#12771=CARTESIAN_POINT('Ctrl Pts',(-0.18204906860269,5.6908883555651,16.2076527317675));
#12772=CARTESIAN_POINT('Ctrl Pts',(-2.88254946474894,4.91022002787362,16.3465972083747));
#12773=CARTESIAN_POINT('Ctrl Pts',(-4.88043480015326,2.93269642144313,16.4855416849819));
#12774=CARTESIAN_POINT('Ctrl Pts',(-5.68872494023477,0.24033454440057,16.6244861615891));
#12775=CARTESIAN_POINT('Ctrl Pts',(-5.11040094990405,-2.51060834659618,
16.7634306381963));
#12776=CARTESIAN_POINT('Ctrl Pts',(-3.28642802354827,-4.64959600236532,
16.9023751148035));
#12777=CARTESIAN_POINT('Ctrl Pts',(-0.661395530420292,-5.65525490942225,
17.0413195914106));
#12778=CARTESIAN_POINT('Ctrl Pts',(2.12485066133594,-5.28245793234956,17.1802640680179));
#12779=CARTESIAN_POINT('Ctrl Pts',(4.39316920100402,-3.6220735095858,17.319208544625));
#12780=CARTESIAN_POINT('Ctrl Pts',(5.59066245801917,-1.07881667567005,17.4581530212322));
#12781=CARTESIAN_POINT('Ctrl Pts',(5.42544409815205,1.72739934029841,17.5970974978394));
#12782=CARTESIAN_POINT('Ctrl Pts',(3.93778573074807,4.11256558147797,17.7360419744466));
#12783=CARTESIAN_POINT('Ctrl Pts',(1.49030079604946,5.49530305934251,17.8749864510538));
#12784=CARTESIAN_POINT('Ctrl Pts',(-1.32044166543948,5.53857254866263,18.0139309276609));
#12785=CARTESIAN_POINT('Ctrl Pts',(-3.80932938609013,4.231827248776,18.1528754042682));
#12786=CARTESIAN_POINT('Ctrl Pts',(-5.36970149541447,1.89358335636413,18.2918198808753));
#12787=CARTESIAN_POINT('Ctrl Pts',(-5.62122072056,-0.906217187356495,18.4307643574825));
#12788=CARTESIAN_POINT('Ctrl Pts',(-4.50257984575516,-3.48512950350393,
18.5697088340897));
#12789=CARTESIAN_POINT('Ctrl Pts',(-2.28644503433923,-5.21454879654256,
18.7086533106969));
#12790=CARTESIAN_POINT('Ctrl Pts',(0.48700559990642,-5.67293415029241,18.8475977873041));
#12791=CARTESIAN_POINT('Ctrl Pts',(3.14174989294686,-4.74855276574965,18.9865422639113));
#12792=CARTESIAN_POINT('Ctrl Pts',(5.03069920652907,-2.66672523687453,19.1254867405184));
#12793=CARTESIAN_POINT('Ctrl Pts',(5.69342746777932,0.0651167507725929,
19.2644312171257));
#12794=CARTESIAN_POINT('Ctrl Pts',(4.96839387671658,2.78107475020022,19.4033756937328));
#12795=CARTESIAN_POINT('Ctrl Pts',(3.03232818612828,4.81917532545164,19.5423201703401));
#12796=CARTESIAN_POINT('Ctrl Pts',(0.357133459505582,5.68256664840653,19.6812646469472));
#12797=CARTESIAN_POINT('Ctrl Pts',(-2.40510048137543,5.16093503766596,19.8202091235544));
#12798=CARTESIAN_POINT('Ctrl Pts',(-4.58111870803096,3.38115984283969,19.9591536001616));
#12799=CARTESIAN_POINT('Ctrl Pts',(-5.64045487189444,0.777584304252472,
20.0980980767688));
#12800=CARTESIAN_POINT('Ctrl Pts',(-5.32504002626521,-2.01623892267917,
20.237042553376));
#12801=CARTESIAN_POINT('Ctrl Pts',(-4.24924184753463,-3.55001077658457,
20.3296722044474));
#12802=CARTESIAN_POINT('Ctrl Pts',(-3.56046309410368,-4.14207434801025,
20.3759870299831));
#12803=CARTESIAN_POINT('Ctrl Pts',(4.37149441094678,-3.79329039855036,-0.375920563284674));
#12804=CARTESIAN_POINT('Ctrl Pts',(5.0023543505019,-3.06627145432599,-0.329599941557627));
#12805=CARTESIAN_POINT('Ctrl Pts',(5.8936400031722,-1.29224455258298,-0.23696449429485));
#12806=CARTESIAN_POINT('Ctrl Pts',(5.79323496071699,1.68547053372857,-0.0980142214963448));
#12807=CARTESIAN_POINT('Ctrl Pts',(4.28095804509276,4.25149899517385,0.0409302551108422));
#12808=CARTESIAN_POINT('Ctrl Pts',(1.72510642637714,5.78159392150968,0.179874731718029));
#12809=CARTESIAN_POINT('Ctrl Pts',(-1.25118546291179,5.90225589696729,0.318819208325216));
#12810=CARTESIAN_POINT('Ctrl Pts',(-3.92252938950839,4.5843487882535,0.457763684932403));
#12811=CARTESIAN_POINT('Ctrl Pts',(-5.63775234171852,2.14896954226947,0.596708161539589));
#12812=CARTESIAN_POINT('Ctrl Pts',(-5.97879229988485,-0.810192200589017,
0.735652638146776));
#12813=CARTESIAN_POINT('Ctrl Pts',(-4.86251144672701,-3.57188365599933,
0.874597114753963));
#12814=CARTESIAN_POINT('Ctrl Pts',(-2.5610059102609,-5.46293011205162,1.01354159136115));
#12815=CARTESIAN_POINT('Ctrl Pts',(0.364740040012614,-6.02240261458903,
1.15248606796834));
#12816=CARTESIAN_POINT('Ctrl Pts',(3.20158096134969,-5.11392616723079,1.29143054457553));
#12817=CARTESIAN_POINT('Ctrl Pts',(5.25804382931122,-2.95894234744282,1.43037502118271));
#12818=CARTESIAN_POINT('Ctrl Pts',(6.0328700187619,-0.0827224488963419,
1.5693194977899));
#12819=CARTESIAN_POINT('Ctrl Pts',(5.33719753517774,2.81366064882291,1.70826397439709));
#12820=CARTESIAN_POINT('Ctrl Pts',(3.34059491881512,5.02422029193383,1.84720845100427));
#12821=CARTESIAN_POINT('Ctrl Pts',(0.529729690177678,6.01013728809799,1.98615292761146));
#12822=CARTESIAN_POINT('Ctrl Pts',(-2.41025598746802,5.53109663291954,2.12509740421865));
#12823=CARTESIAN_POINT('Ctrl Pts',(-4.76274709153145,3.70386338434242,2.26404188082583));
#12824=CARTESIAN_POINT('Ctrl Pts',(-5.95432912117008,0.973821629857239,
2.40298635743302));
#12825=CARTESIAN_POINT('Ctrl Pts',(-5.69455658731797,-1.99358699823395,
2.5419308340402));
#12826=CARTESIAN_POINT('Ctrl Pts',(-4.04674847250281,-4.47506320000782,
2.6808753106474));
#12827=CARTESIAN_POINT('Ctrl Pts',(-1.41255436176173,-5.86575263897786,
2.81981978725458));
#12828=CARTESIAN_POINT('Ctrl Pts',(1.56594675235535,-5.8266778367569,2.95876426386177));
#12829=CARTESIAN_POINT('Ctrl Pts',(4.1627518068643,-4.3673631907713,3.09770874046896));
#12830=CARTESIAN_POINT('Ctrl Pts',(5.74489530933378,-1.84351342007744,3.23665321707614));
#12831=CARTESIAN_POINT('Ctrl Pts',(5.92673327809876,1.12968867198141,3.37559769368333));
#12832=CARTESIAN_POINT('Ctrl Pts',(4.66394311016112,3.82753164722633,3.51454217029051));
#12833=CARTESIAN_POINT('Ctrl Pts',(2.26432711782793,5.59242224342607,3.65348664689771));
#12834=CARTESIAN_POINT('Ctrl Pts',(-0.68721360464186,5.99417227871591,3.79243112350489));
#12835=CARTESIAN_POINT('Ctrl Pts',(-3.47124752992542,4.93485606996784,3.93137560011208));
#12836=CARTESIAN_POINT('Ctrl Pts',(-5.40917254227977,2.67267960166704,4.07032007671926));
#12837=CARTESIAN_POINT('Ctrl Pts',(-6.02862370333322,-0.240956612124415,
4.20926455332645));
#12838=CARTESIAN_POINT('Ctrl Pts',(-5.17861116175084,-3.09586018429574,
4.34820902993364));
#12839=CARTESIAN_POINT('Ctrl Pts',(-3.06632359576249,-5.19615467931707,
4.48715350654083));
#12840=CARTESIAN_POINT('Ctrl Pts',(-0.206626430794233,-6.029897956302,4.626097983148));
#12841=CARTESIAN_POINT('Ctrl Pts',(2.70343546997428,-5.39386693430633,4.76504245975521));
#12842=CARTESIAN_POINT('Ctrl Pts',(4.95454095033299,-3.44309276912364,4.90398693636238));
#12843=CARTESIAN_POINT('Ctrl Pts',(5.99798802505716,-0.653072351726153,
5.04293141296958));
#12844=CARTESIAN_POINT('Ctrl Pts',(5.5794387760111,2.29613300792046,5.18187588957675));
#12845=CARTESIAN_POINT('Ctrl Pts',(3.80091365753151,4.6856610220233,5.32082036618396));
#12846=CARTESIAN_POINT('Ctrl Pts',(1.09592423617828,5.93306951871249,5.45976484279112));
#12847=CARTESIAN_POINT('Ctrl Pts',(-1.8761942954249,5.73430543406377,5.59870931939833));
#12848=CARTESIAN_POINT('Ctrl Pts',(-4.39099461446568,4.13781707438252,5.73765379600551));
#12849=CARTESIAN_POINT('Ctrl Pts',(-5.83549970163454,1.53274494862695,5.87659827261269));
#12850=CARTESIAN_POINT('Ctrl Pts',(-5.85761463471991,-1.4459303705342,6.01554274921988));
#12851=CARTESIAN_POINT('Ctrl Pts',(-4.45194894766288,-4.07216335781382,
6.15448722582707));
#12852=CARTESIAN_POINT('Ctrl Pts',(-1.9611305447443,-5.70581552731852,6.29343170243426));
#12853=CARTESIAN_POINT('Ctrl Pts',(1.00770909377392,-5.94868777358868,6.43237617904144));
#12854=CARTESIAN_POINT('Ctrl Pts',(3.73092186802155,-4.74158052341587,6.57132065564863));
#12855=CARTESIAN_POINT('Ctrl Pts',(5.54473068338591,-2.37872350096367,6.71026513225582));
#12856=CARTESIAN_POINT('Ctrl Pts',(6.00702365017893,0.563942117162005,6.849209608863));
#12857=CARTESIAN_POINT('Ctrl Pts',(5.00511787954972,3.36914809070927,6.98815408547019));
#12858=CARTESIAN_POINT('Ctrl Pts',(2.78322568857942,5.35313166396547,7.12709856207738));
#12859=CARTESIAN_POINT('Ctrl Pts',(-0.117071612225535,6.03230122614323,
7.26604303868457));
#12860=CARTESIAN_POINT('Ctrl Pts',(-2.98883296631359,5.24111069762843,7.40498751529175));
#12861=CARTESIAN_POINT('Ctrl Pts',(-5.13207289107254,3.17241102098019,7.54393199189894));
#12862=CARTESIAN_POINT('Ctrl Pts',(-6.02438139204003,0.330443169939912,
7.68287646850613));
#12863=CARTESIAN_POINT('Ctrl Pts',(-5.44826024437244,-2.59206947339553,
7.82182094511331));
#12864=CARTESIAN_POINT('Ctrl Pts',(-3.54413770441465,-4.88277091183526,
7.96076542172051));
#12865=CARTESIAN_POINT('Ctrl Pts',(-0.776139432604244,-5.98330773289114,
8.09970989832767));
#12866=CARTESIAN_POINT('Ctrl Pts',(2.18104111040448,-5.62542651894447,8.23865437493489));
#12867=CARTESIAN_POINT('Ctrl Pts',(4.60659770350166,-3.89636002487083,8.37759885154205));
#12868=CARTESIAN_POINT('Ctrl Pts',(5.90930628832132,-1.21756438684943,8.51654332814926));
#12869=CARTESIAN_POINT('Ctrl Pts',(5.77163452668715,1.75800987928705,8.65548780475643));
#12870=CARTESIAN_POINT('Ctrl Pts',(4.22713960620191,4.30507312307204,8.79443228136362));
#12871=CARTESIAN_POINT('Ctrl Pts',(1.65228874994075,5.80278430860025,8.93337675797081));
#12872=CARTESIAN_POINT('Ctrl Pts',(-1.32530383706894,5.88607964478638,9.07232123457799));
#12873=CARTESIAN_POINT('Ctrl Pts',(-3.97985654310871,4.53465607754247,9.21126571118519));
#12874=CARTESIAN_POINT('Ctrl Pts',(-5.6643280134324,2.07792011433624,9.35021018779235));
#12875=CARTESIAN_POINT('Ctrl Pts',(-5.96813205033154,-0.885304283917966,
9.48915466439957));
#12876=CARTESIAN_POINT('Ctrl Pts',(-4.81721709130929,-3.63273771975294,
9.62809914100673));
#12877=CARTESIAN_POINT('Ctrl Pts',(-2.49211611376292,-5.49469936582898,
9.76704361761394));
#12878=CARTESIAN_POINT('Ctrl Pts',(0.44043265819534,-6.01734018640404,9.90598809422111));
#12879=CARTESIAN_POINT('Ctrl Pts',(3.26562694320564,-5.07326763665466,10.0449325708283));
#12880=CARTESIAN_POINT('Ctrl Pts',(5.2948318788164,-2.89259731390109,10.1838770474355));
#12881=CARTESIAN_POINT('Ctrl Pts',(6.03343324711893,-0.00686278938451319,
10.3228215240426));
#12882=CARTESIAN_POINT('Ctrl Pts',(5.30139859711817,2.88054452487575,10.4617660006498));
#12883=CARTESIAN_POINT('Ctrl Pts',(3.27715975673751,5.06582547805768,10.600710477257));
#12884=CARTESIAN_POINT('Ctrl Pts',(0.454120469149858,6.01632266794404,10.7396549538642));
#12885=CARTESIAN_POINT('Ctrl Pts',(-2.47960967905176,5.50035450538153,10.8785994304714));
#12886=CARTESIAN_POINT('Ctrl Pts',(-4.8089404486594,3.64368708955169,11.0175439070786));
#12887=CARTESIAN_POINT('Ctrl Pts',(-5.96610261309502,0.898878999275805,
11.1564883836858));
#12888=CARTESIAN_POINT('Ctrl Pts',(-5.66904045244993,-2.06502886028363,
11.2954328602929));
#12889=CARTESIAN_POINT('Ctrl Pts',(-3.99016221178573,-4.52559049947687,
11.4343773369001));
#12890=CARTESIAN_POINT('Ctrl Pts',(-1.33869075144399,-5.88304945732368,
11.5733218135073));
#12891=CARTESIAN_POINT('Ctrl Pts',(1.63908362065749,-5.80652811323691,11.7122662901145));
#12892=CARTESIAN_POINT('Ctrl Pts',(4.21733498308602,-4.31467837570276,11.8512107667217));
#12893=CARTESIAN_POINT('Ctrl Pts',(5.76762026495197,-1.77113532081357,11.9901552433289));
#12894=CARTESIAN_POINT('Ctrl Pts',(5.91206085539211,1.20411805378807,12.1290997199361));
#12895=CARTESIAN_POINT('Ctrl Pts',(4.61544967974331,3.88587031423793,12.2680441965433));
#12896=CARTESIAN_POINT('Ctrl Pts',(2.19383284617359,5.62045027452143,12.4069886731505));
#12897=CARTESIAN_POINT('Ctrl Pts',(-0.762525894627859,5.98505790325709,
12.5459331497576));
#12898=CARTESIAN_POINT('Ctrl Pts',(-3.53302063402278,4.89082089683188,12.6848776263648));
#12899=CARTESIAN_POINT('Ctrl Pts',(-5.44234940290103,2.60445710697275,12.823822102972));
#12900=CARTESIAN_POINT('Ctrl Pts',(-6.02511753403304,-0.316737346086145,
12.9627665795792));
#12901=CARTESIAN_POINT('Ctrl Pts',(-5.13927658354627,-3.16072777112031,
13.1017110561864));
#12902=CARTESIAN_POINT('Ctrl Pts',(-3.00074832514988,-5.23429778809233,
13.2406555327936));
#12903=CARTESIAN_POINT('Ctrl Pts',(-0.130794295044517,-6.03201928857177,
13.3796000094008));
#12904=CARTESIAN_POINT('Ctrl Pts',(2.77104055538365,-5.35944942001855,13.5185444860079));
#12905=CARTESIAN_POINT('Ctrl Pts',(4.99744039526088,-3.38052560131306,13.6574889626151));
#12906=CARTESIAN_POINT('Ctrl Pts',(6.00572518462289,-0.577606139254506,
13.7964334392223));
#12907=CARTESIAN_POINT('Ctrl Pts',(5.55012773467197,2.36610354256596,13.9353779158295));
#12908=CARTESIAN_POINT('Ctrl Pts',(3.74169891682778,4.73308071567851,14.0743223924367));
#12909=CARTESIAN_POINT('Ctrl Pts',(1.02123925827433,5.94637992586056,14.2132668690439));
#12910=CARTESIAN_POINT('Ctrl Pts',(-1.948145212241,5.71026217238234,14.3522113456511));
#12911=CARTESIAN_POINT('Ctrl Pts',(-4.44267359325295,4.08228063576368,14.4911558222582));
#12912=CARTESIAN_POINT('Ctrl Pts',(-5.85431010553948,1.45925221723197,14.6301002988654));
#12913=CARTESIAN_POINT('Ctrl Pts',(-5.8389714693673,-1.51946570386857,14.7690447754726));
#12914=CARTESIAN_POINT('Ctrl Pts',(-4.40039644340045,-4.12781721812228,
14.9079892520798));
#12915=CARTESIAN_POINT('Ctrl Pts',(-1.88923451053967,-5.73002240916248,
15.046933728687));
#12916=CARTESIAN_POINT('Ctrl Pts',(1.08242415849501,-5.93554730302306,15.1858782052942));
#12917=CARTESIAN_POINT('Ctrl Pts',(3.79024433137585,-4.69429566109675,15.3248226819014));
#12918=CARTESIAN_POINT('Ctrl Pts',(5.57420082605109,-2.30881982756756,15.4637671585085));
#12919=CARTESIAN_POINT('Ctrl Pts',(5.9994581900181,0.63942573575238,15.6027116351158));
#12920=CARTESIAN_POINT('Ctrl Pts',(4.96236088075527,3.43181268930434,15.7416561117229));
#12921=CARTESIAN_POINT('Ctrl Pts',(2.71569907510162,5.38770288516396,15.8806005883301));
#12922=CARTESIAN_POINT('Ctrl Pts',(-0.192908377605067,6.03035241119298,
16.0195450649373));
#12923=CARTESIAN_POINT('Ctrl Pts',(-3.05449483965596,5.20311686586152,16.1584895415445));
#12924=CARTESIAN_POINT('Ctrl Pts',(-5.17155493588167,3.10763308492114,16.2974340181517));
#12925=CARTESIAN_POINT('Ctrl Pts',(-6.02805994716301,0.254670608306993,
16.4363784947589));
#12926=CARTESIAN_POINT('Ctrl Pts',(-5.41523867012438,-2.66036726614962,
16.5753229713661));
#12927=CARTESIAN_POINT('Ctrl Pts',(-3.48246493653952,-4.92694649975305,
16.7142674479732));
#12928=CARTESIAN_POINT('Ctrl Pts',(-0.700848071939763,-5.99259341392561,
16.8532119245804));
#12929=CARTESIAN_POINT('Ctrl Pts',(2.25159896107991,-5.59755892912898,16.9921564011876));
#12930=CARTESIAN_POINT('Ctrl Pts',(4.65522372410391,-3.83813182711437,17.1311008777948));
#12931=CARTESIAN_POINT('Ctrl Pts',(5.92414799368071,-1.14316857665995,17.270045354402));
#12932=CARTESIAN_POINT('Ctrl Pts',(5.74907428417388,1.83043948958779,17.4089898310092));
#12933=CARTESIAN_POINT('Ctrl Pts',(4.17267642457904,4.35788197218855,17.5479343076163));
#12934=CARTESIAN_POINT('Ctrl Pts',(1.57919791030011,5.82310036388892,17.6868787842236));
#12935=CARTESIAN_POINT('Ctrl Pts',(-1.39920660598374,5.86895089775106,17.8258232608307));
#12936=CARTESIAN_POINT('Ctrl Pts',(-4.03655760105942,4.48425765169917,17.9647677374379));
#12937=CARTESIAN_POINT('Ctrl Pts',(-5.69000661005654,2.00653645712075,18.1037122140451));
#12938=CARTESIAN_POINT('Ctrl Pts',(-5.9565290703565,-0.960273451067746,
18.2426566906523));
#12939=CARTESIAN_POINT('Ctrl Pts',(-4.77116076313227,-3.69301904934098,
18.3816011672595));
#12940=CARTESIAN_POINT('Ctrl Pts',(-2.42283251127295,-5.52559898276046,
18.5205456438667));
#12941=CARTESIAN_POINT('Ctrl Pts',(0.516055703462933,-6.01132722948276,
18.6594901204738));
#12942=CARTESIAN_POINT('Ctrl Pts',(3.32915669023277,-5.03180607867891,18.7984345970811));
#12943=CARTESIAN_POINT('Ctrl Pts',(5.33078268183083,-2.82579659930416,18.9373790736882));
#12944=CARTESIAN_POINT('Ctrl Pts',(6.03304298259528,0.0690009943081289,
19.0763235502954));
#12945=CARTESIAN_POINT('Ctrl Pts',(5.26476081101034,2.94696711264378,19.2152680269026));
#12946=CARTESIAN_POINT('Ctrl Pts',(3.21320792927966,5.10664130590087,19.3542125035098));
#12947=CARTESIAN_POINT('Ctrl Pts',(0.378436631346168,6.0215343104513,19.493156980117));
#12948=CARTESIAN_POINT('Ctrl Pts',(-2.54856580920985,5.468787139,19.6321014567242));
#12949=CARTESIAN_POINT('Ctrl Pts',(-4.8543845039449,3.58284755155288,19.7710459333314));
#12950=CARTESIAN_POINT('Ctrl Pts',(-5.97691054748803,0.823967558504157,
19.9099904099385));
#12951=CARTESIAN_POINT('Ctrl Pts',(-5.64268106414096,-2.13650848325456,
20.0489348865457));
#12952=CARTESIAN_POINT('Ctrl Pts',(-4.50271103912352,-3.7617705196067,20.1415645376172));
#12953=CARTESIAN_POINT('Ctrl Pts',(-3.7728463225773,-4.38915094994582,20.1878793631529));
#12954=CARTESIAN_POINT('Ctrl Pts',(4.61757708086507,-4.00682447667092,-0.564028230114873));
#12955=CARTESIAN_POINT('Ctrl Pts',(5.28394974986152,-3.23887976517851,-0.517707608387826));
#12956=CARTESIAN_POINT('Ctrl Pts',(6.22540816553931,-1.36498832388706,-0.425072161125049));
#12957=CARTESIAN_POINT('Ctrl Pts',(6.11935106486372,1.7803500074321,-0.286121888326544));
#12958=CARTESIAN_POINT('Ctrl Pts',(4.52194418999246,4.49082681434422,-0.147177411719357));
#12959=CARTESIAN_POINT('Ctrl Pts',(1.82221710647615,6.1070547216026,-0.00823293511216988));
#12960=CARTESIAN_POINT('Ctrl Pts',(-1.32161791239755,6.2345090701681,0.130711541495017));
#12961=CARTESIAN_POINT('Ctrl Pts',(-4.14333866301131,4.84241357882606,0.269656018102203));
#12962=CARTESIAN_POINT('Ctrl Pts',(-5.95511592912563,2.26994056792388,0.40860049470939));
#12963=CARTESIAN_POINT('Ctrl Pts',(-6.31535390416332,-0.855800004494397,
0.547544971316578));
#12964=CARTESIAN_POINT('Ctrl Pts',(-5.1362347291639,-3.77295417881752,0.686489447923763));
#12965=CARTESIAN_POINT('Ctrl Pts',(-2.70517152339663,-5.77045250626636,
0.825433924530953));
#12966=CARTESIAN_POINT('Ctrl Pts',(0.385272195480467,-6.3614191557082,0.964378401138136));
#12967=CARTESIAN_POINT('Ctrl Pts',(3.38180619255566,-5.40180223127101,1.10332287774532));
#12968=CARTESIAN_POINT('Ctrl Pts',(5.55403264741978,-3.12550882667008,1.24226735435251));
#12969=CARTESIAN_POINT('Ctrl Pts',(6.3724757969986,-0.0873791084211981,
1.3812118309597));
#12970=CARTESIAN_POINT('Ctrl Pts',(5.63764211908227,2.9720488473695,1.52015630756688));
#12971=CARTESIAN_POINT('Ctrl Pts',(3.52864560342288,5.30704658140607,1.65910078417407));
#12972=CARTESIAN_POINT('Ctrl Pts',(0.559549537634755,6.34846338242561,1.79804526078126));
#12973=CARTESIAN_POINT('Ctrl Pts',(-2.54593549951255,5.84245629601246,1.93698973738844));
#12974=CARTESIAN_POINT('Ctrl Pts',(-5.03085438168256,3.9123633857033,2.07593421399563));
#12975=CARTESIAN_POINT('Ctrl Pts',(-6.28951363016558,1.0286405554172,2.21487869060282));
#12976=CARTESIAN_POINT('Ctrl Pts',(-6.0151178318889,-2.10581114062593,2.35382316721));
#12977=CARTESIAN_POINT('Ctrl Pts',(-4.27455035785067,-4.72697602358444,
2.49276764381719));
#12978=CARTESIAN_POINT('Ctrl Pts',(-1.49207068182762,-6.19595094984961,
2.63171212042438));
#12979=CARTESIAN_POINT('Ctrl Pts',(1.65409792482501,-6.15467652645724,2.77065659703156));
#12980=CARTESIAN_POINT('Ctrl Pts',(4.39708381842427,-4.61321330367469,2.90960107363875));
#12981=CARTESIAN_POINT('Ctrl Pts',(6.06829025010777,-1.94728953455831,3.04854555024594));
#12982=CARTESIAN_POINT('Ctrl Pts',(6.26036434607312,1.19328175444802,3.18749002685313));
#12983=CARTESIAN_POINT('Ctrl Pts',(4.92648846994049,4.04299325335068,3.32643450346031));
#12984=CARTESIAN_POINT('Ctrl Pts',(2.39179191826967,5.90723408294864,3.4653789800675));
#12985=CARTESIAN_POINT('Ctrl Pts',(-0.725898626910438,6.33159966158133,
3.60432345667468));
#12986=CARTESIAN_POINT('Ctrl Pts',(-3.66665298623168,5.21265181741733,3.74326793328188));
#12987=CARTESIAN_POINT('Ctrl Pts',(-5.71366878455327,2.82313161427111,3.88221240988906));
#12988=CARTESIAN_POINT('Ctrl Pts',(-6.36799044554703,-0.254520679894365,
4.02115688649625));
#12989=CARTESIAN_POINT('Ctrl Pts',(-5.4701285105918,-3.27013412090137,4.16010136310343));
#12990=CARTESIAN_POINT('Ctrl Pts',(-3.23893484179065,-5.48865959790801,
4.29904583971062));
#12991=CARTESIAN_POINT('Ctrl Pts',(-0.218257964312433,-6.36933642949458,
4.43799031631781));
#12992=CARTESIAN_POINT('Ctrl Pts',(2.85561880955198,-5.69750158451984,4.576934792925));
#12993=CARTESIAN_POINT('Ctrl Pts',(5.23344481035494,-3.6369133214914,4.71587926953218));
#12994=CARTESIAN_POINT('Ctrl Pts',(6.33563020610351,-0.68983547500961,4.85482374613937));
#12995=CARTESIAN_POINT('Ctrl Pts',(5.89351974274144,2.42538824376421,4.99376822274656));
#12996=CARTESIAN_POINT('Ctrl Pts',(4.01487686851768,4.94942893894988,5.13271269935375));
#12997=CARTESIAN_POINT('Ctrl Pts',(1.15761663166472,6.26705726997656,5.27165717596093));
#12998=CARTESIAN_POINT('Ctrl Pts',(-1.98181010047945,6.05710424350701,5.41060165256812));
#12999=CARTESIAN_POINT('Ctrl Pts',(-4.63817500102154,4.3707454456845,5.54954612917531));
#13000=CARTESIAN_POINT('Ctrl Pts',(-6.16399499681084,1.6190271061238,5.68849060578249));
#13001=CARTESIAN_POINT('Ctrl Pts',(-6.18735483638979,-1.52732551202311,
5.82743508238968));
#13002=CARTESIAN_POINT('Ctrl Pts',(-4.70256061049319,-4.30139591245804,
5.96637955899686));
#13003=CARTESIAN_POINT('Ctrl Pts',(-2.07152762984648,-6.02701056659564,
6.10532403560405));
#13004=CARTESIAN_POINT('Ctrl Pts',(1.06443563188314,-6.28355471661148,6.24426851221124));
#13005=CARTESIAN_POINT('Ctrl Pts',(3.94094506106056,-5.00849629297808,6.38321298881842));
#13006=CARTESIAN_POINT('Ctrl Pts',(5.8568578422652,-2.51262796819774,6.52215746542561));
#13007=CARTESIAN_POINT('Ctrl Pts',(6.34517446981551,0.595687870175684,6.6611019420328));
#13008=CARTESIAN_POINT('Ctrl Pts',(5.28686884507105,3.55880610684117,6.80004641863999));
#13009=CARTESIAN_POINT('Ctrl Pts',(2.93990062489312,5.65447322098407,6.93899089524718));
#13010=CARTESIAN_POINT('Ctrl Pts',(-0.123661874547718,6.37187498557969,
7.07793537185436));
#13011=CARTESIAN_POINT('Ctrl Pts',(-3.15708206539707,5.53614630617914,7.21687984846155));
#13012=CARTESIAN_POINT('Ctrl Pts',(-5.42097048089627,3.35099420117735,7.35582432506874));
#13013=CARTESIAN_POINT('Ctrl Pts',(-6.36350932363407,0.349044666332412,
7.49476880167592));
#13014=CARTESIAN_POINT('Ctrl Pts',(-5.75495683398433,-2.73798373443851,
7.63371327828311));
#13015=CARTESIAN_POINT('Ctrl Pts',(-3.74364633621719,-5.15763465169844,
7.7726577548903));
#13016=CARTESIAN_POINT('Ctrl Pts',(-0.819830318568966,-6.32012352251346,
7.91160223149748));
#13017=CARTESIAN_POINT('Ctrl Pts',(2.3038175271616,-5.94209625406859,8.05054670810467));
#13018=CARTESIAN_POINT('Ctrl Pts',(4.86591494276851,-4.11569615749451,8.18949118471185));
#13019=CARTESIAN_POINT('Ctrl Pts',(6.24195634619481,-1.28610421944378,8.32843566131905));
#13020=CARTESIAN_POINT('Ctrl Pts',(6.09653468681619,1.85697277942353,8.46738013792624));
#13021=CARTESIAN_POINT('Ctrl Pts',(4.46509617268103,4.54741676776849,8.60632461453341));
#13022=CARTESIAN_POINT('Ctrl Pts',(1.74530033564544,6.12943797011348,8.74526909114061));
#13023=CARTESIAN_POINT('Ctrl Pts',(-1.39990860057091,6.21742221512424,8.88421356774779));
#13024=CARTESIAN_POINT('Ctrl Pts',(-4.20389290961247,4.78992353755077,9.02315804435498));
#13025=CARTESIAN_POINT('Ctrl Pts',(-5.98318761378964,2.19489158485495,9.16210252096216));
#13026=CARTESIAN_POINT('Ctrl Pts',(-6.30409356172975,-0.935140340286029,
9.30104699756935));
#13027=CARTESIAN_POINT('Ctrl Pts',(-5.08839063792002,-3.83723387442058,
9.43999147417654));
#13028=CARTESIAN_POINT('Ctrl Pts',(-2.63240374297399,-5.80401013309328,
9.57893595078373));
#13029=CARTESIAN_POINT('Ctrl Pts',(0.465225745926736,-6.35607175041312,
9.71788042739091));
#13030=CARTESIAN_POINT('Ctrl Pts',(3.44945748754508,-5.3588549273788,9.8568249039981));
#13031=CARTESIAN_POINT('Ctrl Pts',(5.59289159090131,-3.05542906045914,9.99576938060529));
#13032=CARTESIAN_POINT('Ctrl Pts',(6.37307073092924,-0.00724911345954777,
10.1347138572125));
#13033=CARTESIAN_POINT('Ctrl Pts',(5.59982796667497,3.04269778892314,10.2736583338197));
#13034=CARTESIAN_POINT('Ctrl Pts',(3.46163951282899,5.35099383052288,10.4126028104269));
#13035=CARTESIAN_POINT('Ctrl Pts',(0.479684078983856,6.35499695322053,10.551547287034));
#13036=CARTESIAN_POINT('Ctrl Pts',(-2.6191932888691,5.80998361500408,10.6904917636412));
#13037=CARTESIAN_POINT('Ctrl Pts',(-5.07964808175639,3.84879961242222,10.8294362402485));
#13038=CARTESIAN_POINT('Ctrl Pts',(-6.30194988224866,0.949479211304296,
10.9683807168555));
#13039=CARTESIAN_POINT('Ctrl Pts',(-5.98816532812638,-2.18127464893759,
11.1073251934627));
#13040=CARTESIAN_POINT('Ctrl Pts',(-4.21477871089973,-4.78034763476667,
11.2462696700699));
#13041=CARTESIAN_POINT('Ctrl Pts',(-1.41404909880579,-6.21422145061144,
11.3852141466772));
#13042=CARTESIAN_POINT('Ctrl Pts',(1.73135185565299,-6.13339252314735,11.5241586232844));
#13043=CARTESIAN_POINT('Ctrl Pts',(4.4547396220989,-4.55756272478778,11.6631030998916));
#13044=CARTESIAN_POINT('Ctrl Pts',(6.0922944519577,-1.87083708583035,11.8020475764987));
#13045=CARTESIAN_POINT('Ctrl Pts',(6.24486597493456,1.27190095769183,11.9409920531059));
#13046=CARTESIAN_POINT('Ctrl Pts',(4.87526521953232,4.10461595405606,12.0799365297131));
#13047=CARTESIAN_POINT('Ctrl Pts',(2.31732934265519,5.93683988404119,12.2188810063202));
#13048=CARTESIAN_POINT('Ctrl Pts',(-0.80545043950706,6.32197221447316,12.3578254829274));
#13049=CARTESIAN_POINT('Ctrl Pts',(-3.73190345732448,5.16613779106621,12.4967699595346));
#13050=CARTESIAN_POINT('Ctrl Pts',(-5.74871325603565,2.75106869978792,12.6357144361419));
#13051=CARTESIAN_POINT('Ctrl Pts',(-6.36428690495424,-0.334567306383601,
12.774658912749));
#13052=CARTESIAN_POINT('Ctrl Pts',(-5.4285796877572,-3.33865327111739,12.9136033893563));
#13053=CARTESIAN_POINT('Ctrl Pts',(-3.16966817044503,-5.52894988043305,
13.0525478659634));
#13054=CARTESIAN_POINT('Ctrl Pts',(-0.138157042496288,-6.37157717701681,
13.1914923425705));
#13055=CARTESIAN_POINT('Ctrl Pts',(2.92702955919275,-5.66114661978338,13.3304368191777));
#13056=CARTESIAN_POINT('Ctrl Pts',(5.2787591754345,-3.57082408679553,13.469381295785));
#13057=CARTESIAN_POINT('Ctrl Pts',(6.34380291029186,-0.610121075234528,
13.6083257723922));
#13058=CARTESIAN_POINT('Ctrl Pts',(5.86255870745683,2.49929759986584,13.7472702489993));
#13059=CARTESIAN_POINT('Ctrl Pts',(3.95232877767757,4.99951800918994,13.8862147256066));
#13060=CARTESIAN_POINT('Ctrl Pts',(1.07872744416156,6.28111695419576,14.0251592022138));
#13061=CARTESIAN_POINT('Ctrl Pts',(-2.05781131956035,6.03170752475302,14.1641036788208));
#13062=CARTESIAN_POINT('Ctrl Pts',(-4.6927631225145,4.31208271801931,14.303048155428));
#13063=CARTESIAN_POINT('Ctrl Pts',(-6.18386428675798,1.54139727975371,14.4419926320353));
#13064=CARTESIAN_POINT('Ctrl Pts',(-6.16766219928348,-1.6050003385054,14.5809371086424));
#13065=CARTESIAN_POINT('Ctrl Pts',(-4.64810608310154,-4.36018267178192,
14.7198815852497));
#13066=CARTESIAN_POINT('Ctrl Pts',(-1.99558438286049,-6.05258011611217,
14.8588260618568));
#13067=CARTESIAN_POINT('Ctrl Pts',(1.14335659986781,-6.26967453514227,14.997770538464));
#13068=CARTESIAN_POINT('Ctrl Pts',(4.00360693853646,-4.95854964407699,15.1367150150712));
#13069=CARTESIAN_POINT('Ctrl Pts',(5.88798693509895,-2.43878923713729,15.2756594916783));
#13070=CARTESIAN_POINT('Ctrl Pts',(6.3371831304334,0.675420655904715,15.4146039682855));
#13071=CARTESIAN_POINT('Ctrl Pts',(5.24170494478436,3.62499825695112,15.5535484448927));
#13072=CARTESIAN_POINT('Ctrl Pts',(2.86857276457088,5.69099054518877,15.6924929214999));
#13073=CARTESIAN_POINT('Ctrl Pts',(-0.203767686607458,6.36981646682085,
15.8314373981072));
#13074=CARTESIAN_POINT('Ctrl Pts',(-3.22644021456298,5.49601370384942,15.9703818747144));
#13075=CARTESIAN_POINT('Ctrl Pts',(-5.46267507161012,3.28256974839915,16.1093263513215));
#13076=CARTESIAN_POINT('Ctrl Pts',(-6.36739495409124,0.269006672213413,
16.2482708279286));
#13077=CARTESIAN_POINT('Ctrl Pts',(-5.72007639034474,-2.81012618570307,
16.3872153045359));
#13078=CARTESIAN_POINT('Ctrl Pts',(-3.67850184953075,-5.2042969971408,16.526159781143));
#13079=CARTESIAN_POINT('Ctrl Pts',(-0.740300613459242,-6.32993191842897,
16.6651042577503));
#13080=CARTESIAN_POINT('Ctrl Pts',(2.37834726082389,-5.91265992590842,16.8040487343575));
#13081=CARTESIAN_POINT('Ctrl Pts',(4.91727824720379,-4.05419014464293,16.9429932109646));
#13082=CARTESIAN_POINT('Ctrl Pts',(6.25763352934226,-1.20752047764986,17.0819376875718));
#13083=CARTESIAN_POINT('Ctrl Pts',(6.07270447019572,1.93347963887718,17.220882164179));
#13084=CARTESIAN_POINT('Ctrl Pts',(4.40756711841003,4.60319836289913,17.3598266407861));
#13085=CARTESIAN_POINT('Ctrl Pts',(1.66809502455076,6.15089766843531,17.4987711173933));
#13086=CARTESIAN_POINT('Ctrl Pts',(-1.477971546528,6.1993292468395,17.6377155940006));
#13087=CARTESIAN_POINT('Ctrl Pts',(-4.2637858160287,4.73668805462234,17.7766600706078));
#13088=CARTESIAN_POINT('Ctrl Pts',(-6.0103117246986,2.11948955787736,17.915604547215));
#13089=CARTESIAN_POINT('Ctrl Pts',(-6.29183742015302,-1.014329714779,18.0545490238221));
#13090=CARTESIAN_POINT('Ctrl Pts',(-5.03974168050939,-3.90090859517803,
18.1934935004293));
#13091=CARTESIAN_POINT('Ctrl Pts',(-2.55921998820667,-5.83664916897836,
18.3324379770364));
#13092=CARTESIAN_POINT('Ctrl Pts',(0.545105807019446,-6.34972030867309,
18.4713824536436));
#13093=CARTESIAN_POINT('Ctrl Pts',(3.51656348751869,-5.31505939160815,18.6103269302508));
#13094=CARTESIAN_POINT('Ctrl Pts',(5.63086615713259,-2.98486796173379,18.749271406858));
#13095=CARTESIAN_POINT('Ctrl Pts',(6.37265849741127,0.072885237843671,18.8882158834652));
#13096=CARTESIAN_POINT('Ctrl Pts',(5.56112774530412,3.11285947508733,19.0271603600725));
#13097=CARTESIAN_POINT('Ctrl Pts',(3.39408767243104,5.39410728635009,19.1661048366796));
#13098=CARTESIAN_POINT('Ctrl Pts',(0.399739803186753,6.36050197249609,19.3050493132868));
#13099=CARTESIAN_POINT('Ctrl Pts',(-2.69203113704428,5.77663924033402,19.4439937898939));
#13100=CARTESIAN_POINT('Ctrl Pts',(-5.12765029985884,3.78453526026606,19.5829382665011));
#13101=CARTESIAN_POINT('Ctrl Pts',(-6.3133662230816,0.870350812755841,19.7218827431083));
#13102=CARTESIAN_POINT('Ctrl Pts',(-5.96032210201671,-2.25677804382996,
19.8608272197155));
#13103=CARTESIAN_POINT('Ctrl Pts',(-4.75618023071243,-3.97353026262882,
19.9534568707871));
#13104=CARTESIAN_POINT('Ctrl Pts',(-3.98522955105091,-4.63622755188139,
19.9997716963227));
#13105=CARTESIAN_POINT('',(-2.03522692205371,4.71657388088067,20.0001232957739));
#13106=CARTESIAN_POINT('Ctrl Pts',(-3.98497178445977,-4.63592767842204,
20.));
#13107=CARTESIAN_POINT('Ctrl Pts',(-4.10345142310591,-4.51664357863181,
20.));
#13108=CARTESIAN_POINT('Ctrl Pts',(-4.21664327579648,-4.39262753031591,
20.));
#13109=CARTESIAN_POINT('Ctrl Pts',(-4.32436939900696,-4.2642850247564,20.));
#13110=CARTESIAN_POINT('Ctrl Pts',(-4.43329818051566,-4.13450969886763,
20.));
#13111=CARTESIAN_POINT('Ctrl Pts',(-4.53663891101179,-4.00031013114139,
20.));
#13112=CARTESIAN_POINT('Ctrl Pts',(-4.63416502605001,-3.86207416964644,
20.));
#13113=CARTESIAN_POINT('Ctrl Pts',(-4.73137732966119,-3.72428301233883,
20.));
#13114=CARTESIAN_POINT('Ctrl Pts',(-4.82281267416501,-3.58248070026889,
20.));
#13115=CARTESIAN_POINT('Ctrl Pts',(-4.90819951386566,-3.43703052021648,
20.));
#13116=CARTESIAN_POINT('Ctrl Pts',(-4.99221969940335,-3.29390833467434,
20.));
#13117=CARTESIAN_POINT('Ctrl Pts',(-5.07038362157542,-3.14725345974558,
20.));
#13118=CARTESIAN_POINT('Ctrl Pts',(-5.14238351610632,-2.99740187421602,
20.));
#13119=CARTESIAN_POINT('Ctrl Pts',(-5.17779799209172,-2.92369460823058,
20.));
#13120=CARTESIAN_POINT('Ctrl Pts',(-5.21172040481118,-2.84921385219213,
20.));
#13121=CARTESIAN_POINT('Ctrl Pts',(-5.24410947080105,-2.77399939051084,
20.));
#13122=CARTESIAN_POINT('Ctrl Pts',(-5.25356655628965,-2.75203797938769,
20.));
#13123=CARTESIAN_POINT('Ctrl Pts',(-5.26289289622801,-2.73001401712101,
20.));
#13124=CARTESIAN_POINT('Ctrl Pts',(-5.27208741122818,-2.70792849662542,
20.));
#13125=CARTESIAN_POINT('Ctrl Pts',(-5.28025870056582,-2.68830079705255,
20.));
#13126=CARTESIAN_POINT('Ctrl Pts',(-5.28832272962313,-2.6686319848304,20.));
#13127=CARTESIAN_POINT('Ctrl Pts',(-5.29627731007746,-2.64892710108863,
20.));
#13128=CARTESIAN_POINT('Ctrl Pts',(-5.35809518452346,-2.49579343978298,
20.));
#13129=CARTESIAN_POINT('Ctrl Pts',(-5.41334140189166,-2.34040024681067,
20.));
#13130=CARTESIAN_POINT('Ctrl Pts',(-5.46179567772308,-2.18310192386359,
20.));
#13131=CARTESIAN_POINT('Ctrl Pts',(-5.47241361317542,-2.14863265544187,
20.));
#13132=CARTESIAN_POINT('Ctrl Pts',(-5.48270521458296,-2.11407184571832,
20.));
#13133=CARTESIAN_POINT('Ctrl Pts',(-5.49266783943823,-2.07942313795932,
20.));
#13134=CARTESIAN_POINT('Ctrl Pts',(-5.53831342921429,-1.92067373972215,
20.));
#13135=CARTESIAN_POINT('Ctrl Pts',(-5.57705736058314,-1.76007949695175,
20.));
#13136=CARTESIAN_POINT('Ctrl Pts',(-5.60888551437011,-1.59809685908707,
20.));
#13137=CARTESIAN_POINT('Ctrl Pts',(-5.64065619906291,-1.43640669798783,
20.));
#13138=CARTESIAN_POINT('Ctrl Pts',(-5.66553599618983,-1.2733323692898,20.));
#13139=CARTESIAN_POINT('Ctrl Pts',(-5.68345920600138,-1.10933093107998,
20.));
#13140=CARTESIAN_POINT('Ctrl Pts',(-5.70113221551854,-0.947618882357451,
20.));
#13141=CARTESIAN_POINT('Ctrl Pts',(-5.71204135337902,-0.785004725997997,
20.));
#13142=CARTESIAN_POINT('Ctrl Pts',(-5.71607509551897,-0.621940605475564,
20.));
#13143=CARTESIAN_POINT('Ctrl Pts',(-5.71706208119408,-0.582041686432943,
20.));
#13144=CARTESIAN_POINT('Ctrl Pts',(-5.71763721586455,-0.54211592222943,
20.));
#13145=CARTESIAN_POINT('Ctrl Pts',(-5.71779842995933,-0.502170139060898,
20.));
#13146=CARTESIAN_POINT('Ctrl Pts',(-5.71788229794433,-0.481389249226882,
20.));
#13147=CARTESIAN_POINT('Ctrl Pts',(-5.71785409277925,-0.460611220002977,
20.));
#13148=CARTESIAN_POINT('Ctrl Pts',(-5.71771384536836,-0.439841148815751,
20.));
#13149=CARTESIAN_POINT('Ctrl Pts',(-5.71662256856856,-0.278227492825956,
20.));
#13150=CARTESIAN_POINT('Ctrl Pts',(-5.70875229303737,-0.117013828842298,
20.));
#13151=CARTESIAN_POINT('Ctrl Pts',(-5.69409684800798,0.0433725228550221,
20.));
#13152=CARTESIAN_POINT('Ctrl Pts',(-5.67956337329034,0.202424055085909,
20.));
#13153=CARTESIAN_POINT('Ctrl Pts',(-5.65835705764461,0.36066270542086,20.));
#13154=CARTESIAN_POINT('Ctrl Pts',(-5.63042198125465,0.517661960780568,
20.));
#13155=CARTESIAN_POINT('Ctrl Pts',(-5.61544285829542,0.601846844248007,
20.));
#13156=CARTESIAN_POINT('Ctrl Pts',(-5.59852821807851,0.685675140861376,
20.));
#13157=CARTESIAN_POINT('Ctrl Pts',(-5.57966365650049,0.769078844724802,
20.));
#13158=CARTESIAN_POINT('Ctrl Pts',(-5.54429238610119,0.925461750813273,
20.));
#13159=CARTESIAN_POINT('Ctrl Pts',(-5.50206814309807,1.08035384648384,20.));
#13160=CARTESIAN_POINT('Ctrl Pts',(-5.45314714973918,1.23332826719705,20.));
#13161=CARTESIAN_POINT('Ctrl Pts',(-5.41289015274892,1.35921064143795,20.));
#13162=CARTESIAN_POINT('Ctrl Pts',(-5.36809746764452,1.48379413599428,20.));
#13163=CARTESIAN_POINT('Ctrl Pts',(-5.31883665527128,1.60682291183031,20.));
#13164=CARTESIAN_POINT('Ctrl Pts',(-5.30921006803183,1.63086529331958,20.));
#13165=CARTESIAN_POINT('Ctrl Pts',(-5.29941130945311,1.65485162666062,20.));
#13166=CARTESIAN_POINT('Ctrl Pts',(-5.28945123030884,1.678755478121,20.));
#13167=CARTESIAN_POINT('Ctrl Pts',(-5.22881157867328,1.824288581253,20.));
#13168=CARTESIAN_POINT('Ctrl Pts',(-5.16212791782585,1.96694176941535,20.));
#13169=CARTESIAN_POINT('Ctrl Pts',(-5.08961453505449,2.10634429686568,20.));
#13170=CARTESIAN_POINT('Ctrl Pts',(-5.01729884220903,2.24536677756778,20.));
#13171=CARTESIAN_POINT('Ctrl Pts',(-4.93918471648935,2.38115692318346,20.));
#13172=CARTESIAN_POINT('Ctrl Pts',(-4.8554417170334,2.51331841980725,20.));
#13173=CARTESIAN_POINT('Ctrl Pts',(-4.77314573387395,2.64319626477504,20.));
#13174=CARTESIAN_POINT('Ctrl Pts',(-4.68541322918649,2.76957026126409,20.));
#13175=CARTESIAN_POINT('Ctrl Pts',(-4.59237070154098,2.89202857031072,20.));
#13176=CARTESIAN_POINT('Ctrl Pts',(-4.51158814582467,2.99835086640283,20.));
#13177=CARTESIAN_POINT('Ctrl Pts',(-4.4268020750054,3.10172108215086,20.));
#13178=CARTESIAN_POINT('Ctrl Pts',(-4.33807775610302,3.20184297416315,20.));
#13179=CARTESIAN_POINT('Ctrl Pts',(-4.30162703065241,3.24297617915682,20.));
#13180=CARTESIAN_POINT('Ctrl Pts',(-4.26451141446763,3.28356080052371,20.));
#13181=CARTESIAN_POINT('Ctrl Pts',(-4.22674502571624,3.32358241695396,20.));
#13182=CARTESIAN_POINT('Ctrl Pts',(-4.20574577986708,3.34583563709189,20.));
#13183=CARTESIAN_POINT('Ctrl Pts',(-4.18454533067273,3.36791477988588,20.));
#13184=CARTESIAN_POINT('Ctrl Pts',(-4.16314607616287,3.38981726275068,20.));
#13185=CARTESIAN_POINT('Ctrl Pts',(-4.14604768953812,3.40731773782059,20.));
#13186=CARTESIAN_POINT('Ctrl Pts',(-4.12882477256853,3.42470289052077,20.));
#13187=CARTESIAN_POINT('Ctrl Pts',(-4.11148805803735,3.44196235396036,20.));
#13188=CARTESIAN_POINT('Ctrl Pts',(-4.00202352440943,3.55093912188743,20.));
#13189=CARTESIAN_POINT('Ctrl Pts',(-3.88791934040221,3.65501678237065,20.));
#13190=CARTESIAN_POINT('Ctrl Pts',(-3.76954171862907,3.75394242380618,20.));
#13191=CARTESIAN_POINT('Ctrl Pts',(-3.66605495616142,3.8404240932624,20.));
#13192=CARTESIAN_POINT('Ctrl Pts',(-3.55930146424434,3.92296791358125,20.));
#13193=CARTESIAN_POINT('Ctrl Pts',(-3.44951147850304,4.00137564676462,20.));
#13194=CARTESIAN_POINT('Ctrl Pts',(-3.39461648563239,4.04057951335631,20.));
#13195=CARTESIAN_POINT('Ctrl Pts',(-3.33896219659931,4.0787489115657,20.));
#13196=CARTESIAN_POINT('Ctrl Pts',(-3.28257658007889,4.11585626044096,20.));
#13197=CARTESIAN_POINT('Ctrl Pts',(-3.24675220416138,4.13943226612191,20.));
#13198=CARTESIAN_POINT('Ctrl Pts',(-3.21063260796433,4.16257952185971,20.));
#13199=CARTESIAN_POINT('Ctrl Pts',(-3.17422489271026,4.18529053994777,20.));
#13200=CARTESIAN_POINT('Ctrl Pts',(-3.15332884709973,4.19832542737528,20.));
#13201=CARTESIAN_POINT('Ctrl Pts',(-3.13234039284392,4.21121498778926,20.));
#13202=CARTESIAN_POINT('Ctrl Pts',(-3.1112699212428,4.22395259948423,20.));
#13203=CARTESIAN_POINT('Ctrl Pts',(-2.98179244193094,4.30222487957077,20.));
#13204=CARTESIAN_POINT('Ctrl Pts',(-2.84912244425002,4.37482416604639,20.));
#13205=CARTESIAN_POINT('Ctrl Pts',(-2.71359482646064,4.44147979884137,20.));
#13206=CARTESIAN_POINT('Ctrl Pts',(-2.58015601234134,4.50710810943671,20.));
#13207=CARTESIAN_POINT('Ctrl Pts',(-2.44394632034707,4.56697476102533,20.));
#13208=CARTESIAN_POINT('Ctrl Pts',(-2.3052748294092,4.62077220858218,20.));
#13209=CARTESIAN_POINT('Ctrl Pts',(-2.2623645775541,4.6374191920985,20.));
#13210=CARTESIAN_POINT('Ctrl Pts',(-2.21921856473085,4.6534846662791,20.));
#13211=CARTESIAN_POINT('Ctrl Pts',(-2.17584588854955,4.66895849845131,20.));
#13212=CARTESIAN_POINT('Ctrl Pts',(-2.12925963268156,4.68557882185077,20.));
#13213=CARTESIAN_POINT('Ctrl Pts',(-2.08241187520335,4.70151658422014,20.));
#13214=CARTESIAN_POINT('Ctrl Pts',(-2.03531819920643,4.71676781801449,20.));
#13215=CARTESIAN_POINT('Ctrl Pts',(3.87994761181449,-3.36633437021265,-1.66506348639461E-15));
#13216=CARTESIAN_POINT('Ctrl Pts',(3.98625412824271,-3.26478406208168,-3.99257968720234E-15));
#13217=CARTESIAN_POINT('Ctrl Pts',(4.08787833026421,-3.15878135837575,-4.66065732929026E-15));
#13218=CARTESIAN_POINT('Ctrl Pts',(4.18469942561242,-3.04876049740387,-3.16066617322974E-15));
#13219=CARTESIAN_POINT('Ctrl Pts',(4.28403790290049,-2.93587905602415,-1.62167472872341E-15));
#13220=CARTESIAN_POINT('Ctrl Pts',(4.37832079024333,-2.8187674593301,-5.82952701121535E-16));
#13221=CARTESIAN_POINT('Ctrl Pts',(4.46739427387372,-2.69784518274753,-1.11716191852906E-15));
#13222=CARTESIAN_POINT('Ctrl Pts',(4.55725996217229,-2.57584744365813,-1.65612230338365E-15));
#13223=CARTESIAN_POINT('Ctrl Pts',(4.64182368695275,-2.4499704170692,-3.02543370549841E-15));
#13224=CARTESIAN_POINT('Ctrl Pts',(4.72089616098145,-2.32060185485371,-4.26048085699904E-15));
#13225=CARTESIAN_POINT('Ctrl Pts',(4.80003857099738,-2.19111887206108,-5.49662035122531E-15));
#13226=CARTESIAN_POINT('Ctrl Pts',(4.87368051051603,-2.05813757511725,-3.42002525595283E-15));
#13227=CARTESIAN_POINT('Ctrl Pts',(4.94159337332724,-1.92201238315165,-2.17881268582687E-15));
#13228=CARTESIAN_POINT('Ctrl Pts',(4.9612628949575,-1.88258660581057,-1.819321766357E-15));
#13229=CARTESIAN_POINT('Ctrl Pts',(4.98045155883349,-1.84289691540223,-3.90912234781053E-15));
#13230=CARTESIAN_POINT('Ctrl Pts',(4.99915311004593,-1.8029514969195,-3.83026943495679E-15));
#13231=CARTESIAN_POINT('Ctrl Pts',(5.0122478283282,-1.77498194531617,-3.86522662205903E-15));
#13232=CARTESIAN_POINT('Ctrl Pts',(5.02510451482084,-1.74688523424048,-6.32070288793251E-15));
#13233=CARTESIAN_POINT('Ctrl Pts',(5.03771836274217,-1.71866987256631,-5.49560397189452E-15));
#13234=CARTESIAN_POINT('Ctrl Pts',(5.04744161877782,-1.69692034875664,-4.85958488672596E-15));
#13235=CARTESIAN_POINT('Ctrl Pts',(5.05701729403857,-1.67510763703549,-4.39002047913497E-15));
#13236=CARTESIAN_POINT('Ctrl Pts',(5.0664416202758,-1.65324062354264,-3.95516952522712E-15));
#13237=CARTESIAN_POINT('Ctrl Pts',(5.12809970670852,-1.5101770056215,-1.11018336637909E-15));
#13238=CARTESIAN_POINT('Ctrl Pts',(5.18333108174967,-1.36468296185368,-3.57813607222297E-15));
#13239=CARTESIAN_POINT('Ctrl Pts',(5.23197030770333,-1.21718642306848,-4.52415882534751E-15));
#13240=CARTESIAN_POINT('Ctrl Pts',(5.23918133000613,-1.19531928168388,-4.66441169816742E-15));
#13241=CARTESIAN_POINT('Ctrl Pts',(5.24624739671494,-1.17340805699876,-4.80562514306417E-15));
#13242=CARTESIAN_POINT('Ctrl Pts',(5.25316790132191,-1.15145407394423,-4.71844785465692E-15));
#13243=CARTESIAN_POINT('Ctrl Pts',(5.2993807558818,-1.0048525927621,-3.31652852302662E-15));
#13244=CARTESIAN_POINT('Ctrl Pts',(5.33910647450617,-0.85634686171711,-4.64282921799142E-15));
#13245=CARTESIAN_POINT('Ctrl Pts',(5.37241286996191,-0.70637980290893,-3.24740234702858E-15));
#13246=CARTESIAN_POINT('Ctrl Pts',(5.40605735852673,-0.554890428987424,
-1.83781050255697E-15));
#13247=CARTESIAN_POINT('Ctrl Pts',(5.433151739794,-0.40190923262953,-4.04102800082177E-15));
#13248=CARTESIAN_POINT('Ctrl Pts',(5.45371837894091,-0.247868617103554,
-3.7470027081099E-15));
#13249=CARTESIAN_POINT('Ctrl Pts',(5.47436154606792,-0.0932548200734815,
-3.45188335420551E-15));
#13250=CARTESIAN_POINT('Ctrl Pts',(5.48842846893721,0.0624270392375904,
-4.61732734771393E-15));
#13251=CARTESIAN_POINT('Ctrl Pts',(5.49589140153741,0.218753153023537,-2.94209101525666E-15));
#13252=CARTESIAN_POINT('Ctrl Pts',(5.49724004581173,0.247003216313493,-2.63935507900513E-15));
#13253=CARTESIAN_POINT('Ctrl Pts',(5.49837288778739,0.275274336924491,-2.06251622087461E-15));
#13254=CARTESIAN_POINT('Ctrl Pts',(5.49928958238686,0.303564030594172,-1.08246744900953E-15));
#13255=CARTESIAN_POINT('Ctrl Pts',(5.49992470520323,0.323164265970328,-1.07591380186277E-15));
#13256=CARTESIAN_POINT('Ctrl Pts',(5.50045595765575,0.342771173576785,-2.10354853696197E-15));
#13257=CARTESIAN_POINT('Ctrl Pts',(5.50088315437835,0.362372657450585,-2.38697950294409E-15));
#13258=CARTESIAN_POINT('Ctrl Pts',(5.50434740873726,0.521326418934704,-4.20068571385626E-15));
#13259=CARTESIAN_POINT('Ctrl Pts',(5.50097990316086,0.680128718969271,-5.0287057528373E-15));
#13260=CARTESIAN_POINT('Ctrl Pts',(5.49085897729658,0.83831694807423,-4.49640324973188E-15));
#13261=CARTESIAN_POINT('Ctrl Pts',(5.48062459361156,0.998278502266276,-5.58026560193877E-15));
#13262=CARTESIAN_POINT('Ctrl Pts',(5.46348472039185,1.15761287955169,-3.85240679458042E-15));
#13263=CARTESIAN_POINT('Ctrl Pts',(5.43947063245582,1.31586030999698,-3.60822483003176E-15));
#13264=CARTESIAN_POINT('Ctrl Pts',(5.42659218943676,1.40072634868776,-3.51003661510938E-15));
#13265=CARTESIAN_POINT('Ctrl Pts',(5.41173583367755,1.48528002633643,-6.25273444309056E-15));
#13266=CARTESIAN_POINT('Ctrl Pts',(5.39490030124413,1.56945143909657,-5.93969318174459E-15));
#13267=CARTESIAN_POINT('Ctrl Pts',(5.36361962345765,1.72584321653484,-5.17779511488788E-15));
#13268=CARTESIAN_POINT('Ctrl Pts',(5.32550956672002,1.88091577537441,-5.32303990139189E-15));
#13269=CARTESIAN_POINT('Ctrl Pts',(5.28079475052835,2.0343024122608,-6.21724893790088E-15));
#13270=CARTESIAN_POINT('Ctrl Pts',(5.24056853374701,2.17229166576248,-7.02169474835133E-15));
#13271=CARTESIAN_POINT('Ctrl Pts',(5.19499619626958,2.30891683667062,-8.73640693159127E-15));
#13272=CARTESIAN_POINT('Ctrl Pts',(5.14420597728033,2.44390372836124,-6.38378239159465E-15));
#13273=CARTESIAN_POINT('Ctrl Pts',(5.13676783596577,2.46367232940273,-5.89581381797849E-15));
#13274=CARTESIAN_POINT('Ctrl Pts',(5.12922090618192,2.48339729434992,-7.37503164949818E-15));
#13275=CARTESIAN_POINT('Ctrl Pts',(5.12156722405834,2.50307433977403,-7.16093850883226E-15));
#13276=CARTESIAN_POINT('Ctrl Pts',(5.06254373198642,2.65481933203217,-5.82228573301255E-15));
#13277=CARTESIAN_POINT('Ctrl Pts',(4.99715084449456,2.80378105414597,-6.86084642416168E-15));
#13278=CARTESIAN_POINT('Ctrl Pts',(4.92569221311423,2.94959170115283,-5.93969318174459E-15));
#13279=CARTESIAN_POINT('Ctrl Pts',(4.85355670772662,3.09678350303263,-4.90588385216813E-15));
#13280=CARTESIAN_POINT('Ctrl Pts',(4.77523981660915,3.24076495388049,-2.82624632148367E-15));
#13281=CARTESIAN_POINT('Ctrl Pts',(4.69100020769895,3.38115471434809,-3.1641356201817E-15));
#13282=CARTESIAN_POINT('Ctrl Pts',(4.60668102574095,3.52167708750544,-3.16778207269044E-15));
#13283=CARTESIAN_POINT('Ctrl Pts',(4.51642766943348,3.6586017037791,-3.45017579044051E-15));
#13284=CARTESIAN_POINT('Ctrl Pts',(4.42044948051561,3.79153244523825,-1.72084568816899E-15));
#13285=CARTESIAN_POINT('Ctrl Pts',(4.3370333504216,3.90706461091121,-6.97009822649519E-16));
#13286=CARTESIAN_POINT('Ctrl Pts',(4.24929202402402,4.01958003898395,9.76388561238391E-16));
#13287=CARTESIAN_POINT('Ctrl Pts',(4.15733458420634,4.12880382702963,2.05391259555654E-15));
#13288=CARTESIAN_POINT('Ctrl Pts',(4.11146289933332,4.18328858863024,3.36724768757498E-15));
#13289=CARTESIAN_POINT('Ctrl Pts',(4.0645416851672,4.2369540081248,9.48537125816697E-16));
#13290=CARTESIAN_POINT('Ctrl Pts',(4.01659887073521,4.2897806305052,1.83186799063151E-15));
#13291=CARTESIAN_POINT('Ctrl Pts',(3.99710940469441,4.31125543700396,2.19095510507315E-15));
#13292=CARTESIAN_POINT('Ctrl Pts',(3.97744901168162,4.33259382998145,4.96890495175676E-15));
#13293=CARTESIAN_POINT('Ctrl Pts',(3.95762725058284,4.35378620795006,3.83026943495679E-15));
#13294=CARTESIAN_POINT('Ctrl Pts',(3.93076602539778,4.38250480838041,2.2872609773302E-15));
#13295=CARTESIAN_POINT('Ctrl Pts',(3.90361969409604,4.41094340467956,2.65613658226391E-15));
#13296=CARTESIAN_POINT('Ctrl Pts',(3.87619542506123,4.43909844700456,2.05391259555654E-15));
#13297=CARTESIAN_POINT('Ctrl Pts',(3.7605238672531,4.5578522997236,-4.86180145054305E-16));
#13298=CARTESIAN_POINT('Ctrl Pts',(3.63990082270005,4.67157471441651,6.00296082402392E-16));
#13299=CARTESIAN_POINT('Ctrl Pts',(3.51475018610364,4.78007264497113,1.94289029309402E-15));
#13300=CARTESIAN_POINT('Ctrl Pts',(3.38799964511639,4.88995759456307,3.30264799916393E-15));
#13301=CARTESIAN_POINT('Ctrl Pts',(3.25660455332876,4.99448417190688,4.82424686146942E-16));
#13302=CARTESIAN_POINT('Ctrl Pts',(3.12096094677142,5.09342213195151,4.10782519111308E-15));
#13303=CARTESIAN_POINT('Ctrl Pts',(3.0422347841794,5.15084471254106,6.21197058254715E-15));
#13304=CARTESIAN_POINT('Ctrl Pts',(2.96207671226679,5.20638416123899,4.7199000144875E-15));
#13305=CARTESIAN_POINT('Ctrl Pts',(2.88055840535682,5.25998984590168,5.16253706450698E-15));
#13306=CARTESIAN_POINT('Ctrl Pts',(2.81549585559289,5.30277437686413,5.32754643687697E-15));
#13307=CARTESIAN_POINT('Ctrl Pts',(2.7496398810422,5.34427876513908,2.86135815288528E-15));
#13308=CARTESIAN_POINT('Ctrl Pts',(2.68303739503652,5.38448001903572,3.44169137633799E-15));
#13309=CARTESIAN_POINT('Ctrl Pts',(2.53350644115478,5.47473688785431,4.7446124184256E-15));
#13310=CARTESIAN_POINT('Ctrl Pts',(2.38020694554204,5.55843341882744,6.34977018440613E-15));
#13311=CARTESIAN_POINT('Ctrl Pts',(2.22358026859405,5.63532026171932,7.21644966006352E-15));
#13312=CARTESIAN_POINT('Ctrl Pts',(2.06695359164605,5.7122071046112,8.08312913572091E-15));
#13313=CARTESIAN_POINT('Ctrl Pts',(1.90699906471761,5.78228482847051,5.00728262377208E-15));
#13314=CARTESIAN_POINT('Ctrl Pts',(1.74412150459255,5.84526005779857,3.66373598126302E-15));
#13315=CARTESIAN_POINT('Ctrl Pts',(1.68944058194602,5.86640197348599,3.0447967981167E-15));
#13316=CARTESIAN_POINT('Ctrl Pts',(1.6344299541403,5.88674298606999,3.67419985746786E-15));
#13317=CARTESIAN_POINT('Ctrl Pts',(1.57910765804983,5.90628229011343,4.44089209850063E-15));
#13318=CARTESIAN_POINT('Ctrl Pts',(-2.03514912955913,4.71639359924028,20.0001232957739));
#13319=CARTESIAN_POINT('Ctrl Pts',(-2.0338211300873,4.71696663813373,20.0000821971826));
#13320=CARTESIAN_POINT('Ctrl Pts',(-2.03249288858879,4.71753911613801,20.0000410985913));
#13321=CARTESIAN_POINT('Ctrl Pts',(-2.03116440553748,4.71811103304888,20.));
#13322=CARTESIAN_POINT('Ctrl Pts',(-1.57898373554274,5.90622195601506,0.000227687169849418));
#13323=CARTESIAN_POINT('Ctrl Pts',(-2.56111970282799,5.64365533898239,0.0465425127055785));
#13324=CARTESIAN_POINT('Ctrl Pts',(-4.39088445035941,4.61937212663427,0.139172163777036));
#13325=CARTESIAN_POINT('Ctrl Pts',(-6.0657765047469,1.95510796653054,0.278116640384223));
#13326=CARTESIAN_POINT('Ctrl Pts',(-6.26190048847721,-1.18494435610987,
0.41706111699141));
#13327=CARTESIAN_POINT('Ctrl Pts',(-4.93182523694634,-4.03654277149442,
0.556005593598598));
#13328=CARTESIAN_POINT('Ctrl Pts',(-2.39956484444413,-5.90405390794762,
0.694950070205784));
#13329=CARTESIAN_POINT('Ctrl Pts',(0.717551765537385,-6.33256105617076,
0.833894546812973));
#13330=CARTESIAN_POINT('Ctrl Pts',(3.65978322840781,-5.21747149734623,0.972839023420158));
#13331=CARTESIAN_POINT('Ctrl Pts',(5.70994220793149,-2.83065972743125,1.11178350002735));
#13332=CARTESIAN_POINT('Ctrl Pts',(6.36831967964836,0.246131796845876,1.25072797663453));
#13333=CARTESIAN_POINT('Ctrl Pts',(5.47443112253067,3.26292276856099,1.38967245324172));
#13334=CARTESIAN_POINT('Ctrl Pts',(3.24616319142365,5.48438682410978,1.52861692984891));
#13335=CARTESIAN_POINT('Ctrl Pts',(0.226649590892417,6.36904203396657,1.66756140645609));
#13336=CARTESIAN_POINT('Ctrl Pts',(-2.84810905785752,5.70125818109619,1.80650588306328));
#13337=CARTESIAN_POINT('Ctrl Pts',(-5.22864756594639,3.64380481219555,1.94545035967047));
#13338=CARTESIAN_POINT('Ctrl Pts',(-6.33471471180235,0.698182296261472,
2.08439483627765));
#13339=CARTESIAN_POINT('Ctrl Pts',(-5.89670918641703,-2.4176207243154,2.22333931288484));
#13340=CARTESIAN_POINT('Ctrl Pts',(-4.02139381088499,-4.94413397937359,
2.36228378949203));
#13341=CARTESIAN_POINT('Ctrl Pts',(-1.16587259232897,-6.26552553432391,
2.50122826609921));
#13342=CARTESIAN_POINT('Ctrl Pts',(1.97382749872696,-6.05970907400165,2.6401727427064));
#13343=CARTESIAN_POINT('Ctrl Pts',(4.63241149714395,-4.37685192827009,2.77911721931359));
#13344=CARTESIAN_POINT('Ctrl Pts',(6.1618554334486,-1.62714679528568,2.91806169592078));
#13345=CARTESIAN_POINT('Ctrl Pts',(6.18936072671635,1.51917177059382,3.05700617252796));
#13346=CARTESIAN_POINT('Ctrl Pts',(4.70822302351486,4.2951955762199,3.19595064913515));
#13347=CARTESIAN_POINT('Ctrl Pts',(2.07946636473173,6.02427495328891,3.33489512574233));
#13348=CARTESIAN_POINT('Ctrl Pts',(-1.05615562412742,6.28495062619459,3.47383960234952));
#13349=CARTESIAN_POINT('Ctrl Pts',(-3.93434201406849,5.01368347544235,3.61278407895671));
#13350=CARTESIAN_POINT('Ctrl Pts',(-5.85354123412349,2.52034205935053,3.7517285555639));
#13351=CARTESIAN_POINT('Ctrl Pts',(-6.34595271643967,-0.587327163036974,
3.89067303217109));
#13352=CARTESIAN_POINT('Ctrl Pts',(-5.29155225056067,-3.55183668758433,
4.02961750877827));
#13353=CARTESIAN_POINT('Ctrl Pts',(-2.94734761951486,-5.65059387015744,
4.16856198538546));
#13354=CARTESIAN_POINT('Ctrl Pts',(0.115266479274401,-6.37203128636819,
4.30750646199265));
#13355=CARTESIAN_POINT('Ctrl Pts',(3.14978462851293,-5.54030016061337,4.44645093859983));
#13356=CARTESIAN_POINT('Ctrl Pts',(5.4165497365127,-3.35813311641903,4.58539541520702));
#13357=CARTESIAN_POINT('Ctrl Pts',(6.36304281842322,-0.35742854757112,4.7243398918142));
#13358=CARTESIAN_POINT('Ctrl Pts',(5.75855827756034,2.73039843972416,4.8632843684214));
#13359=CARTESIAN_POINT('Ctrl Pts',(3.75043788466858,5.15269684232915,5.00222884502858));
#13360=CARTESIAN_POINT('Ctrl Pts',(0.828156546972091,6.31903677860904,5.14117332163577));
#13361=CARTESIAN_POINT('Ctrl Pts',(-2.29598611857659,5.94512546705365,5.28011779824296));
#13362=CARTESIAN_POINT('Ctrl Pts',(-4.8604872425344,4.12210296339946,5.41906227485014));
#13363=CARTESIAN_POINT('Ctrl Pts',(-6.2402553442469,1.29432697349022,5.55800675145734));
#13364=CARTESIAN_POINT('Ctrl Pts',(-6.09897499861954,-1.84893835535969,
5.69695122806451));
#13365=CARTESIAN_POINT('Ctrl Pts',(-4.47108297762739,-4.54152904679438,
5.83589570467171));
#13366=CARTESIAN_POINT('Ctrl Pts',(-1.75337436326174,-6.12713207120288,
5.97484018127889));
#13367=CARTESIAN_POINT('Ctrl Pts',(1.39171537667014,-6.21926019603992,6.11378465788608));
#13368=CARTESIAN_POINT('Ctrl Pts',(4.19757756964354,-4.79545739450698,6.25272913449327));
#13369=CARTESIAN_POINT('Ctrl Pts',(5.98028950791123,-2.20277245245013,6.39167361110045));
#13370=CARTESIAN_POINT('Ctrl Pts',(6.30531909684407,0.926833406109166,6.53061808770763));
#13371=CARTESIAN_POINT('Ctrl Pts',(5.09344109255171,3.83052567050686,6.66956256431483));
#13372=CARTESIAN_POINT('Ctrl Pts',(2.6400480799696,5.80053576931951,6.80850704092201));
#13373=CARTESIAN_POINT('Ctrl Pts',(-0.456850816813612,6.35667809526981,
6.9474515175292));
#13374=CARTESIAN_POINT('Ctrl Pts',(-3.44239333677469,5.36339418564733,7.08639599413638));
#13375=CARTESIAN_POINT('Ctrl Pts',(-5.58886008961009,3.06279479796965,7.22534047074357));
#13376=CARTESIAN_POINT('Ctrl Pts',(-6.37305454864607,0.0156459479743102,
7.36428494735076));
#13377=CARTESIAN_POINT('Ctrl Pts',(-5.60383104779562,-3.03531656725757,
7.50322942395795));
#13378=CARTESIAN_POINT('Ctrl Pts',(-3.4686861151783,-5.34642737817279,7.64217390056513));
#13379=CARTESIAN_POINT('Ctrl Pts',(-0.488056608814282,-6.35435833285306,
7.78111837717233));
#13380=CARTESIAN_POINT('Ctrl Pts',(2.61153561719795,-5.81342848892225,7.9200628537795));
#13381=CARTESIAN_POINT('Ctrl Pts',(5.07457180878865,-3.85548830022266,8.0590073303867));
#13382=CARTESIAN_POINT('Ctrl Pts',(6.30069233830012,-0.957781360119654,
8.19795180699388));
#13383=CARTESIAN_POINT('Ctrl Pts',(5.99103303675496,2.17338266953084,8.33689628360107));
#13384=CARTESIAN_POINT('Ctrl Pts',(4.22107267446567,4.77478947730533,8.47584076020826));
#13385=CARTESIAN_POINT('Ctrl Pts',(1.42223517760143,6.21235190369149,8.61478523681544));
#13386=CARTESIAN_POINT('Ctrl Pts',(-1.7232690002404,6.13566728469829,8.75372971342263));
#13387=CARTESIAN_POINT('Ctrl Pts',(-4.44873016821067,4.56342732670946,8.89267419002982));
#13388=CARTESIAN_POINT('Ctrl Pts',(-6.08982319069643,1.87886204436686,9.031618666637));
#13389=CARTESIAN_POINT('Ctrl Pts',(-6.24653527077042,-1.26367170844621,
9.1705631432442));
#13390=CARTESIAN_POINT('Ctrl Pts',(-4.88066818529498,-4.09818827541583,
9.30950761985137));
#13391=CARTESIAN_POINT('Ctrl Pts',(-2.32514901738218,-5.93378050846787,
9.44845209645857));
#13392=CARTESIAN_POINT('Ctrl Pts',(0.797120084246647,-6.32302685800061,
9.58739657306574));
#13393=CARTESIAN_POINT('Ctrl Pts',(3.72509292721283,-5.17104938666566,9.72634104967295));
#13394=CARTESIAN_POINT('Ctrl Pts',(5.74508260273416,-2.75864005688811,9.86528552628012));
#13395=CARTESIAN_POINT('Ctrl Pts',(6.36472109218032,0.3261816893409,10.0042300028873));
#13396=CARTESIAN_POINT('Ctrl Pts',(5.43297288333417,3.33149736975161,10.1431744794944));
#13397=CARTESIAN_POINT('Ctrl Pts',(3.17694954266129,5.52476792988544,10.2821189561018));
#13398=CARTESIAN_POINT('Ctrl Pts',(0.146551772968109,6.37138851849,10.4210634327089));
#13399=CARTESIAN_POINT('Ctrl Pts',(-2.91956766746306,5.66499723837627,10.560007909316));
#13400=CARTESIAN_POINT('Ctrl Pts',(-5.27404894206298,3.57777540273711,10.6989523859233));
#13401=CARTESIAN_POINT('Ctrl Pts',(-6.34299244425185,0.618478720628544,
10.8378968625304));
#13402=CARTESIAN_POINT('Ctrl Pts',(-5.86584555805418,-2.49157078261131,
10.9768413391376));
#13403=CARTESIAN_POINT('Ctrl Pts',(-3.95891178234414,-4.99430541470214,
11.1157858157449));
#13404=CARTESIAN_POINT('Ctrl Pts',(-1.08700201006022,-6.27968914085971,
11.254730292352));
#13405=CARTESIAN_POINT('Ctrl Pts',(2.04986209957812,-6.03441251891346,11.3936747689591));
#13406=CARTESIAN_POINT('Ctrl Pts',(4.6870768532492,-4.31826118332852,11.5326192455664));
#13407=CARTESIAN_POINT('Ctrl Pts',(6.18182698377473,-1.54954322894881,11.6715637221736));
#13408=CARTESIAN_POINT('Ctrl Pts',(6.16977045068138,1.59687246253577,11.8105081987807));
#13409=CARTESIAN_POINT('Ctrl Pts',(4.65384600726222,4.35405402084034,11.949452675388));
#13410=CARTESIAN_POINT('Ctrl Pts',(2.0035568859567,6.04994453531947,12.0883971519952));
#13411=CARTESIAN_POINT('Ctrl Pts',(-1.13509479784413,6.27117444149129,12.2273416286023));
#13412=CARTESIAN_POINT('Ctrl Pts',(-3.99706963356756,4.96381943871032,12.3662861052095));
#13413=CARTESIAN_POINT('Ctrl Pts',(-5.88476758082163,2.44654441926103,12.5052305818167));
#13414=CARTESIAN_POINT('Ctrl Pts',(-6.33806643733701,-0.667070394792312,
12.6441750584238));
#13415=CARTESIAN_POINT('Ctrl Pts',(-5.24647560876346,-3.61808827453898,
12.783119535031));
#13416=CARTESIAN_POINT('Ctrl Pts',(-2.87606794682533,-5.68720513441799,
12.9220640116383));
#13417=CARTESIAN_POINT('Ctrl Pts',(0.195374920185906,-6.37007831319747,
13.0610084882454));
#13418=CARTESIAN_POINT('Ctrl Pts',(3.2191955822385,-5.50025898290275,13.1999529648527));
#13419=CARTESIAN_POINT('Ctrl Pts',(5.45834443650017,-3.28976368273376,13.3388974414599));
#13420=CARTESIAN_POINT('Ctrl Pts',(6.36703389892958,-0.27739575625459,13.477841918067));
#13421=CARTESIAN_POINT('Ctrl Pts',(5.7237729215335,2.80258677268451,13.6167863946742));
#13422=CARTESIAN_POINT('Ctrl Pts',(3.68535494575419,5.19944497033206,13.7557308712814));
#13423=CARTESIAN_POINT('Ctrl Pts',(0.748639847677835,6.32894994878103,13.8946753478885));
#13424=CARTESIAN_POINT('Ctrl Pts',(-2.37055455855325,5.91578736607636,14.0336198244957));
#13425=CARTESIAN_POINT('Ctrl Pts',(-4.91193153076762,4.06066468854018,14.172564301103));
#13426=CARTESIAN_POINT('Ctrl Pts',(-6.25603604918701,1.21576396844905,14.3115087777102));
#13427=CARTESIAN_POINT('Ctrl Pts',(-6.07524560831743,-1.92547653175161,
14.4504532543174));
#13428=CARTESIAN_POINT('Ctrl Pts',(-4.41362747852017,-4.59738638321363,
14.5893977309245));
#13429=CARTESIAN_POINT('Ctrl Pts',(-1.67619740626309,-6.14869346535858,
14.7283422075317));
#13430=CARTESIAN_POINT('Ctrl Pts',(1.46980207887581,-6.20127010576371,14.8672866841389));
#13431=CARTESIAN_POINT('Ctrl Pts',(4.25754055598848,-4.74230086454031,15.0062311607461));
#13432=CARTESIAN_POINT('Ctrl Pts',(6.00751293300991,-2.12740626948055,15.1451756373533));
#13433=CARTESIAN_POINT('Ctrl Pts',(6.2931673110005,1.00603890156448,15.2841201139604));
#13434=CARTESIAN_POINT('Ctrl Pts',(5.04487606670623,3.89426431399836,15.4230645905676));
#13435=CARTESIAN_POINT('Ctrl Pts',(2.56690743182888,5.83327140737748,15.5620090671748));
#13436=CARTESIAN_POINT('Ctrl Pts',(-0.536739215927813,6.3504314884732,15.7009535437819));
#13437=CARTESIAN_POINT('Ctrl Pts',(-3.50955686615555,5.3196879305958,15.8398980203891));
#13438=CARTESIAN_POINT('Ctrl Pts',(-5.62692778742215,2.99228219772843,15.9788424969964));
#13439=CARTESIAN_POINT('Ctrl Pts',(-6.37274749768898,-0.0644857070020716,
16.1177869736036));
#13440=CARTESIAN_POINT('Ctrl Pts',(-5.56522409106071,-3.10553536318246,
16.2567314502108));
#13441=CARTESIAN_POINT('Ctrl Pts',(-3.40118961303849,-5.3896176387458,16.395675926818));
#13442=CARTESIAN_POINT('Ctrl Pts',(-0.408122684475576,-6.35999252751921,
16.5346204034251));
#13443=CARTESIAN_POINT('Ctrl Pts',(2.68442324634952,-5.78013329519202,16.6735648800323));
#13444=CARTESIAN_POINT('Ctrl Pts',(5.1226469442629,-3.79137934796153,16.8125093566395));
#13445=CARTESIAN_POINT('Ctrl Pts',(6.31223677206156,-0.878485064768902,
16.9514538332466));
#13446=CARTESIAN_POINT('Ctrl Pts',(5.96323283863802,2.24853801130179,17.0903983098538));
#13447=CARTESIAN_POINT('Ctrl Pts',(4.16070408122212,4.82748491694963,17.2293427864611));
#13448=CARTESIAN_POINT('Ctrl Pts',(1.34401290058344,6.22974304447622,17.3682872630683));
#13449=CARTESIAN_POINT('Ctrl Pts',(-1.80027845426065,6.11351507408893,17.5072317396755));
#13450=CARTESIAN_POINT('Ctrl Pts',(-4.50575591432981,4.50713131787952,17.6461762162826));
#13451=CARTESIAN_POINT('Ctrl Pts',(-6.11296533071532,1.8021442634666,17.7851206928898));
#13452=CARTESIAN_POINT('Ctrl Pts',(-6.23015295651432,-1.3421114688075,17.924065169497));
#13453=CARTESIAN_POINT('Ctrl Pts',(-4.82875457494639,-4.15923050307904,
18.0630096461041));
#13454=CARTESIAN_POINT('Ctrl Pts',(-2.25035792833039,-5.96254628347833,
18.2019541227113));
#13455=CARTESIAN_POINT('Ctrl Pts',(0.876558468963431,-6.31250460960645,
18.3408985993185));
#13456=CARTESIAN_POINT('Ctrl Pts',(3.78981571693129,-5.12380384386822,18.4798430759257));
#13457=CARTESIAN_POINT('Ctrl Pts',(5.77931368194271,-2.68618730619559,18.6187875525329));
#13458=CARTESIAN_POINT('Ctrl Pts',(6.3601168652194,0.406181626514434,18.7577320291401));
#13459=CARTESIAN_POINT('Ctrl Pts',(5.39065531759173,3.39954433923207,18.8966765057473));
#13460=CARTESIAN_POINT('Ctrl Pts',(3.10723404554619,5.56427631305468,19.0356209823545));
#13461=CARTESIAN_POINT('Ctrl Pts',(0.0664301762482525,6.37272689989223,
19.1745654589617));
#13462=CARTESIAN_POINT('Ctrl Pts',(-2.99056361179,5.62784200981625,19.3135099355688));
#13463=CARTESIAN_POINT('Ctrl Pts',(-5.31861862440418,3.51117792749949,19.452454412176));
#13464=CARTESIAN_POINT('Ctrl Pts',(-6.35026327979242,0.538682078665528,
19.5913988887833));
#13465=CARTESIAN_POINT('Ctrl Pts',(-5.83406261636922,-2.56513614738856,
19.7303433653904));
#13466=CARTESIAN_POINT('Ctrl Pts',(-3.89578808605346,-5.04366921786192,
19.8692878419977));
#13467=CARTESIAN_POINT('Ctrl Pts',(-1.00799057796779,-6.29289541535634,
20.0082323186047));
#13468=CARTESIAN_POINT('Ctrl Pts',(2.12563365775662,-6.0080922436061,20.147176795212));
#13469=CARTESIAN_POINT('Ctrl Pts',(4.74087939902799,-4.25912600074273,20.2861212718192));
#13470=CARTESIAN_POINT('Ctrl Pts',(6.20114346261515,-1.4712913257721,20.4250715454063));
#13471=CARTESIAN_POINT('Ctrl Pts',(6.16597040977451,0.625509887000643,20.5177069934577));
#13472=CARTESIAN_POINT('Ctrl Pts',(5.89878813698322,1.60653227262758,20.5640276159734));
#13473=CARTESIAN_POINT('Ctrl Pts',(-1.49483566411598,5.59146432056281,-0.187879788315434));
#13474=CARTESIAN_POINT('Ctrl Pts',(-2.42463110016866,5.34289054838787,-0.141564962779705));
#13475=CARTESIAN_POINT('Ctrl Pts',(-4.15688301637475,4.37319400148394,-0.0489353117082476));
#13476=CARTESIAN_POINT('Ctrl Pts',(-5.74251580035167,1.85091527530052,0.0900091648989393));
#13477=CARTESIAN_POINT('Ctrl Pts',(-5.92818783665532,-1.12179564845051,
0.228953641506126));
#13478=CARTESIAN_POINT('Ctrl Pts',(-4.66899568844553,-3.82142510954073,
0.367898118113314));
#13479=CARTESIAN_POINT('Ctrl Pts',(-2.27168591233214,-5.58941181330781,
0.5068425947205));
#13480=CARTESIAN_POINT('Ctrl Pts',(0.6793116013991,-5.99508272243367,0.645787071327689));
#13481=CARTESIAN_POINT('Ctrl Pts',(3.46474404365988,-4.93941913091394,0.784731547934873));
#13482=CARTESIAN_POINT('Ctrl Pts',(5.40564482098563,-2.67980664923482,0.923676024542063));
#13483=CARTESIAN_POINT('Ctrl Pts',(6.02893567764199,0.233014805482908,1.06262050114925));
#13484=CARTESIAN_POINT('Ctrl Pts',(5.1826847221403,3.08903329015262,1.20156497775644));
#13485=CARTESIAN_POINT('Ctrl Pts',(3.07316687363643,5.19210985898417,1.34050945436363));
#13486=CARTESIAN_POINT('Ctrl Pts',(0.214570855985937,6.02961953585579,1.47945393097081));
#13487=CARTESIAN_POINT('Ctrl Pts',(-2.69632606032752,5.39742358809429,1.618398407578));
#13488=CARTESIAN_POINT('Ctrl Pts',(-4.94999959830705,3.44961715801027,1.75734288418519));
#13489=CARTESIAN_POINT('Ctrl Pts',(-5.99712160426244,0.66097438055453,1.89628736079237));
#13490=CARTESIAN_POINT('Ctrl Pts',(-5.58245851072475,-2.28877954830255,
2.03523183739956));
#13491=CARTESIAN_POINT('Ctrl Pts',(-3.80708347568884,-4.68064846658789,
2.17417631400675));
#13492=CARTESIAN_POINT('Ctrl Pts',(-1.10374026761565,-5.93161969456096,
2.31312079061393));
#13493=CARTESIAN_POINT('Ctrl Pts',(1.86863719587062,-5.73677171846951,2.45206526722112));
#13494=CARTESIAN_POINT('Ctrl Pts',(4.3855384706743,-4.14359832318604,2.59100974382831));
#13495=CARTESIAN_POINT('Ctrl Pts',(5.83347443783502,-1.54043199153601,2.72995422043549));
#13496=CARTESIAN_POINT('Ctrl Pts',(5.85951390385553,1.43821123136604,2.86889869704268));
#13497=CARTESIAN_POINT('Ctrl Pts',(4.45730980740144,4.06629364645088,3.00784317364986));
#13498=CARTESIAN_POINT('Ctrl Pts',(1.96864629720973,5.70322597244586,3.14678765025706));
#13499=CARTESIAN_POINT('Ctrl Pts',(-0.999870396549506,5.95000957373033,
3.28573212686423));
#13500=CARTESIAN_POINT('Ctrl Pts',(-3.72467089120331,4.74649149258279,3.42467660347143));
#13501=CARTESIAN_POINT('Ctrl Pts',(-5.54159108873511,2.38602660134033,3.56362108007861));
#13502=CARTESIAN_POINT('Ctrl Pts',(-6.00776070696327,-0.5560270001831,3.7025655566858));
#13503=CARTESIAN_POINT('Ctrl Pts',(-5.00955193180152,-3.36255024938027,
3.84151003329299));
#13504=CARTESIAN_POINT('Ctrl Pts',(-2.79027594586576,-5.34945930753565,
3.98045450990018));
#13505=CARTESIAN_POINT('Ctrl Pts',(0.109123634536512,-6.03244948337102,
4.11939898650736));
#13506=CARTESIAN_POINT('Ctrl Pts',(2.98192457021544,-5.24504343114447,4.25834346311455));
#13507=CARTESIAN_POINT('Ctrl Pts',(5.12788798284495,-3.1791696356813,4.39728793972173));
#13508=CARTESIAN_POINT('Ctrl Pts',(6.0239400338134,-0.338380268431863,4.53623241632893));
#13509=CARTESIAN_POINT('Ctrl Pts',(5.45167001623907,2.58488854132713,4.67517689293611));
#13510=CARTESIAN_POINT('Ctrl Pts',(3.5505674820186,4.87809648250993,4.8141213695433));
#13511=CARTESIAN_POINT('Ctrl Pts',(0.784021971866293,5.98227918812514,4.95306584615048));
#13512=CARTESIAN_POINT('Ctrl Pts',(-2.17362716100671,5.62829456425105,5.09201032275767));
#13513=CARTESIAN_POINT('Ctrl Pts',(-4.60145947774681,3.90242558054578,5.23095479936486));
#13514=CARTESIAN_POINT('Ctrl Pts',(-5.90769621738016,1.22534898710367,5.36989927597204));
#13515=CARTESIAN_POINT('Ctrl Pts',(-5.77394506179285,-1.75040371355922,
5.50884375257924));
#13516=CARTESIAN_POINT('Ctrl Pts',(-4.23280755952943,-4.29949937795489,
5.64778822918641));
#13517=CARTESIAN_POINT('Ctrl Pts',(-1.65993257039433,-5.80060157214647,
5.78673270579361));
#13518=CARTESIAN_POINT('Ctrl Pts',(1.3175473138297,-5.88781995418203,5.92567718240079));
#13519=CARTESIAN_POINT('Ctrl Pts',(3.97387795247917,-4.539895236219,6.06462165900799));
#13520=CARTESIAN_POINT('Ctrl Pts',(5.66158462366403,-2.08538108894634,6.20356613561516));
#13521=CARTESIAN_POINT('Ctrl Pts',(5.9692925566167,0.877440089444528,6.34251061222236));
#13522=CARTESIAN_POINT('Ctrl Pts',(4.82199862280603,3.62638718543689,6.48145508882954));
#13523=CARTESIAN_POINT('Ctrl Pts',(2.4993531827375,5.49141042037324,6.62039956543673));
#13524=CARTESIAN_POINT('Ctrl Pts',(-0.432504071309366,6.01791450299395,
6.75934404204391));
#13525=CARTESIAN_POINT('Ctrl Pts',(-3.25893941393721,5.07756522689079,6.8982885186511));
#13526=CARTESIAN_POINT('Ctrl Pts',(-5.29101547764327,2.89957064966237,7.03723299525829));
#13527=CARTESIAN_POINT('Ctrl Pts',(-6.03341821339165,0.0148121354922382,
7.17617747186546));
#13528=CARTESIAN_POINT('Ctrl Pts',(-5.30518859527455,-2.87355680396488,
7.31512194847268));
#13529=CARTESIAN_POINT('Ctrl Pts',(-3.28383098310395,-5.06150262387076,
7.45406642507984));
#13530=CARTESIAN_POINT('Ctrl Pts',(-0.462046827044943,-6.01571836663433,
7.59301090168704));
#13531=CARTESIAN_POINT('Ctrl Pts',(2.47236022184536,-5.50361605405762,7.73195537829422));
#13532=CARTESIAN_POINT('Ctrl Pts',(4.8041349313123,-3.65001949293274,7.87089985490142));
#13533=CARTESIAN_POINT('Ctrl Pts',(5.96491236983892,-0.906738748034197,
8.00984433150859));
#13534=CARTESIAN_POINT('Ctrl Pts',(5.67175560244776,2.05755756253537,8.1487888081158));
#13535=CARTESIAN_POINT('Ctrl Pts',(3.99612094322675,4.52032876505112,8.28773328472297));
#13536=CARTESIAN_POINT('Ctrl Pts',(1.34644063671004,5.88127982235669,8.42667776133016));
#13537=CARTESIAN_POINT('Ctrl Pts',(-1.63143159897046,5.80868192234044,8.56562223793735));
#13538=CARTESIAN_POINT('Ctrl Pts',(-4.21164598835098,4.32023064266841,8.70456671454454));
#13539=CARTESIAN_POINT('Ctrl Pts',(-5.76528097706123,1.7787326928406,8.84351119115172));
#13540=CARTESIAN_POINT('Ctrl Pts',(-5.91364147059847,-1.19632741933878,
8.98245566775891));
#13541=CARTESIAN_POINT('Ctrl Pts',(-4.62056492658388,-3.87978536729377,
9.1214001443661));
#13542=CARTESIAN_POINT('Ctrl Pts',(-2.20123589453721,-5.61755420745052,
9.26034462097328));
#13543=CARTESIAN_POINT('Ctrl Pts',(0.754639521416892,-5.98605662600678,
9.39928909758048));
#13544=CARTESIAN_POINT('Ctrl Pts',(3.52657322200342,-4.89547097293942,9.53823357418765));
#13545=CARTESIAN_POINT('Ctrl Pts',(5.4389124945023,-2.61162509066496,9.67717805079486));
#13546=CARTESIAN_POINT('Ctrl Pts',(6.02552886808051,0.308798634990865,9.81612252740202));
#13547=CARTESIAN_POINT('Ctrl Pts',(5.14343589827507,3.15395337590449,9.95506700400922));
#13548=CARTESIAN_POINT('Ctrl Pts',(3.00764179678818,5.23033895261644,10.0940114806164));
#13549=CARTESIAN_POINT('Ctrl Pts',(0.138741655117083,6.03184097023283,10.2329559572236));
#13550=CARTESIAN_POINT('Ctrl Pts',(-2.76397645832849,5.36309508351754,10.3719004338308));
#13551=CARTESIAN_POINT('Ctrl Pts',(-4.99298141926652,3.38710662423008,10.510844910438));
#13552=CARTESIAN_POINT('Ctrl Pts',(-6.0049581952323,0.585518411799595,10.6497893870452));
#13553=CARTESIAN_POINT('Ctrl Pts',(-5.55323968385385,-2.35878861933721,
10.7887338636523));
#13554=CARTESIAN_POINT('Ctrl Pts',(-3.74793127384739,-4.72814613813498,
10.9276783402595));
#13555=CARTESIAN_POINT('Ctrl Pts',(-1.02907289988345,-5.94502848637157,
11.0666228168667));
#13556=CARTESIAN_POINT('Ctrl Pts',(1.94061971886987,-5.71282328133623,11.2055672934739));
#13557=CARTESIAN_POINT('Ctrl Pts',(4.43729057049544,-4.08813002851381,11.3445117700811));
#13558=CARTESIAN_POINT('Ctrl Pts',(5.85238165329467,-1.46696411722439,11.4834562466883));
#13559=CARTESIAN_POINT('Ctrl Pts',(5.84096764360742,1.51177105521146,11.6224007232955));
#13560=CARTESIAN_POINT('Ctrl Pts',(4.4058306810666,4.1220153744032,11.7613451999027));
#13561=CARTESIAN_POINT('Ctrl Pts',(1.89678222821199,5.72752755696409,11.9002896765098));
#13562=CARTESIAN_POINT('Ctrl Pts',(-1.07460270031642,5.93696755705441,12.039234153117));
#13563=CARTESIAN_POINT('Ctrl Pts',(-3.78405559583427,4.69928483757681,12.1781786297242));
#13564=CARTESIAN_POINT('Ctrl Pts',(-5.57115330375587,2.31616182575703,12.3171231063314));
#13565=CARTESIAN_POINT('Ctrl Pts',(-6.00029470779274,-0.631520511684512,
12.4560675829386));
#13566=CARTESIAN_POINT('Ctrl Pts',(-4.9668775392411,-3.42527112025111,12.5950120595458));
#13567=CARTESIAN_POINT('Ctrl Pts',(-2.72279494877608,-5.38411946412442,
12.733956536153));
#13568=CARTESIAN_POINT('Ctrl Pts',(0.184962892266474,-6.03060058912282,
12.8729010127602));
#13569=CARTESIAN_POINT('Ctrl Pts',(3.04763643714207,-5.20713614994345,13.0118454893673));
#13570=CARTESIAN_POINT('Ctrl Pts',(5.16745533664726,-3.114443783535,13.1507899659745));
#13571=CARTESIAN_POINT('Ctrl Pts',(6.02771841945788,-0.262612628736961,
13.2897344425817));
#13572=CARTESIAN_POINT('Ctrl Pts',(5.41873846057615,2.6532297738637,13.4286789191889));
#13573=CARTESIAN_POINT('Ctrl Pts',(3.48895297895264,4.92235328351202,13.5676233957961));
#13574=CARTESIAN_POINT('Ctrl Pts',(0.7087429203332,5.99166406016906,13.7065678724033));
#13575=CARTESIAN_POINT('Ctrl Pts',(-2.24422165858479,5.60051996551953,13.8455123490105));
#13576=CARTESIAN_POINT('Ctrl Pts',(-4.65016216862009,3.84426150808949,13.9844568256176));
#13577=CARTESIAN_POINT('Ctrl Pts',(-5.92263592829572,1.15097280502394,14.1234013022249));
#13578=CARTESIAN_POINT('Ctrl Pts',(-5.75148027123621,-1.82286297527398,
14.262345778832));
#13579=CARTESIAN_POINT('Ctrl Pts',(-4.17841401054488,-4.35237993441822,
14.4012902554392));
#13580=CARTESIAN_POINT('Ctrl Pts',(-1.58686857032097,-5.82101390460213,
14.5402347320464));
#13581=CARTESIAN_POINT('Ctrl Pts',(1.39147257646715,-5.87078860171135,14.6791792086536));
#13582=CARTESIAN_POINT('Ctrl Pts',(4.03064535830965,-4.48957155334236,14.8181236852608));
#13583=CARTESIAN_POINT('Ctrl Pts',(5.68735724298926,-2.01403136213456,14.957068161868));
#13584=CARTESIAN_POINT('Ctrl Pts',(5.95778837044127,0.952424521985176,15.0960126384751));
#13585=CARTESIAN_POINT('Ctrl Pts',(4.77602175108252,3.6867290340125,15.2349571150823));
#13586=CARTESIAN_POINT('Ctrl Pts',(2.43011038632597,5.52240149276691,15.3739015916895));
#13587=CARTESIAN_POINT('Ctrl Pts',(-0.508135013830756,6.0120007938093,15.5128460682967));
#13588=CARTESIAN_POINT('Ctrl Pts',(-3.32252362749587,5.03618818967038,15.6517905449039));
#13589=CARTESIAN_POINT('Ctrl Pts',(-5.32705445072409,2.83281584577332,15.7907350215111));
#13590=CARTESIAN_POINT('Ctrl Pts',(-6.03312752596339,-0.0610490991658619,
15.9296794981182));
#13591=CARTESIAN_POINT('Ctrl Pts',(-5.26863910175461,-2.94003346111913,
16.0686239747255));
#13592=CARTESIAN_POINT('Ctrl Pts',(-3.21993154175411,-5.10239116527476,
16.2075684513326));
#13593=CARTESIAN_POINT('Ctrl Pts',(-0.386372785454403,-6.02105230069328,
16.3465129279398));
#13594=CARTESIAN_POINT('Ctrl Pts',(2.54136348329514,-5.47209524614095,16.485457404547));
#13595=CARTESIAN_POINT('Ctrl Pts',(4.84964802017221,-3.58932707028654,16.6244018811542));
#13596=CARTESIAN_POINT('Ctrl Pts',(5.97584157127411,-0.831668354556176,
16.7633463577614));
#13597=CARTESIAN_POINT('Ctrl Pts',(5.6454369478098,2.12870768441387,16.9022908343686));
#13598=CARTESIAN_POINT('Ctrl Pts',(3.93896954632401,4.57021593028499,17.0412353109758));
#13599=CARTESIAN_POINT('Ctrl Pts',(1.27238702438789,5.89774414488229,17.1801797875829));
#13600=CARTESIAN_POINT('Ctrl Pts',(-1.70433702272646,5.78771025954717,17.3191242641901));
#13601=CARTESIAN_POINT('Ctrl Pts',(-4.26563268698053,4.26693479176628,17.4580687407973));
#13602=CARTESIAN_POINT('Ctrl Pts',(-5.78718981340038,1.70610339819993,17.5970132174045));
#13603=CARTESIAN_POINT('Ctrl Pts',(-5.89813221166215,-1.27058692476204,
17.7359576940117));
#13604=CARTESIAN_POINT('Ctrl Pts',(-4.57141792496805,-3.93757449891943,
17.8749021706189));
#13605=CARTESIAN_POINT('Ctrl Pts',(-2.13043061342123,-5.64478698092605,
18.0138466472261));
#13606=CARTESIAN_POINT('Ctrl Pts',(0.829844431956138,-5.97609513507295,
18.1527911238333));
#13607=CARTESIAN_POINT('Ctrl Pts',(3.58784676914289,-4.85074326564618,18.2917356004405));
#13608=CARTESIAN_POINT('Ctrl Pts',(5.47131931217262,-2.54303353189171,18.4306800770476));
#13609=CARTESIAN_POINT('Ctrl Pts',(6.02117001212022,0.38453517142386,18.5696245536548));
#13610=CARTESIAN_POINT('Ctrl Pts',(5.10337354356777,3.2183739487861,18.708569030262));
#13611=CARTESIAN_POINT('Ctrl Pts',(2.94164161636617,5.2677418332564,18.8475135068692));
#13612=CARTESIAN_POINT('Ctrl Pts',(0.0628899426853606,6.03310802587577,
18.9864579834764));
#13613=CARTESIAN_POINT('Ctrl Pts',(-2.83118884766385,5.32791995187452,19.1254024600835));
#13614=CARTESIAN_POINT('Ctrl Pts',(-5.03517586953364,3.32405829834529,19.2643469366908));
#13615=CARTESIAN_POINT('Ctrl Pts',(-6.01184154939821,0.509974336456724,
19.4032914132979));
#13616=CARTESIAN_POINT('Ctrl Pts',(-5.52315053621304,-2.42843349815221,
19.5422358899051));
#13617=CARTESIAN_POINT('Ctrl Pts',(-3.68817160036747,-4.77487921829192,
19.6811803665123));
#13618=CARTESIAN_POINT('Ctrl Pts',(-0.954272188574022,-5.95753096480961,
19.8201248431195));
#13619=CARTESIAN_POINT('Ctrl Pts',(2.01235321741153,-5.68790568064591,19.9590693197267));
#13620=CARTESIAN_POINT('Ctrl Pts',(4.48822584135349,-4.03214631066831,20.0980137963339));
#13621=CARTESIAN_POINT('Ctrl Pts',(5.87066870769925,-1.39288245759711,20.236964069921));
#13622=CARTESIAN_POINT('Ctrl Pts',(5.83737011657478,0.592174869378453,20.3295995179724));
#13623=CARTESIAN_POINT('Ctrl Pts',(5.58442666871165,1.52091606938026,20.3759201404881));
#13624=CARTESIAN_POINT('Ctrl Pts',(-1.41068759268922,5.27670668511055,-0.375987263800719));
#13625=CARTESIAN_POINT('Ctrl Pts',(-2.28814249750933,5.04212575779336,-0.329672438264988));
#13626=CARTESIAN_POINT('Ctrl Pts',(-3.92288158239009,4.12701587633362,-0.237042787193532));
#13627=CARTESIAN_POINT('Ctrl Pts',(-5.41925509595642,1.7467225840705,-0.0980983105863442));
#13628=CARTESIAN_POINT('Ctrl Pts',(-5.59447518483343,-1.05864694079116,
0.0408461660208423));
#13629=CARTESIAN_POINT('Ctrl Pts',(-4.40616613994472,-3.60630744758704,
0.179790642628029));
#13630=CARTESIAN_POINT('Ctrl Pts',(-2.14380698022015,-5.27476971866798,
0.318735119235216));
#13631=CARTESIAN_POINT('Ctrl Pts',(0.641071437260819,-5.65760438869658,
0.457679595842404));
#13632=CARTESIAN_POINT('Ctrl Pts',(3.26970485891195,-4.66136676448167,0.59662407244959));
#13633=CARTESIAN_POINT('Ctrl Pts',(5.10134743403979,-2.52895357103839,0.735568549056777));
#13634=CARTESIAN_POINT('Ctrl Pts',(5.68955167563563,0.219897814119939,0.874513025663964));
#13635=CARTESIAN_POINT('Ctrl Pts',(4.89093832174991,2.91514381174423,1.01345750227115));
#13636=CARTESIAN_POINT('Ctrl Pts',(2.9001705558492,4.89983289385856,1.15240197887834));
#13637=CARTESIAN_POINT('Ctrl Pts',(0.202492121079464,5.690197037745,1.29134645548553));
#13638=CARTESIAN_POINT('Ctrl Pts',(-2.54454306279754,5.09358899509239,1.43029093209272));
#13639=CARTESIAN_POINT('Ctrl Pts',(-4.67135163066769,3.25542950382497,1.5692354086999));
#13640=CARTESIAN_POINT('Ctrl Pts',(-5.65952849672254,0.623766464847588,
1.70817988530709));
#13641=CARTESIAN_POINT('Ctrl Pts',(-5.26820783503249,-2.1599383722897,1.84712436191428));
#13642=CARTESIAN_POINT('Ctrl Pts',(-3.59277314049268,-4.41716295380219,
1.98606883852146));
#13643=CARTESIAN_POINT('Ctrl Pts',(-1.04160794290234,-5.59771385479801,
2.12501331512865));
#13644=CARTESIAN_POINT('Ctrl Pts',(1.76344689301429,-5.41383436293737,2.26395779173584));
#13645=CARTESIAN_POINT('Ctrl Pts',(4.13866544420465,-3.91034471810202,2.40290226834302));
#13646=CARTESIAN_POINT('Ctrl Pts',(5.50509344222147,-1.45371718778633,2.54184674495021));
#13647=CARTESIAN_POINT('Ctrl Pts',(5.52966708099472,1.35725069213826,2.6807912215574));
#13648=CARTESIAN_POINT('Ctrl Pts',(4.20639659128802,3.83739171668186,2.81973569816458));
#13649=CARTESIAN_POINT('Ctrl Pts',(1.85782622968774,5.38217699160281,2.95868017477177));
#13650=CARTESIAN_POINT('Ctrl Pts',(-0.943585168971598,5.61506852126607,
3.09762465137895));
#13651=CARTESIAN_POINT('Ctrl Pts',(-3.51499976833812,4.47929950972323,3.23656912798615));
#13652=CARTESIAN_POINT('Ctrl Pts',(-5.22964094334671,2.25171114333013,3.37551360459333));
#13653=CARTESIAN_POINT('Ctrl Pts',(-5.66956869748686,-0.524726837329223,
3.51445808120052));
#13654=CARTESIAN_POINT('Ctrl Pts',(-4.72755161304236,-3.17326381117624,
3.65340255780771));
#13655=CARTESIAN_POINT('Ctrl Pts',(-2.63320427221665,-5.04832474491386,
3.79234703441489));
#13656=CARTESIAN_POINT('Ctrl Pts',(0.10298078979862,-5.69286768037385,3.93129151102208));
#13657=CARTESIAN_POINT('Ctrl Pts',(2.81406451191796,-4.94978670167555,4.07023598762927));
#13658=CARTESIAN_POINT('Ctrl Pts',(4.83922622917719,-3.00020615494359,4.20918046423645));
#13659=CARTESIAN_POINT('Ctrl Pts',(5.68483724920358,-0.319331989292594,
4.34812494084364));
#13660=CARTESIAN_POINT('Ctrl Pts',(5.1447817549178,2.43937864293008,4.48706941745082));
#13661=CARTESIAN_POINT('Ctrl Pts',(3.35069707936864,4.60349612269073,4.62601389405802));
#13662=CARTESIAN_POINT('Ctrl Pts',(0.739887396760496,5.64552159764121,4.7649583706652));
#13663=CARTESIAN_POINT('Ctrl Pts',(-2.05126820343682,5.31146366144845,4.90390284727239));
#13664=CARTESIAN_POINT('Ctrl Pts',(-4.34243171295922,3.68274819769209,5.04284732387957));
#13665=CARTESIAN_POINT('Ctrl Pts',(-5.57513709051344,1.15637100071714,5.18179180048677));
#13666=CARTESIAN_POINT('Ctrl Pts',(-5.44891512496616,-1.65186907175875,
5.32073627709394));
#13667=CARTESIAN_POINT('Ctrl Pts',(-3.99453214143147,-4.05746970911543,
5.45968075370114));
#13668=CARTESIAN_POINT('Ctrl Pts',(-1.56649077752693,-5.47407107309006,
5.59862523030832));
#13669=CARTESIAN_POINT('Ctrl Pts',(1.24337925098927,-5.55637971232417,5.73756970691551));
#13670=CARTESIAN_POINT('Ctrl Pts',(3.75017833531478,-4.28433307793102,5.8765141835227));
#13671=CARTESIAN_POINT('Ctrl Pts',(5.34287973941681,-1.96798972544256,6.01545866012988));
#13672=CARTESIAN_POINT('Ctrl Pts',(5.63326601638935,0.828046772779887,6.15440313673707));
#13673=CARTESIAN_POINT('Ctrl Pts',(4.55055615306033,3.42224870036692,6.29334761334426));
#13674=CARTESIAN_POINT('Ctrl Pts',(2.3586582855054,5.18228507142697,6.43229208995144));
#13675=CARTESIAN_POINT('Ctrl Pts',(-0.40815732580512,5.67915091071807,6.57123656655863));
#13676=CARTESIAN_POINT('Ctrl Pts',(-3.07548549109974,4.79173626813426,6.71018104316582));
#13677=CARTESIAN_POINT('Ctrl Pts',(-4.99317086567645,2.73634650135507,6.849125519773));
#13678=CARTESIAN_POINT('Ctrl Pts',(-5.69378187813725,0.0139783230101666,
6.9880699963802));
#13679=CARTESIAN_POINT('Ctrl Pts',(-5.00654614275347,-2.71179704067219,
7.12701447298738));
#13680=CARTESIAN_POINT('Ctrl Pts',(-3.0989758510296,-4.77657786956871,7.26595894959457));
#13681=CARTESIAN_POINT('Ctrl Pts',(-0.4360370452756,-5.6770784004156,7.40490342620175));
#13682=CARTESIAN_POINT('Ctrl Pts',(2.33318482649275,-5.19380361919299,7.54384790280894));
#13683=CARTESIAN_POINT('Ctrl Pts',(4.53369805383594,-3.44455068564283,7.68279237941613));
#13684=CARTESIAN_POINT('Ctrl Pts',(5.62913240137773,-0.855696135948733,
7.82173685602332));
#13685=CARTESIAN_POINT('Ctrl Pts',(5.35247816814056,1.9417324555399,7.9606813326305));
#13686=CARTESIAN_POINT('Ctrl Pts',(3.77116921198781,4.26586805279693,8.09962580923769));
#13687=CARTESIAN_POINT('Ctrl Pts',(1.27064609581863,5.55020774102186,8.23857028584488));
#13688=CARTESIAN_POINT('Ctrl Pts',(-1.53959419770053,5.48169655998261,8.37751476245207));
#13689=CARTESIAN_POINT('Ctrl Pts',(-3.9745618084913,4.07703395862735,8.51645923905925));
#13690=CARTESIAN_POINT('Ctrl Pts',(-5.44073876342602,1.67860334131436,8.65540371566644));
#13691=CARTESIAN_POINT('Ctrl Pts',(-5.58074767042653,-1.12898313023138,
8.79434819227362));
#13692=CARTESIAN_POINT('Ctrl Pts',(-4.36046166787279,-3.6613824591717,8.93329266888081));
#13693=CARTESIAN_POINT('Ctrl Pts',(-2.07732277169224,-5.30132790643318,
9.072237145488));
#13694=CARTESIAN_POINT('Ctrl Pts',(0.712158958587137,-5.64908639401295,
9.21118162209519));
#13695=CARTESIAN_POINT('Ctrl Pts',(3.32805351679401,-4.61989255921318,9.35012609870237));
#13696=CARTESIAN_POINT('Ctrl Pts',(5.13274238627044,-2.4646101244418,9.48907057530957));
#13697=CARTESIAN_POINT('Ctrl Pts',(5.68633664398072,0.291415580640832,9.62801505191675));
#13698=CARTESIAN_POINT('Ctrl Pts',(4.85389891321596,2.97640938205737,9.76695952852393));
#13699=CARTESIAN_POINT('Ctrl Pts',(2.83833405091507,4.93590997534744,9.90590400513113));
#13700=CARTESIAN_POINT('Ctrl Pts',(0.130931537266056,5.69229342197565,10.0448484817383));
#13701=CARTESIAN_POINT('Ctrl Pts',(-2.6083852491939,5.06119292865881,10.1837929583455));
#13702=CARTESIAN_POINT('Ctrl Pts',(-4.71191389647006,3.19643784572305,10.3227374349526));
#13703=CARTESIAN_POINT('Ctrl Pts',(-5.66692394621277,0.552558102970641,
10.4616819115598));
#13704=CARTESIAN_POINT('Ctrl Pts',(-5.24063380965353,-2.2260064560631,10.600626388167));
#13705=CARTESIAN_POINT('Ctrl Pts',(-3.53695076535063,-4.46198686156782,
10.7395708647742));
#13706=CARTESIAN_POINT('Ctrl Pts',(-0.971143789706699,-5.61036783188342,
10.8785153413814));
#13707=CARTESIAN_POINT('Ctrl Pts',(1.83137733816162,-5.39123404375903,11.0174598179886));
#13708=CARTESIAN_POINT('Ctrl Pts',(4.18750428774166,-3.85799887369909,11.1564042945958));
#13709=CARTESIAN_POINT('Ctrl Pts',(5.52293632281464,-1.38438500549997,11.295348771203));
#13710=CARTESIAN_POINT('Ctrl Pts',(5.51216483653343,1.42666964788716,11.4342932478101));
#13711=CARTESIAN_POINT('Ctrl Pts',(4.15781535487098,3.88997672796604,11.5732377244173));
#13712=CARTESIAN_POINT('Ctrl Pts',(1.79000757046727,5.40511057860874,11.7121822010245));
#13713=CARTESIAN_POINT('Ctrl Pts',(-1.0141106027887,5.60276067261754,11.8511266776317));
#13714=CARTESIAN_POINT('Ctrl Pts',(-3.57104155810099,4.4347502364433,11.9900711542389));
#13715=CARTESIAN_POINT('Ctrl Pts',(-5.25753902669011,2.18577923225303,12.1290156308461));
#13716=CARTESIAN_POINT('Ctrl Pts',(-5.66252297824849,-0.595970628576718,
12.2679601074533));
#13717=CARTESIAN_POINT('Ctrl Pts',(-4.68727946971874,-3.23245396596321,
12.4069045840605));
#13718=CARTESIAN_POINT('Ctrl Pts',(-2.56952195072682,-5.08103379383087,
12.5458490606676));
#13719=CARTESIAN_POINT('Ctrl Pts',(0.174550864347044,-5.69112286504815,
12.6847935372748));
#13720=CARTESIAN_POINT('Ctrl Pts',(2.87607729204563,-4.91401331698417,12.823738013882));
#13721=CARTESIAN_POINT('Ctrl Pts',(4.87656623679432,-2.93912388433625,12.9626824904892));
#13722=CARTESIAN_POINT('Ctrl Pts',(5.6884029399862,-0.247829501219334,13.1016269670964));
#13723=CARTESIAN_POINT('Ctrl Pts',(5.11370399961879,2.50387277504289,13.2405714437036));
#13724=CARTESIAN_POINT('Ctrl Pts',(3.29255101215109,4.64526159669196,13.3795159203108));
#13725=CARTESIAN_POINT('Ctrl Pts',(0.668845992988569,5.6543781715571,13.518460396918));
#13726=CARTESIAN_POINT('Ctrl Pts',(-2.11788875861632,5.2852525649627,13.6574048735251));
#13727=CARTESIAN_POINT('Ctrl Pts',(-4.38839280647255,3.62785832763879,13.7963493501323));
#13728=CARTESIAN_POINT('Ctrl Pts',(-5.58923580740444,1.08618164159884,13.9352938267395));
#13729=CARTESIAN_POINT('Ctrl Pts',(-5.42771493415498,-1.72024941879635,
14.0742383033467));
#13730=CARTESIAN_POINT('Ctrl Pts',(-3.94320054256959,-4.1073734856228,14.2131827799539));
#13731=CARTESIAN_POINT('Ctrl Pts',(-1.49753973437886,-5.49333434384569,
14.3521272565611));
#13732=CARTESIAN_POINT('Ctrl Pts',(1.31314307405848,-5.54030709765898,14.4910717331683));
#13733=CARTESIAN_POINT('Ctrl Pts',(3.80375016063084,-4.2368422421444,14.6300162097754));
#13734=CARTESIAN_POINT('Ctrl Pts',(5.36720155296861,-1.90065645478859,14.7689606863826));
#13735=CARTESIAN_POINT('Ctrl Pts',(5.62240942988205,0.898810142405872,14.9079051629898));
#13736=CARTESIAN_POINT('Ctrl Pts',(4.50716743545881,3.47919375402662,15.046849639597));
#13737=CARTESIAN_POINT('Ctrl Pts',(2.29331334082306,5.21153157815636,15.1857941162042));
#13738=CARTESIAN_POINT('Ctrl Pts',(-0.479530811733698,5.67357009914538,
15.3247385928114));
#13739=CARTESIAN_POINT('Ctrl Pts',(-3.1354903888362,4.75268844874498,15.4636830694186));
#13740=CARTESIAN_POINT('Ctrl Pts',(-5.02718111402602,2.67334949381821,15.6026275460257));
#13741=CARTESIAN_POINT('Ctrl Pts',(-5.69350755423781,-0.0576124913296487,
15.741572022633));
#13742=CARTESIAN_POINT('Ctrl Pts',(-4.9720541124485,-2.7745315590558,15.8805164992401));
#13743=CARTESIAN_POINT('Ctrl Pts',(-3.03867347046972,-4.81516469180373,
16.0194609758473));
#13744=CARTESIAN_POINT('Ctrl Pts',(-0.364622886433228,-5.68211207386736,
16.1584054524545));
#13745=CARTESIAN_POINT('Ctrl Pts',(2.39830372024077,-5.16405719708987,16.2973499290617));
#13746=CARTESIAN_POINT('Ctrl Pts',(4.57664909608152,-3.38727479261154,16.4362944056689));
#13747=CARTESIAN_POINT('Ctrl Pts',(5.63944637048666,-0.784851644343455,
16.575238882276));
#13748=CARTESIAN_POINT('Ctrl Pts',(5.32764105698159,2.00887735752595,16.7141833588833));
#13749=CARTESIAN_POINT('Ctrl Pts',(3.71723501142589,4.31294694362033,16.8531278354904));
#13750=CARTESIAN_POINT('Ctrl Pts',(1.20076114819234,5.56574524528835,16.9920723120976));
#13751=CARTESIAN_POINT('Ctrl Pts',(-1.60839559119228,5.4619054450054,17.1310167887048));
#13752=CARTESIAN_POINT('Ctrl Pts',(-4.02550945963125,4.02673826565304,17.269961265312));
#13753=CARTESIAN_POINT('Ctrl Pts',(-5.46141429608546,1.61006253293328,17.4089057419192));
#13754=CARTESIAN_POINT('Ctrl Pts',(-5.56611146680997,-1.1990623807166,17.5478502185264));
#13755=CARTESIAN_POINT('Ctrl Pts',(-4.31408127498971,-3.71591849475981,
17.6867946951336));
#13756=CARTESIAN_POINT('Ctrl Pts',(-2.01050329851204,-5.32702767837376,
17.8257391717407));
#13757=CARTESIAN_POINT('Ctrl Pts',(0.78313039494884,-5.63968566053946,17.9646836483479));
#13758=CARTESIAN_POINT('Ctrl Pts',(3.3858778213545,-4.57768268742415,18.1036281249551));
#13759=CARTESIAN_POINT('Ctrl Pts',(5.16332494240252,-2.39987975758783,18.2425726015623));
#13760=CARTESIAN_POINT('Ctrl Pts',(5.68222315902107,0.362888716333284,18.3815170781695));
#13761=CARTESIAN_POINT('Ctrl Pts',(4.81609176954379,3.03720355834013,18.5204615547767));
#13762=CARTESIAN_POINT('Ctrl Pts',(2.77604918718616,4.97120735345811,18.6594060313839));
#13763=CARTESIAN_POINT('Ctrl Pts',(0.0593497091224659,5.69348915185932,
18.7983505079911));
#13764=CARTESIAN_POINT('Ctrl Pts',(-2.6718140835377,5.02799789393279,18.9372949845982));
#13765=CARTESIAN_POINT('Ctrl Pts',(-4.7517331146631,3.13693866919109,19.0762394612054));
#13766=CARTESIAN_POINT('Ctrl Pts',(-5.67341981900402,0.481266594247914,
19.2151839378126));
#13767=CARTESIAN_POINT('Ctrl Pts',(-5.21223845605685,-2.29173084891586,
19.3541284144198));
#13768=CARTESIAN_POINT('Ctrl Pts',(-3.48055511468148,-4.50608921872194,
19.493072891027));
#13769=CARTESIAN_POINT('Ctrl Pts',(-0.900553799180242,-5.6221665142629,
19.6320173676342));
#13770=CARTESIAN_POINT('Ctrl Pts',(1.89907277706644,-5.3677191176857,19.7709618442413));
#13771=CARTESIAN_POINT('Ctrl Pts',(4.23557228367901,-3.8051666205939,19.9099063208486));
#13772=CARTESIAN_POINT('Ctrl Pts',(5.54019395278335,-1.31447358942211,20.0488565944357));
#13773=CARTESIAN_POINT('Ctrl Pts',(5.50876982337505,0.558839851756261,20.1414920424871));
#13774=CARTESIAN_POINT('Ctrl Pts',(5.27006520044008,1.43529986613293,20.1878126650028));
#13775=CARTESIAN_POINT('Ctrl Pts',(-1.32653952126248,4.96194904965828,-0.564094739286002));
#13776=CARTESIAN_POINT('Ctrl Pts',(-2.15165389485,4.74136096719883,-0.517779913750273));
#13777=CARTESIAN_POINT('Ctrl Pts',(-3.68888014840542,3.88083775118329,-0.425150262678815));
#13778=CARTESIAN_POINT('Ctrl Pts',(-5.0959943915612,1.64252989284048,-0.286205786071628));
#13779=CARTESIAN_POINT('Ctrl Pts',(-5.26076253301154,-0.99549823313181,
-0.147261309464441));
#13780=CARTESIAN_POINT('Ctrl Pts',(-4.14333659144391,-3.39118978563335,
-0.00831683285725419));
#13781=CARTESIAN_POINT('Ctrl Pts',(-2.01592804810816,-4.96012762402817,
0.130627643749933));
#13782=CARTESIAN_POINT('Ctrl Pts',(0.602831273122537,-5.32012605495949,
0.269572120357121));
#13783=CARTESIAN_POINT('Ctrl Pts',(3.07466567416403,-4.38331439804939,0.408516596964306));
#13784=CARTESIAN_POINT('Ctrl Pts',(4.79705004709394,-2.37810049284196,0.547461073571495));
#13785=CARTESIAN_POINT('Ctrl Pts',(5.35016767362928,0.20678082275697,0.686405550178681));
#13786=CARTESIAN_POINT('Ctrl Pts',(4.59919192135954,2.74125433333585,0.825350026785868));
#13787=CARTESIAN_POINT('Ctrl Pts',(2.72717423806198,4.60755592873295,0.964294503393056));
#13788=CARTESIAN_POINT('Ctrl Pts',(0.190413386172985,5.35077453963423,1.10323898000024));
#13789=CARTESIAN_POINT('Ctrl Pts',(-2.39276006526755,4.78975440209051,1.24218345660743));
#13790=CARTESIAN_POINT('Ctrl Pts',(-4.39270366302834,3.06124184963968,1.38112793321462));
#13791=CARTESIAN_POINT('Ctrl Pts',(-5.32193538918262,0.586558549140649,
1.5200724098218));
#13792=CARTESIAN_POINT('Ctrl Pts',(-4.95395715934022,-2.03109719627685,
1.65901688642899));
#13793=CARTESIAN_POINT('Ctrl Pts',(-3.37846280529652,-4.15367744101648,
1.79796136303618));
#13794=CARTESIAN_POINT('Ctrl Pts',(-0.979475618189015,-5.26380801503507,
1.93690583964336));
#13795=CARTESIAN_POINT('Ctrl Pts',(1.65825659015796,-5.09089700740523,2.07585031625056));
#13796=CARTESIAN_POINT('Ctrl Pts',(3.89179241773501,-3.67709111301799,2.21479479285774));
#13797=CARTESIAN_POINT('Ctrl Pts',(5.1767124466079,-1.36700238403667,2.35373926946493));
#13798=CARTESIAN_POINT('Ctrl Pts',(5.19982025813391,1.27629015291048,2.49268374607211));
#13799=CARTESIAN_POINT('Ctrl Pts',(3.9554833751746,3.60848978691285,2.6316282226793));
#13800=CARTESIAN_POINT('Ctrl Pts',(1.74700616216575,5.06112801075975,2.77057269928649));
#13801=CARTESIAN_POINT('Ctrl Pts',(-0.887299941393687,5.28012746880181,
2.90951717589367));
#13802=CARTESIAN_POINT('Ctrl Pts',(-3.30532864547293,4.21210752686368,3.04846165250086));
#13803=CARTESIAN_POINT('Ctrl Pts',(-4.91769079795831,2.11739568531994,3.18740612910805));
#13804=CARTESIAN_POINT('Ctrl Pts',(-5.33137668801045,-0.49342667447535,
3.32635060571523));
#13805=CARTESIAN_POINT('Ctrl Pts',(-4.44555129428321,-2.98397737297218,
3.46529508232243));
#13806=CARTESIAN_POINT('Ctrl Pts',(-2.47613259856755,-4.74719018229208,
3.60423955892961));
#13807=CARTESIAN_POINT('Ctrl Pts',(0.0968379450607276,-5.35328587737668,
3.7431840355368));
#13808=CARTESIAN_POINT('Ctrl Pts',(2.64620445362047,-4.65452997220665,3.88212851214398));
#13809=CARTESIAN_POINT('Ctrl Pts',(4.55056447550943,-2.82124267420587,4.02107298875117));
#13810=CARTESIAN_POINT('Ctrl Pts',(5.34573446459376,-0.30028371015333,4.16001746535835));
#13811=CARTESIAN_POINT('Ctrl Pts',(4.83789349359654,2.29386874453304,4.29896194196555));
#13812=CARTESIAN_POINT('Ctrl Pts',(3.15082667671865,4.32889576287152,4.43790641857272));
#13813=CARTESIAN_POINT('Ctrl Pts',(0.695752821654702,5.30876400715728,4.57685089517993));
#13814=CARTESIAN_POINT('Ctrl Pts',(-1.92890924586693,4.99463275864584,4.7157953717871));
#13815=CARTESIAN_POINT('Ctrl Pts',(-4.08340394817162,3.4630708148384,4.8547398483943));
#13816=CARTESIAN_POINT('Ctrl Pts',(-5.2425779636467,1.08739301433061,4.99368432500148));
#13817=CARTESIAN_POINT('Ctrl Pts',(-5.1238851881395,-1.55333442995828,5.13262880160866));
#13818=CARTESIAN_POINT('Ctrl Pts',(-3.7562567233335,-3.81544004027595,5.27157327821586));
#13819=CARTESIAN_POINT('Ctrl Pts',(-1.47304898465952,-5.14754057403365,
5.41051775482304));
#13820=CARTESIAN_POINT('Ctrl Pts',(1.16921118814885,-5.2249394704663,5.54946223143023));
#13821=CARTESIAN_POINT('Ctrl Pts',(3.5264787181504,-4.02877091964304,5.68840670803742));
#13822=CARTESIAN_POINT('Ctrl Pts',(5.0241748551696,-1.85059836193878,5.8273511846446));
#13823=CARTESIAN_POINT('Ctrl Pts',(5.29723947616198,0.778653456115254,5.96629566125179));
#13824=CARTESIAN_POINT('Ctrl Pts',(4.27911368331464,3.21811021529694,6.10524013785897));
#13825=CARTESIAN_POINT('Ctrl Pts',(2.2179633882733,4.87315972248072,6.24418461446617));
#13826=CARTESIAN_POINT('Ctrl Pts',(-0.383810580300875,5.34038731844219,
6.38312909107335));
#13827=CARTESIAN_POINT('Ctrl Pts',(-2.89203156826225,4.50590730937773,6.52207356768053));
#13828=CARTESIAN_POINT('Ctrl Pts',(-4.69532625370965,2.57312235304776,6.66101804428772));
#13829=CARTESIAN_POINT('Ctrl Pts',(-5.35414554288283,0.0131445105281004,
6.79996252089491));
#13830=CARTESIAN_POINT('Ctrl Pts',(-4.70790369023241,-2.55003727737951,
6.9389069975021));
#13831=CARTESIAN_POINT('Ctrl Pts',(-2.91412071895525,-4.49165311526668,
7.07785147410929));
#13832=CARTESIAN_POINT('Ctrl Pts',(-0.410027263506262,-5.3384384341969,
7.21679595071647));
#13833=CARTESIAN_POINT('Ctrl Pts',(2.19400943114016,-4.88399118432835,7.35574042732366));
#13834=CARTESIAN_POINT('Ctrl Pts',(4.26326117635958,-3.23908187835291,7.49468490393085));
#13835=CARTESIAN_POINT('Ctrl Pts',(5.29335243291654,-0.804653523863272,
7.63362938053803));
#13836=CARTESIAN_POINT('Ctrl Pts',(5.03320073383335,1.82590734854443,7.77257385714523));
#13837=CARTESIAN_POINT('Ctrl Pts',(3.54621748074888,4.01140734054273,7.9115183337524));
#13838=CARTESIAN_POINT('Ctrl Pts',(1.19485155492724,5.21913565968705,8.0504628103596));
#13839=CARTESIAN_POINT('Ctrl Pts',(-1.4477567964306,5.15471119762476,8.18940728696677));
#13840=CARTESIAN_POINT('Ctrl Pts',(-3.7374776286316,3.83383727458631,8.32835176357398));
#13841=CARTESIAN_POINT('Ctrl Pts',(-5.11619654979082,1.57847398978809,8.46729624018115));
#13842=CARTESIAN_POINT('Ctrl Pts',(-5.24785387025458,-1.06163884112396,
8.60624071678835));
#13843=CARTESIAN_POINT('Ctrl Pts',(-4.1003584091617,-3.44297955104964,8.74518519339552));
#13844=CARTESIAN_POINT('Ctrl Pts',(-1.95340964884727,-4.98510160541583,
8.88412967000273));
#13845=CARTESIAN_POINT('Ctrl Pts',(0.669678395757383,-5.31211616201914,
9.0230741466099));
#13846=CARTESIAN_POINT('Ctrl Pts',(3.1295338115846,-4.34431414548693,9.16201862321709));
#13847=CARTESIAN_POINT('Ctrl Pts',(4.82657227803858,-2.31759515821866,9.30096309982428));
#13848=CARTESIAN_POINT('Ctrl Pts',(5.34714441988092,0.274032526290802,9.43990757643146));
#13849=CARTESIAN_POINT('Ctrl Pts',(4.56436192815685,2.79886538821026,9.57885205303865));
#13850=CARTESIAN_POINT('Ctrl Pts',(2.66902630504195,4.64148099807844,9.71779652964585));
#13851=CARTESIAN_POINT('Ctrl Pts',(0.123121419415037,5.35274587371849,9.85674100625302));
#13852=CARTESIAN_POINT('Ctrl Pts',(-2.45279404005934,4.75929077380007,9.99568548286022));
#13853=CARTESIAN_POINT('Ctrl Pts',(-4.4308463736736,3.00576906721603,10.1346299594674));
#13854=CARTESIAN_POINT('Ctrl Pts',(-5.32888969719323,0.519597794141693,
10.2735744360746));
#13855=CARTESIAN_POINT('Ctrl Pts',(-4.92802793545319,-2.09322429278901,
10.4125189126818));
#13856=CARTESIAN_POINT('Ctrl Pts',(-3.32597025685388,-4.19582758500065,
10.551463389289));
#13857=CARTESIAN_POINT('Ctrl Pts',(-0.913214679529933,-5.27570717739528,
10.6904078658962));
#13858=CARTESIAN_POINT('Ctrl Pts',(1.72213495745338,-5.0696448061818,10.8293523425034));
#13859=CARTESIAN_POINT('Ctrl Pts',(3.93771800498789,-3.62786771888437,10.9682968191105));
#13860=CARTESIAN_POINT('Ctrl Pts',(5.19349099233457,-1.30180589377555,11.1072412957177));
#13861=CARTESIAN_POINT('Ctrl Pts',(5.18336202945946,1.34156824056286,11.2461857723249));
#13862=CARTESIAN_POINT('Ctrl Pts',(3.90980002867536,3.65793808152889,11.3851302489321));
#13863=CARTESIAN_POINT('Ctrl Pts',(1.68323291272256,5.08269360025337,11.5240747255393));
#13864=CARTESIAN_POINT('Ctrl Pts',(-0.953618505260992,5.26855378818066,
11.6630192021465));
#13865=CARTESIAN_POINT('Ctrl Pts',(-3.3580275203677,4.17021563530979,11.8019636787537));
#13866=CARTESIAN_POINT('Ctrl Pts',(-4.94392474962437,2.05539663874902,11.9409081553609));
#13867=CARTESIAN_POINT('Ctrl Pts',(-5.32475124870422,-0.560420745468919,
12.079852631968));
#13868=CARTESIAN_POINT('Ctrl Pts',(-4.40768140019639,-3.03963681167534,
12.2187971085752));
#13869=CARTESIAN_POINT('Ctrl Pts',(-2.41624895267756,-4.77794812353731,
12.3577415851824));
#13870=CARTESIAN_POINT('Ctrl Pts',(0.164138836427611,-5.35164514097351,
12.4966860617896));
#13871=CARTESIAN_POINT('Ctrl Pts',(2.70451814694919,-4.62089048402487,12.6356305383968));
#13872=CARTESIAN_POINT('Ctrl Pts',(4.58567713694141,-2.76380398513751,12.774575015004));
#13873=CARTESIAN_POINT('Ctrl Pts',(5.34908746051452,-0.233046373701707,
12.9135194916112));
#13874=CARTESIAN_POINT('Ctrl Pts',(4.80866953866144,2.35451577622209,13.0524639682184));
#13875=CARTESIAN_POINT('Ctrl Pts',(3.09614904534953,4.36816990987189,13.1914084448255));
#13876=CARTESIAN_POINT('Ctrl Pts',(0.628949065643935,5.31709228294514,13.3303529214327));
#13877=CARTESIAN_POINT('Ctrl Pts',(-1.99155585864786,4.96998516440586,13.4692973980399));
#13878=CARTESIAN_POINT('Ctrl Pts',(-4.12662344432501,3.41145514718809,13.6082418746471));
#13879=CARTESIAN_POINT('Ctrl Pts',(-5.25583568651315,1.02139047817374,13.7471863512543));
#13880=CARTESIAN_POINT('Ctrl Pts',(-5.10394959707376,-1.61763586231873,
13.8861308278615));
#13881=CARTESIAN_POINT('Ctrl Pts',(-3.70798707459429,-3.86236703682739,
14.0250753044687));
#13882=CARTESIAN_POINT('Ctrl Pts',(-1.40821089843674,-5.16565478308926,
14.1640197810758));
#13883=CARTESIAN_POINT('Ctrl Pts',(1.23481357164983,-5.20982559360661,14.302964257683));
#13884=CARTESIAN_POINT('Ctrl Pts',(3.57685496295202,-3.98411293094645,14.4419087342902));
#13885=CARTESIAN_POINT('Ctrl Pts',(5.04704586294798,-1.7872815474426,14.5808532108974));
#13886=CARTESIAN_POINT('Ctrl Pts',(5.28703048932282,0.845195762826563,14.7197976875046));
#13887=CARTESIAN_POINT('Ctrl Pts',(4.2383131198351,3.27165847404077,14.8587421641118));
#13888=CARTESIAN_POINT('Ctrl Pts',(2.15651629532014,4.9006616635458,14.997686640719));
#13889=CARTESIAN_POINT('Ctrl Pts',(-0.450926609636636,5.33513940448148,
15.1366311173262));
#13890=CARTESIAN_POINT('Ctrl Pts',(-2.94845715017653,4.46918870781955,15.2755755939333));
#13891=CARTESIAN_POINT('Ctrl Pts',(-4.72730777732795,2.5138831418631,15.4145200705406));
#13892=CARTESIAN_POINT('Ctrl Pts',(-5.35388758251222,-0.054175883493441,
15.5534645471477));
#13893=CARTESIAN_POINT('Ctrl Pts',(-4.67546912314239,-2.60902965699247,
15.6924090237549));
#13894=CARTESIAN_POINT('Ctrl Pts',(-2.85741539918533,-4.52793821833268,
15.8313535003621));
#13895=CARTESIAN_POINT('Ctrl Pts',(-0.342872987412053,-5.34317184704143,
15.9702979769693));
#13896=CARTESIAN_POINT('Ctrl Pts',(2.25524395718639,-4.85601914803879,16.1092424535765));
#13897=CARTESIAN_POINT('Ctrl Pts',(4.30365017199082,-3.18522251493655,16.2481869301836));
#13898=CARTESIAN_POINT('Ctrl Pts',(5.30305116969921,-0.73803493413073,16.3871314067908));
#13899=CARTESIAN_POINT('Ctrl Pts',(5.00984516615337,1.88904703063804,16.526075883398));
#13900=CARTESIAN_POINT('Ctrl Pts',(3.49550047652777,4.05567795695568,16.6650203600052));
#13901=CARTESIAN_POINT('Ctrl Pts',(1.12913527199678,5.23374634569442,16.8039648366124));
#13902=CARTESIAN_POINT('Ctrl Pts',(-1.51245415965809,5.13610063046365,16.9429093132196));
#13903=CARTESIAN_POINT('Ctrl Pts',(-3.78538623228198,3.78654173953978,17.0818537898268));
#13904=CARTESIAN_POINT('Ctrl Pts',(-5.13563877877053,1.51402166766663,17.220798266434));
#13905=CARTESIAN_POINT('Ctrl Pts',(-5.23409072195781,-1.12753783667114,
17.3597427430411));
#13906=CARTESIAN_POINT('Ctrl Pts',(-4.05674462501138,-3.4942624906002,17.4986872196483));
#13907=CARTESIAN_POINT('Ctrl Pts',(-1.89057598360286,-5.00926837582149,
17.6376316962555));
#13908=CARTESIAN_POINT('Ctrl Pts',(0.736416357941547,-5.30327618600596,
17.7765761728627));
#13909=CARTESIAN_POINT('Ctrl Pts',(3.18390887356609,-4.3046221092021,17.9155206494699));
#13910=CARTESIAN_POINT('Ctrl Pts',(4.85533057263242,-2.25672598328394,18.0544651260771));
#13911=CARTESIAN_POINT('Ctrl Pts',(5.3432763059219,0.341242261242714,18.1934096026843));
#13912=CARTESIAN_POINT('Ctrl Pts',(4.52880999551982,2.85603316789416,18.3323540792915));
#13913=CARTESIAN_POINT('Ctrl Pts',(2.61045675800614,4.67467287365983,18.4712985558986));
#13914=CARTESIAN_POINT('Ctrl Pts',(0.0558094755595731,5.35387027784286,
18.6102430325058));
#13915=CARTESIAN_POINT('Ctrl Pts',(-2.51243931941155,4.72807583599107,18.749187509113));
#13916=CARTESIAN_POINT('Ctrl Pts',(-4.46829035979255,2.9498190400369,18.8881319857202));
#13917=CARTESIAN_POINT('Ctrl Pts',(-5.33499808860984,0.452558852039112,
19.0270764623274));
#13918=CARTESIAN_POINT('Ctrl Pts',(-4.90132637590066,-2.15502819967951,
19.1660209389346));
#13919=CARTESIAN_POINT('Ctrl Pts',(-3.27293862899549,-4.23729921915194,
19.3049654155417));
#13920=CARTESIAN_POINT('Ctrl Pts',(-0.846835409786463,-5.28680206371619,
19.443909892149));
#13921=CARTESIAN_POINT('Ctrl Pts',(1.78579233672135,-5.0475325547255,19.5828543687561));
#13922=CARTESIAN_POINT('Ctrl Pts',(3.98291872600452,-3.57818693051949,19.7217988453633));
#13923=CARTESIAN_POINT('Ctrl Pts',(5.20971919786745,-1.23606472124711,19.8607491189504));
#13924=CARTESIAN_POINT('Ctrl Pts',(5.18016953017532,0.525504834134071,19.9533845670019));
#13925=CARTESIAN_POINT('Ctrl Pts',(4.95570373216851,1.3496836628856,19.9997051895175));
#13926=CARTESIAN_POINT('Ctrl Pts',(4.95630975100502,1.34951628911715,20.));
#13927=CARTESIAN_POINT('Ctrl Pts',(5.00802755365851,1.211898038485,20.));
#13928=CARTESIAN_POINT('Ctrl Pts',(5.05359491432269,1.07229989795897,20.));
#13929=CARTESIAN_POINT('Ctrl Pts',(5.09309141450286,0.931165512631317,20.));
#13930=CARTESIAN_POINT('Ctrl Pts',(5.13361484558061,0.786361555054366,20.));
#13931=CARTESIAN_POINT('Ctrl Pts',(5.16774795161437,0.639939896759643,20.));
#13932=CARTESIAN_POINT('Ctrl Pts',(5.1955341576068,0.492345209748209,20.));
#13933=CARTESIAN_POINT('Ctrl Pts',(5.22356749502463,0.343437810760418,20.));
#13934=CARTESIAN_POINT('Ctrl Pts',(5.24514076865378,0.193335729449919,20.));
#13935=CARTESIAN_POINT('Ctrl Pts',(5.26025167875134,0.0424704475167592,
20.));
#13936=CARTESIAN_POINT('Ctrl Pts',(5.27537595868635,-0.108528317064509,
20.));
#13937=CARTESIAN_POINT('Ctrl Pts',(5.28402662307941,-0.260292389709474,
20.));
#13938=CARTESIAN_POINT('Ctrl Pts',(5.28615148445568,-0.412403260215922,
20.));
#13939=CARTESIAN_POINT('Ctrl Pts',(5.28676690382088,-0.456458828457367,
20.));
#13940=CARTESIAN_POINT('Ctrl Pts',(5.28683458090809,-0.500543537596189,
20.));
#13941=CARTESIAN_POINT('Ctrl Pts',(5.2863524316627,-0.544647299363032,20.));
#13942=CARTESIAN_POINT('Ctrl Pts',(5.28606370890326,-0.571057710498386,
20.));
#13943=CARTESIAN_POINT('Ctrl Pts',(5.28557781638241,-0.597474953969446,
20.));
#13944=CARTESIAN_POINT('Ctrl Pts',(5.28489424200912,-0.62389686300013,20.));
#13945=CARTESIAN_POINT('Ctrl Pts',(5.2843968262318,-0.643123263128963,20.));
#13946=CARTESIAN_POINT('Ctrl Pts',(5.28379474164197,-0.662350293752617,
20.));
#13947=CARTESIAN_POINT('Ctrl Pts',(5.28308839198291,-0.681565428488897,
20.));
#13948=CARTESIAN_POINT('Ctrl Pts',(5.27736618453607,-0.837229108183571,
20.));
#13949=CARTESIAN_POINT('Ctrl Pts',(5.26480020104454,-0.9923217207242,20.));
#13950=CARTESIAN_POINT('Ctrl Pts',(5.2454298214747,-1.14638516961014,20.));
#13951=CARTESIAN_POINT('Ctrl Pts',(5.24142362338621,-1.17824870084388,20.));
#13952=CARTESIAN_POINT('Ctrl Pts',(5.23712620434838,-1.21006827943255,20.));
#13953=CARTESIAN_POINT('Ctrl Pts',(5.23253765420047,-1.24183995038678,20.));
#13954=CARTESIAN_POINT('Ctrl Pts',(5.21056598904419,-1.39397439223904,20.));
#13955=CARTESIAN_POINT('Ctrl Pts',(5.18192339605888,-1.54500983747171,20.));
#13956=CARTESIAN_POINT('Ctrl Pts',(5.14686314689944,-1.69457665028804,20.));
#13957=CARTESIAN_POINT('Ctrl Pts',(5.11144700718872,-1.84566169006348,20.));
#13958=CARTESIAN_POINT('Ctrl Pts',(5.0694821499338,-1.99524882750055,20.));
#13959=CARTESIAN_POINT('Ctrl Pts',(5.02117633579842,-2.14295818514512,20.));
#13960=CARTESIAN_POINT('Ctrl Pts',(4.97269078910331,-2.29121712841247,20.));
#13961=CARTESIAN_POINT('Ctrl Pts',(4.91781683973363,-2.43758503571107,20.));
#13962=CARTESIAN_POINT('Ctrl Pts',(4.85671337014158,-2.58166803167885,20.));
#13963=CARTESIAN_POINT('Ctrl Pts',(4.84567119665135,-2.60770566013255,20.));
#13964=CARTESIAN_POINT('Ctrl Pts',(4.83442545485886,-2.63366862717467,20.));
#13965=CARTESIAN_POINT('Ctrl Pts',(4.82297691173008,-2.65955454483019,20.));
#13966=CARTESIAN_POINT('Ctrl Pts',(4.81504490372224,-2.6774893426315,20.));
#13967=CARTESIAN_POINT('Ctrl Pts',(4.807016416577,-2.69538508390504,20.));
#13968=CARTESIAN_POINT('Ctrl Pts',(4.79889653142679,-2.71323079035806,20.));
#13969=CARTESIAN_POINT('Ctrl Pts',(4.73305025549089,-2.85794629921556,20.));
#13970=CARTESIAN_POINT('Ctrl Pts',(4.66111448930543,-2.99956115386831,20.));
#13971=CARTESIAN_POINT('Ctrl Pts',(4.58336053077309,-3.1376925483382,20.));
#13972=CARTESIAN_POINT('Ctrl Pts',(4.50473495546917,-3.27737238667349,20.));
#13973=CARTESIAN_POINT('Ctrl Pts',(4.4201598678686,-3.4134909783492,20.));
#13974=CARTESIAN_POINT('Ctrl Pts',(4.32986292961299,-3.54564765538286,20.));
#13975=CARTESIAN_POINT('Ctrl Pts',(4.28143800460734,-3.61652134498943,20.));
#13976=CARTESIAN_POINT('Ctrl Pts',(4.23136657861736,-3.68625543000986,20.));
#13977=CARTESIAN_POINT('Ctrl Pts',(4.17967784234231,-3.75478638155876,20.));
#13978=CARTESIAN_POINT('Ctrl Pts',(4.08363909948493,-3.88211830932257,20.));
#13979=CARTESIAN_POINT('Ctrl Pts',(3.98201968089173,-4.00529850891546,20.));
#13980=CARTESIAN_POINT('Ctrl Pts',(3.87518106995263,-4.12409405024153,20.));
#13981=CARTESIAN_POINT('Ctrl Pts',(3.7790674283499,-4.23096432853,20.));
#13982=CARTESIAN_POINT('Ctrl Pts',(3.67872896688893,-4.33428603353984,20.));
#13983=CARTESIAN_POINT('Ctrl Pts',(3.57440019418943,-4.43386776444262,20.));
#13984=CARTESIAN_POINT('Ctrl Pts',(3.55912119418721,-4.44845155784223,20.));
#13985=CARTESIAN_POINT('Ctrl Pts',(3.54376310959292,-4.46294883322329,20.));
#13986=CARTESIAN_POINT('Ctrl Pts',(3.52832963421354,-4.47735661404417,20.));
#13987=CARTESIAN_POINT('Ctrl Pts',(3.40931164145479,-4.58846478062726,20.));
#13988=CARTESIAN_POINT('Ctrl Pts',(3.28576263570275,-4.69430173361665,20.));
#13989=CARTESIAN_POINT('Ctrl Pts',(3.15811578368783,-4.7946678411415,20.));
#13990=CARTESIAN_POINT('Ctrl Pts',(3.02925981578756,-4.89598465174318,20.));
#13991=CARTESIAN_POINT('Ctrl Pts',(2.89622752993871,-4.99172703492966,20.));
#13992=CARTESIAN_POINT('Ctrl Pts',(2.75941743654065,-5.08166364708008,20.));
#13993=CARTESIAN_POINT('Ctrl Pts',(2.62247809700501,-5.1716852234277,20.));
#13994=CARTESIAN_POINT('Ctrl Pts',(2.48175325925716,-5.25589059093984,20.));
#13995=CARTESIAN_POINT('Ctrl Pts',(2.33760340461929,-5.33401368905513,20.));
#13996=CARTESIAN_POINT('Ctrl Pts',(2.21232042361525,-5.40191174307497,20.));
#13997=CARTESIAN_POINT('Ctrl Pts',(2.08444948553081,-5.46521516943517,20.));
#13998=CARTESIAN_POINT('Ctrl Pts',(1.95420814809202,-5.52372361795384,20.));
#13999=CARTESIAN_POINT('Ctrl Pts',(1.89742161393368,-5.54923389046558,20.));
#14000=CARTESIAN_POINT('Ctrl Pts',(1.84018425350229,-5.57383227726414,20.));
#14001=CARTESIAN_POINT('Ctrl Pts',(1.78251853632916,-5.59751523771367,20.));
#14002=CARTESIAN_POINT('Ctrl Pts',(1.75691956432136,-5.60802858032569,20.));
#14003=CARTESIAN_POINT('Ctrl Pts',(1.73123617245675,-5.6183615112354,20.));
#14004=CARTESIAN_POINT('Ctrl Pts',(1.70547030102192,-5.62851365711605,20.));
#14005=CARTESIAN_POINT('Ctrl Pts',(1.68482728538373,-5.63664731976764,20.));
#14006=CARTESIAN_POINT('Ctrl Pts',(1.66413268935087,-5.64466435227788,20.));
#14007=CARTESIAN_POINT('Ctrl Pts',(1.64339888368342,-5.65256041345011,20.));
#14008=CARTESIAN_POINT('Ctrl Pts',(1.4887528735376,-5.71145429794664,20.));
#14009=CARTESIAN_POINT('Ctrl Pts',(1.33175860111718,-5.76368915521618,20.));
#14010=CARTESIAN_POINT('Ctrl Pts',(1.17288405441337,-5.80928192680759,20.));
#14011=CARTESIAN_POINT('Ctrl Pts',(1.0117104916612,-5.85553445489085,20.));
#14012=CARTESIAN_POINT('Ctrl Pts',(0.848601209939264,-5.89495157525683,
20.));
#14013=CARTESIAN_POINT('Ctrl Pts',(0.684016067746065,-5.92750558887808,
20.));
#14014=CARTESIAN_POINT('Ctrl Pts',(0.561129089048119,-5.95181194074616,
20.));
#14015=CARTESIAN_POINT('Ctrl Pts',(0.437418685281485,-5.97229131717515,
20.));
#14016=CARTESIAN_POINT('Ctrl Pts',(0.313069360631807,-5.98891456741767,
20.));
#14017=CARTESIAN_POINT('Ctrl Pts',(0.286181878098548,-5.99250893636018,
20.));
#14018=CARTESIAN_POINT('Ctrl Pts',(0.259274152325606,-5.99592166155524,
20.));
#14019=CARTESIAN_POINT('Ctrl Pts',(0.232350196748965,-5.99915251615709,
20.));
#14020=CARTESIAN_POINT('Ctrl Pts',(0.0633272905923215,-6.01943513891737,
20.));
#14021=CARTESIAN_POINT('Ctrl Pts',(-0.106359787945285,-6.03255750685238,
20.));
#14022=CARTESIAN_POINT('Ctrl Pts',(-0.276237342802518,-6.03850393719931,
20.));
#14023=CARTESIAN_POINT('Ctrl Pts',(-0.446444855390507,-6.04446191745738,
20.));
#14024=CARTESIAN_POINT('Ctrl Pts',(-0.61684432643634,-6.04321626583662,
20.));
#14025=CARTESIAN_POINT('Ctrl Pts',(-0.786975461233458,-6.03470182931886,
20.));
#14026=CARTESIAN_POINT('Ctrl Pts',(-0.846277277337399,-6.03173399189624,
20.));
#14027=CARTESIAN_POINT('Ctrl Pts',(-0.90554658260626,-6.02788255987274,
20.));
#14028=CARTESIAN_POINT('Ctrl Pts',(-0.964764086495351,-6.02314329455464,
20.));
#14029=CARTESIAN_POINT('Ctrl Pts',(-1.02320302808891,-6.01846633874036,
20.));
#14030=CARTESIAN_POINT('Ctrl Pts',(-1.08159152517642,-6.01292474055862,
20.));
#14031=CARTESIAN_POINT('Ctrl Pts',(-1.13991297760764,-6.00652560023185,
20.));
#14032=CARTESIAN_POINT('',(-3.88011837732335,-3.36643235951024,-0.00012510356376383));
#14033=CARTESIAN_POINT('Ctrl Pts',(-3.87712761685009,-3.36958187393604,
0.));
#14034=CARTESIAN_POINT('Ctrl Pts',(-3.87807635419917,-3.36849023232742,
-4.17011879212766E-5));
#14035=CARTESIAN_POINT('Ctrl Pts',(-3.87902463050534,-3.36739819002994,
-8.34023758425532E-5));
#14036=CARTESIAN_POINT('Ctrl Pts',(-3.87997244543031,-3.36630574743317,
-0.00012510356376383));
#14037=CARTESIAN_POINT('Ctrl Pts',(-1.5788818818754,5.90584097022478,2.71050543121376E-20));
#14038=CARTESIAN_POINT('Ctrl Pts',(-1.73738372178013,5.84977611874637,1.41954999535879E-15));
#14039=CARTESIAN_POINT('Ctrl Pts',(-1.89317454668904,5.78715364031114,-1.62634446731416E-15));
#14040=CARTESIAN_POINT('Ctrl Pts',(-2.04591809998494,5.71826166590681,-1.90819582357449E-15));
#14041=CARTESIAN_POINT('Ctrl Pts',(-2.20036694327166,5.6486005540046,-2.19319388086643E-15));
#14042=CARTESIAN_POINT('Ctrl Pts',(-2.35170073198387,5.57252876729252,-1.64505916368078E-15));
#14043=CARTESIAN_POINT('Ctrl Pts',(-2.49954705832695,5.49029744531603,-2.67841304690819E-15));
#14044=CARTESIAN_POINT('Ctrl Pts',(-2.64691768285296,5.40833070610091,-3.70844207024844E-15));
#14045=CARTESIAN_POINT('Ctrl Pts',(-2.79082382020564,5.32024350753178,-1.82369499736428E-15));
#14046=CARTESIAN_POINT('Ctrl Pts',(-2.93086319241294,5.22624534364585,9.71445146547012E-17));
#14047=CARTESIAN_POINT('Ctrl Pts',(-3.06866119336755,5.13375164796069,1.98724042653163E-15));
#14048=CARTESIAN_POINT('Ctrl Pts',(-3.20271565751252,5.03553416804527,6.50016582170925E-16));
#14049=CARTESIAN_POINT('Ctrl Pts',(-3.33260352332624,4.93176207959357,1.49880108324396E-15));
#14050=CARTESIAN_POINT('Ctrl Pts',(-3.39649124541486,4.88071988018546,1.9162912620067E-15));
#14051=CARTESIAN_POINT('Ctrl Pts',(-3.45937026984301,4.82833340907307,1.89993404248056E-15));
#14052=CARTESIAN_POINT('Ctrl Pts',(-3.52118613976384,4.77462059891634,1.4432899320127E-15));
#14053=CARTESIAN_POINT('Ctrl Pts',(-3.5392354254394,4.7589372823797,1.30251253808548E-15));
#14054=CARTESIAN_POINT('Ctrl Pts',(-3.55719405290947,4.74314088034149,2.3520270366554E-16));
#14055=CARTESIAN_POINT('Ctrl Pts',(-3.57506061886072,4.72723181907044,1.62370117351429E-15));
#14056=CARTESIAN_POINT('Ctrl Pts',(-3.5909387783033,4.71309330962589,3.67955640940023E-15));
#14057=CARTESIAN_POINT('Ctrl Pts',(-3.60673813814453,4.69887122125484,1.47731149873469E-15));
#14058=CARTESIAN_POINT('Ctrl Pts',(-3.62245453970707,4.68456914621453,1.67921232474555E-15));
#14059=CARTESIAN_POINT('Ctrl Pts',(-3.74459274110421,4.57342222020102,2.48255805465195E-15));
#14060=CARTESIAN_POINT('Ctrl Pts',(-3.86179045770333,4.45738819529234,1.89396572533195E-15));
#14061=CARTESIAN_POINT('Ctrl Pts',(-3.97369545139774,4.33669080159381,3.10862446895044E-15));
#14062=CARTESIAN_POINT('Ctrl Pts',(-3.99821750982727,4.31024203963195,3.70849224798273E-15));
#14063=CARTESIAN_POINT('Ctrl Pts',(-4.02248527033337,4.28356921164166,2.25584676567993E-15));
#14064=CARTESIAN_POINT('Ctrl Pts',(-4.04649477136385,4.25667445357649,2.24820162486594E-15));
#14065=CARTESIAN_POINT('Ctrl Pts',(-4.15647220143564,4.13348087405744,2.10178287836601E-15));
#14066=CARTESIAN_POINT('Ctrl Pts',(-4.26103452091919,4.00563289035671,3.48538070402028E-16));
#14067=CARTESIAN_POINT('Ctrl Pts',(-4.35997112081345,3.87353532936375,1.69309011255336E-15));
#14068=CARTESIAN_POINT('Ctrl Pts',(-4.45871887377264,3.74168991186016,1.25126370824338E-15));
#14069=CARTESIAN_POINT('Ctrl Pts',(-4.55186264529244,3.60561039414627,1.98141016501602E-15));
#14070=CARTESIAN_POINT('Ctrl Pts',(-4.63914521870387,3.46567967142402,2.08166817117217E-15));
#14071=CARTESIAN_POINT('Ctrl Pts',(-4.72248228550573,3.33207435330206,3.79683147803274E-15));
#14072=CARTESIAN_POINT('Ctrl Pts',(-4.80047597977778,3.19495747398172,2.49449903000048E-16));
#14073=CARTESIAN_POINT('Ctrl Pts',(-4.8728580206208,3.05465465625189,2.80331313717852E-15));
#14074=CARTESIAN_POINT('Ctrl Pts',(-4.8935934643793,3.01446179691395,2.71989202312118E-15));
#14075=CARTESIAN_POINT('Ctrl Pts',(-4.91386809532294,2.9740074624354,-1.98418256427254E-15));
#14076=CARTESIAN_POINT('Ctrl Pts',(-4.93367490701556,2.93329929699418,-7.49400541621981E-16));
#14077=CARTESIAN_POINT('Ctrl Pts',(-4.95079469490032,2.89811366649765,9.45444324111637E-16));
#14078=CARTESIAN_POINT('Ctrl Pts',(-4.96755007806123,2.86276890738097,7.94867220024555E-16));
#14079=CARTESIAN_POINT('Ctrl Pts',(-4.98393512137525,2.82727792454592,6.66133814775094E-16));
#14080=CARTESIAN_POINT('Ctrl Pts',(-5.05163794692084,2.68062955912676,1.34208746866495E-16));
#14081=CARTESIAN_POINT('Ctrl Pts',(-5.11304163000182,2.53144510009992,-1.76889492459881E-15));
#14082=CARTESIAN_POINT('Ctrl Pts',(-5.16794971273575,2.38010471812791,-2.35922392732846E-15));
#14083=CARTESIAN_POINT('Ctrl Pts',(-5.22236412788884,2.23012500723624,-2.94424540016139E-15));
#14084=CARTESIAN_POINT('Ctrl Pts',(-5.27039939637123,2.07802726364688,2.92689554064512E-16));
#14085=CARTESIAN_POINT('Ctrl Pts',(-5.31181481886995,1.92416985016893,-2.16493489801906E-15));
#14086=CARTESIAN_POINT('Ctrl Pts',(-5.32933332980379,1.85908895475255,-3.20449741452864E-15));
#14087=CARTESIAN_POINT('Ctrl Pts',(-5.34566676203086,1.79369312832893,-5.30184591639501E-15));
#14088=CARTESIAN_POINT('Ctrl Pts',(-5.36079407817689,1.72800931712517,-4.9960036108132E-15));
#14089=CARTESIAN_POINT('Ctrl Pts',(-5.39677766745839,1.57176618305015,-4.14671790720287E-15));
#14090=CARTESIAN_POINT('Ctrl Pts',(-5.4259401021884,1.41389282238529,-6.4852137940373E-15));
#14091=CARTESIAN_POINT('Ctrl Pts',(-5.44823692450669,1.25484161090092,-6.10622663543836E-15));
#14092=CARTESIAN_POINT('Ctrl Pts',(-5.46658493932396,1.12395865621973,-5.79435878708482E-15));
#14093=CARTESIAN_POINT('Ctrl Pts',(-5.48028287698849,0.992277986873389,
-5.87332885153964E-15));
#14094=CARTESIAN_POINT('Ctrl Pts',(-5.48928060351323,0.86005942044192,-4.6074255521944E-15));
#14095=CARTESIAN_POINT('Ctrl Pts',(-5.49103894671333,0.83422115823499,-3.71615202053864E-15));
#14096=CARTESIAN_POINT('Ctrl Pts',(-5.49261785043889,0.808358691214049,
-6.19489801465623E-15));
#14097=CARTESIAN_POINT('Ctrl Pts',(-5.49401562173337,0.782500543343462,
-5.99520433297585E-15));
#14098=CARTESIAN_POINT('Ctrl Pts',(-5.50252562943416,0.625069182163987,
-4.45309984798879E-15));
#14099=CARTESIAN_POINT('Ctrl Pts',(-5.50434062410808,0.467610134203912,
-8.25842126848828E-15));
#14100=CARTESIAN_POINT('Ctrl Pts',(-5.49949281171653,0.310550407416323,
-7.38298311375729E-15));
#14101=CARTESIAN_POINT('Ctrl Pts',(-5.49465821572017,0.1539188662209,-5.31715605658429E-15));
#14102=CARTESIAN_POINT('Ctrl Pts',(-5.48319695438002,-0.00231628880926202,
-7.47697400666613E-15));
#14103=CARTESIAN_POINT('Ctrl Pts',(-5.46508984137315,-0.157724420450921,
-6.82787160144471E-15));
#14104=CARTESIAN_POINT('Ctrl Pts',(-5.44729560717373,-0.310447203474091,
-6.19858210290864E-15));
#14105=CARTESIAN_POINT('Ctrl Pts',(-5.42308297461965,-0.462371946136479,
-5.20478416826247E-15));
#14106=CARTESIAN_POINT('Ctrl Pts',(-5.39238722509327,-0.613072707074315,
-4.88498130835069E-15));
#14107=CARTESIAN_POINT('Ctrl Pts',(-5.36573616835424,-0.74391605158746,
-6.47002664417425E-15));
#14108=CARTESIAN_POINT('Ctrl Pts',(-5.33419720831201,-0.873836721881379,
-7.00556211049708E-15));
#14109=CARTESIAN_POINT('Ctrl Pts',(-5.29770061351415,-1.00253949229394,
-5.93969318174459E-15));
#14110=CARTESIAN_POINT('Ctrl Pts',(-5.27375172934145,-1.08699361077776,
-5.19880832617926E-15));
#14111=CARTESIAN_POINT('Ctrl Pts',(-5.24766752212855,-1.17092296801775,
-3.77798944519056E-15));
#14112=CARTESIAN_POINT('Ctrl Pts',(-5.21947367702465,-1.25424893059207,
-2.72004641033163E-15));
#14113=CARTESIAN_POINT('Ctrl Pts',(-5.2123588272694,-1.27527663015708,-3.14869267684114E-15));
#14114=CARTESIAN_POINT('Ctrl Pts',(-5.2051112968655,-1.29626080812995,-1.79997908153132E-15));
#14115=CARTESIAN_POINT('Ctrl Pts',(-5.19773424300509,-1.31719316713618,
-1.83186799063151E-15));
#14116=CARTESIAN_POINT('Ctrl Pts',(-5.1464013431419,-1.4628500525406,-2.22845850964274E-15));
#14117=CARTESIAN_POINT('Ctrl Pts',(-5.08876458161359,-1.60610680701176,
-4.14750974226397E-15));
#14118=CARTESIAN_POINT('Ctrl Pts',(-5.02504407081273,-1.74657685516349,
-4.94049245958195E-15));
#14119=CARTESIAN_POINT('Ctrl Pts',(-4.96146013005027,-1.88674583856183,
-2.94724036326532E-15));
#14120=CARTESIAN_POINT('Ctrl Pts',(-4.89181800426118,-2.0241406789921,1.03279346409245E-15));
#14121=CARTESIAN_POINT('Ctrl Pts',(-4.81629593366406,-2.15834507337917,
2.77555756156289E-16));
#14122=CARTESIAN_POINT('Ctrl Pts',(-4.78797515719014,-2.2086717212743,-8.92932335639387E-16));
#14123=CARTESIAN_POINT('Ctrl Pts',(-4.75882714255844,-2.25854933938649,
1.37195633263433E-15));
#14124=CARTESIAN_POINT('Ctrl Pts',(-4.72886002942117,-2.30795452599388,
1.94289029309402E-15));
#14125=CARTESIAN_POINT('Ctrl Pts',(-4.70988523951568,-2.33923725355665,
2.20939297049903E-15));
#14126=CARTESIAN_POINT('Ctrl Pts',(-4.69058154214804,-2.37033133499752,
4.07705897209819E-15));
#14127=CARTESIAN_POINT('Ctrl Pts',(-4.67095240483681,-2.40122824167162,
2.33146835171283E-15));
#14128=CARTESIAN_POINT('Ctrl Pts',(-4.65361468426418,-2.42851838315778,
7.89650087842628E-16));
#14129=CARTESIAN_POINT('Ctrl Pts',(-4.63602837970922,-2.45564625457261,
1.85008738298638E-15));
#14130=CARTESIAN_POINT('Ctrl Pts',(-4.61820068354681,-2.48260005722413,
1.99840144432528E-15));
#14131=CARTESIAN_POINT('Ctrl Pts',(-4.53479193651534,-2.60870625100355,
2.69230434185812E-15));
#14132=CARTESIAN_POINT('Ctrl Pts',(-4.446064923331,-2.73106380349622,4.08197270232755E-15));
#14133=CARTESIAN_POINT('Ctrl Pts',(-4.3522011455562,-2.84928146336898,3.21964677141295E-15));
#14134=CARTESIAN_POINT('Ctrl Pts',(-4.25980099053161,-2.96565574914612,
2.37076713341881E-15));
#14135=CARTESIAN_POINT('Ctrl Pts',(-4.16242250621293,-3.07801870175783,
-2.96586265836701E-15));
#14136=CARTESIAN_POINT('Ctrl Pts',(-4.06020849653285,-3.18595684819616,
2.55351295663786E-15));
#14137=CARTESIAN_POINT('Ctrl Pts',(-4.03579916371253,-3.21173314000457,
3.87157372706141E-15));
#14138=CARTESIAN_POINT('Ctrl Pts',(-4.01111395005447,-3.23725689213896,
5.18084404389532E-15));
#14139=CARTESIAN_POINT('Ctrl Pts',(-3.98615458747356,-3.26252208283929,
5.77315972805081E-15));
#14140=CARTESIAN_POINT('Ctrl Pts',(-3.95139310944715,-3.29770949471794,
6.56610875245429E-15));
#14141=CARTESIAN_POINT('Ctrl Pts',(-3.91609987445632,-3.33239540188103,
3.68058791726313E-15));
#14142=CARTESIAN_POINT('Ctrl Pts',(-3.88028720092977,-3.36656946842384,
5.55111512312578E-16));
#14143=CARTESIAN_POINT('Origin',(0.,0.,20.));
#14144=CARTESIAN_POINT('',(-12.,-1.46957615897682E-15,20.));
#14145=CARTESIAN_POINT('Origin',(0.,0.,20.));
#14146=CARTESIAN_POINT('Origin',(0.,0.,0.));
#14147=CARTESIAN_POINT('',(-12.,-1.46957615897682E-15,0.));
#14148=CARTESIAN_POINT('',(-12.,-1.46957615897682E-15,0.));
#14149=CARTESIAN_POINT('Origin',(0.,0.,0.));
#14150=CARTESIAN_POINT('Origin',(0.,0.,0.));
#37669=UNCERTAINTY_MEASURE_WITH_UNIT(LENGTH_MEASURE(0.01),#37702,
'DISTANCE_ACCURACY_VALUE',
'Maximum model space distance between geometric entities at asserted c
onnectivities');
#37681=UNCERTAINTY_MEASURE_WITH_UNIT(LENGTH_MEASURE(0.01),#37702,
'DISTANCE_ACCURACY_VALUE',
'Maximum model space distance between geometric entities at asserted c
onnectivities');
#37689=(
GEOMETRIC_REPRESENTATION_CONTEXT(3)
GLOBAL_UNCERTAINTY_ASSIGNED_CONTEXT((#37669))
GLOBAL_UNIT_ASSIGNED_CONTEXT((#37702,#37704,#37705))
REPRESENTATION_CONTEXT('','3D')
);
#37701=(
GEOMETRIC_REPRESENTATION_CONTEXT(3)
GLOBAL_UNCERTAINTY_ASSIGNED_CONTEXT((#37681))
GLOBAL_UNIT_ASSIGNED_CONTEXT((#37702,#37704,#37705))
REPRESENTATION_CONTEXT('','3D')
);
#37702=(
LENGTH_UNIT()
NAMED_UNIT(*)
SI_UNIT(.MILLI.,.METRE.)
);
#37704=(
NAMED_UNIT(*)
PLANE_ANGLE_UNIT()
SI_UNIT($,.RADIAN.)
);
#37705=(
NAMED_UNIT(*)
SI_UNIT($,.STERADIAN.)
SOLID_ANGLE_UNIT()
);
#37713=SHAPE_DEFINITION_REPRESENTATION(#37732,#37785);
#37732=PRODUCT_DEFINITION_SHAPE('',$,#37805);
#37785=SHAPE_REPRESENTATION('',(#4454),#37689);
#37797=PRODUCT_DEFINITION_CONTEXT('part definition',#37856,'design');
#37805=PRODUCT_DEFINITION('Threaded clamp boss','Threaded clamp boss',#37824,
#37797);
#37824=PRODUCT_DEFINITION_FORMATION('',$,#37865);
#37856=APPLICATION_CONTEXT(
'Core Data for Automotive Mechanical Design Process');
#37857=PRODUCT_CONTEXT('part definition',#37856,'mechanical');
#37865=PRODUCT('Threaded clamp boss','Threaded clamp boss',$,(#37857));
#37880=PRESENTATION_STYLE_ASSIGNMENT((#37888));
#37888=SURFACE_STYLE_USAGE(.BOTH.,#37896);
#37896=SURFACE_SIDE_STYLE('',(#37904));
#37904=SURFACE_STYLE_FILL_AREA(#37912);
#37912=FILL_AREA_STYLE('Opaque(185,192,202)',(#37920));
#37920=FILL_AREA_STYLE_COLOUR('Opaque(185,192,202)',#37928);
#37928=COLOUR_RGB('Opaque(185,192,202)',0.725490196078431,0.752941176470588,
0.792156862745098);
ENDSEC;
END-ISO-10303-21;
